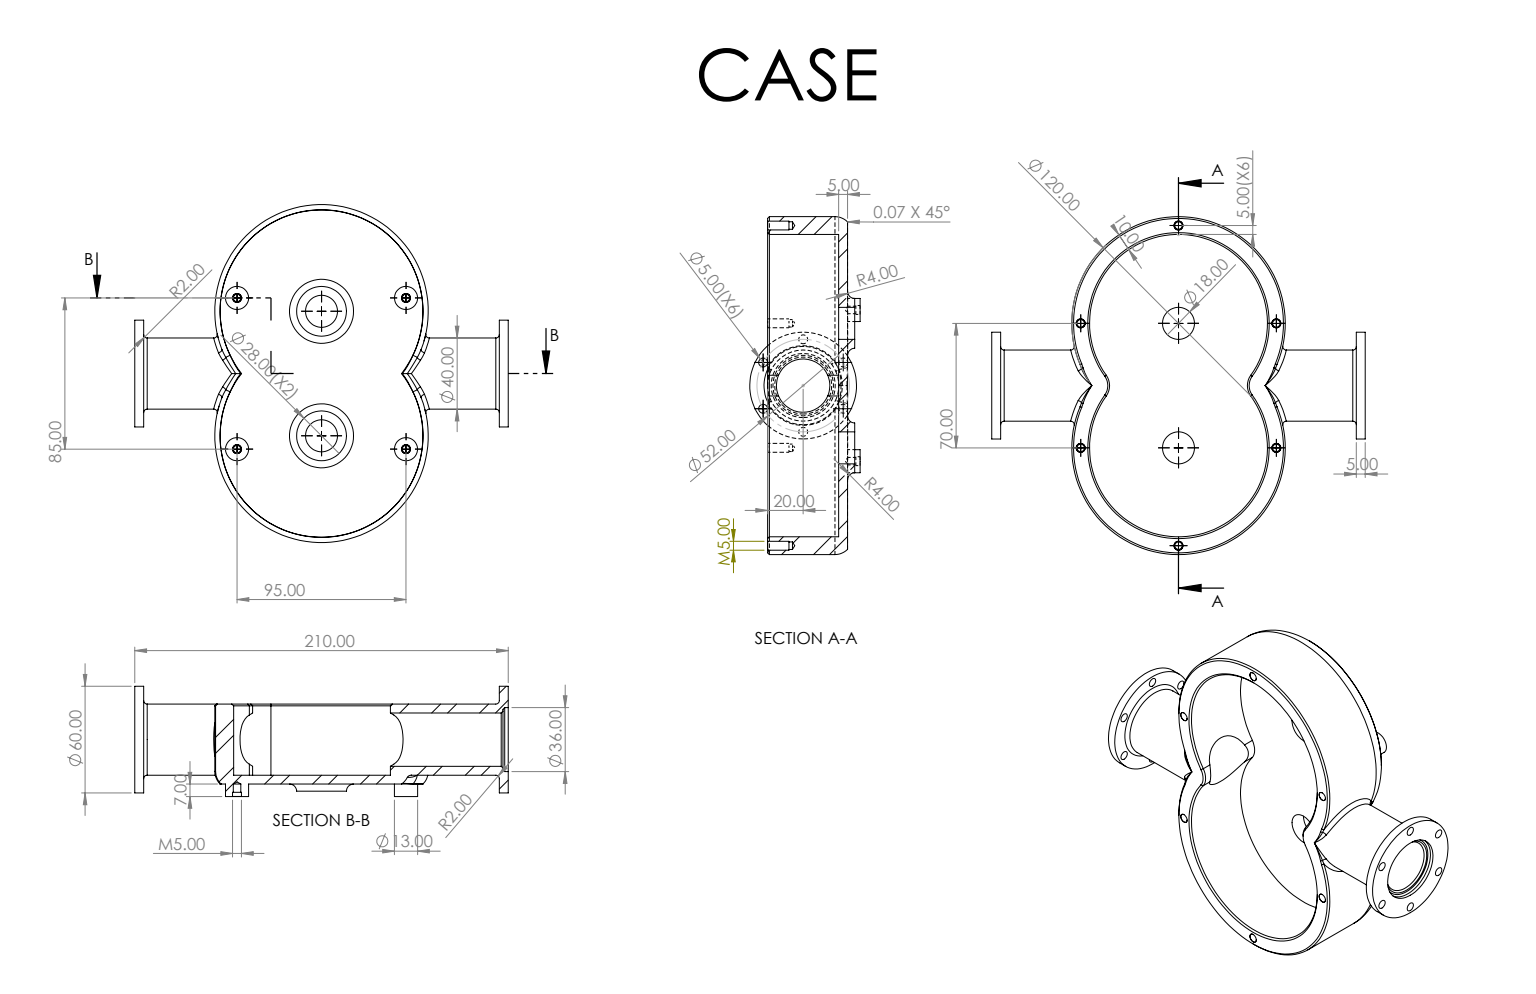
ISO-10303-21;
HEADER;
FILE_DESCRIPTION (('STEP AP214'),
    '1' );
FILE_NAME ('CASE.step',
    '2026-10-24T00:51:42',
    ( '' ),
    ( '' ),
    'SwSTEP 2.0',
    'SolidWorks 2025',
    '' );
FILE_SCHEMA (( 'AUTOMOTIVE_DESIGN' ));
ENDSEC;

DATA;
#6=VECTOR ( 'NONE', #825, 1000.000000000000000 ) ;
#8=LINE ( 'NONE', #12148, #20561 ) ;
#9=CARTESIAN_POINT ( 'NONE',  ( 7.505578006075174891, 1.461761173328240959, -55.63523492904085543 ) ) ;
#15=CARTESIAN_POINT ( 'NONE',  ( -11.08851315719095609, 40.00000000000000000, -54.00022650832062254 ) ) ;
#16=VERTEX_POINT ( 'NONE', #2397 ) ;
#17=DIRECTION ( 'NONE',  ( 0.000000000000000000, -1.000000000000000000, 0.000000000000000000 ) ) ;
#18=CARTESIAN_POINT ( 'NONE',  ( 17.25453130113929134, 34.47978402352274685, -57.33123263757907750 ) ) ;
#21=CARTESIAN_POINT ( 'NONE',  ( 7.552830766296163567, 40.00000000000000000, 52.78252194617787296 ) ) ;
#22=CARTESIAN_POINT ( 'NONE',  ( 14.52224280010135615, 23.83254695043585869, -45.61498238574513664 ) ) ;
#25=CARTESIAN_POINT ( 'NONE',  ( -14.27302218980893578, 2.669631712211265828, 56.31136122552221934 ) ) ;
#26=ADVANCED_FACE ( 'NONE', ( #12912 ), #4119, .F. ) ;
#30=DIRECTION ( 'NONE',  ( -0.000000000000000000, -1.000000000000000000, -0.000000000000000000 ) ) ;
#32=AXIS2_PLACEMENT_3D ( 'NONE', #9463, #19547, #3850 ) ;
#33=ORIENTED_EDGE ( 'NONE', *, *, #2893, .T. ) ;
#37=CARTESIAN_POINT ( 'NONE',  ( 17.68664055422810932, 6.162676607241195370, 57.44855069909474565 ) ) ;
#38=CARTESIAN_POINT ( 'NONE',  ( 9.260192184203184240, 40.00000000000000000, 53.42688922108487759 ) ) ;
#39=EDGE_CURVE ( 'NONE', #4801, #16804, #900, .T. ) ;
#42=CARTESIAN_POINT ( 'NONE',  ( -0.5350771668691333138, 5.000000000000000888, 38.73397172404479960 ) ) ;
#44=CARTESIAN_POINT ( 'NONE',  ( 4.012214033923966740E-15, -1.570715777137759117, 48.07784006879590066 ) ) ;
#46=CARTESIAN_POINT ( 'NONE',  ( -20.00000000000001421, 20.00000000000000000, -60.62177826491068799 ) ) ;
#47=EDGE_LOOP ( 'NONE', ( #21691, #2135, #22378, #2493 ) ) ;
#50=CARTESIAN_POINT ( 'NONE',  ( 35.00000000000000000, -5.000000000000000888, -18.00000000000000000 ) ) ;
#52=CARTESIAN_POINT ( 'NONE',  ( 19.96400288702118431, 18.50890182901837022, 60.61328093326561373 ) ) ;
#54=CARTESIAN_POINT ( 'NONE',  ( -5.833333333333327708, 6.180730040185831164, 40.61164310337068173 ) ) ;
#56=AXIS2_PLACEMENT_3D ( 'NONE', #2091, #11020, #12611 ) ;
#58=ORIENTED_EDGE ( 'NONE', *, *, #10603, .F. ) ;
#59=ORIENTED_EDGE ( 'NONE', *, *, #871, .T. ) ;
#60=DIRECTION ( 'NONE',  ( -0.000000000000000000, -0.000000000000000000, 1.000000000000000000 ) ) ;
#62=ADVANCED_FACE ( 'NONE', ( #18545 ), #20663, .F. ) ;
#63=DIRECTION ( 'NONE',  ( -0.000000000000000000, -1.000000000000000000, -0.000000000000000000 ) ) ;
#65=CARTESIAN_POINT ( 'NONE',  ( 2.244030701350347989, 39.96966515414118959, 50.39883264010746444 ) ) ;
#67=DIRECTION ( 'NONE',  ( -0.000000000000000000, 1.000000000000000000, -0.000000000000000000 ) ) ;
#70=CARTESIAN_POINT ( 'NONE',  ( -34.99999999999999289, 40.00000000000000000, 60.00000000000001421 ) ) ;
#71=ADVANCED_FACE ( 'NONE', ( #20271 ), #22509, .T. ) ;
#76=CARTESIAN_POINT ( 'NONE',  ( -8.123117863918686510, 39.63127865102772063, 53.85467328977310331 ) ) ;
#77=DIRECTION ( 'NONE',  ( 0.000000000000000000, 0.000000000000000000, -1.000000000000000000 ) ) ;
#82=ORIENTED_EDGE ( 'NONE', *, *, #17683, .T. ) ;
#88=DIRECTION ( 'NONE',  ( 0.000000000000000000, 0.000000000000000000, -1.000000000000000000 ) ) ;
#89=DIRECTION ( 'NONE',  ( -0.000000000000000000, 1.000000000000000000, -0.000000000000000000 ) ) ;
#90=CARTESIAN_POINT ( 'NONE',  ( -11.54473802384001324, 36.35512261685148871, -55.24115706042312013 ) ) ;
#91=CARTESIAN_POINT ( 'NONE',  ( -14.50678847729824383, 23.83439465050324912, -45.60743157421818950 ) ) ;
#95=DIRECTION ( 'NONE',  ( 0.7071067811865561215, 8.659560562355038861E-17, -0.7071067811865390240 ) ) ;
#105=VERTEX_POINT ( 'NONE', #9938 ) ;
#108=CYLINDRICAL_SURFACE ( 'NONE', #5479, 2.500000000000002220 ) ;
#110=CARTESIAN_POINT ( 'NONE',  ( 90.00000000000000000, 40.00000000000000000, -2.099999999999991651 ) ) ;
#112=ORIENTED_EDGE ( 'NONE', *, *, #18556, .F. ) ;
#114=CARTESIAN_POINT ( 'NONE',  ( -11.49398617737440986, 39.99999999999999289, 54.13866599136459001 ) ) ;
#117=CIRCLE ( 'NONE', #11814, 20.00000000000000000 ) ;
#118=CARTESIAN_POINT ( 'NONE',  ( 14.34650594848453942, 37.25275621493270961, -56.33443587181653811 ) ) ;
#120=CARTESIAN_POINT ( 'NONE',  ( 14.04383866228953259, 25.28361825225917769, -45.39674436955350245 ) ) ;
#121=VERTEX_POINT ( 'NONE', #15312 ) ;
#123=CARTESIAN_POINT ( 'NONE',  ( -1.321840103127373878, 39.98984252836526565, -49.73540240164955151 ) ) ;
#124=ORIENTED_EDGE ( 'NONE', *, *, #15859, .T. ) ;
#125=DIRECTION ( 'NONE',  ( -0.000000000000000000, -0.000000000000000000, 1.000000000000000000 ) ) ;
#126=VECTOR ( 'NONE', #7524, 1000.000000000000000 ) ;
#130=AXIS2_PLACEMENT_3D ( 'NONE', #19374, #14408, #3677 ) ;
#133=ORIENTED_EDGE ( 'NONE', *, *, #15085, .T. ) ;
#134=ADVANCED_FACE ( 'NONE', ( #4576 ), #8565, .F. ) ;
#136=DIRECTION ( 'NONE',  ( 0.000000000000000000, 0.000000000000000000, -1.000000000000000000 ) ) ;
#139=CARTESIAN_POINT ( 'NONE',  ( 2.175117723777981293, 39.99999999999999289, 50.07592572012215015 ) ) ;
#140=ORIENTED_EDGE ( 'NONE', *, *, #13576, .T. ) ;
#141=FACE_BOUND ( 'NONE', #13024, .T. ) ;
#142=DIRECTION ( 'NONE',  ( 0.000000000000000000, -0.000000000000000000, -1.000000000000000000 ) ) ;
#145=EDGE_CURVE ( 'NONE', #18194, #11720, #10158, .T. ) ;
#149=CARTESIAN_POINT ( 'NONE',  ( -3.591923118226331086E-15, -4.883049072964007919, -45.13706194851761921 ) ) ;
#150=ORIENTED_EDGE ( 'NONE', *, *, #14053, .T. ) ;
#151=CARTESIAN_POINT ( 'NONE',  ( 8.331955809010642255, 38.18181818181816567, 56.36098470834075158 ) ) ;
#152=DIRECTION ( 'NONE',  ( 1.000000000000000000, 0.000000000000000000, 0.000000000000000000 ) ) ;
#153=CARTESIAN_POINT ( 'NONE',  ( -4.436826463219276206, 39.87775421764654027, 51.86208637039475633 ) ) ;
#154=VECTOR ( 'NONE', #7572, 1000.000000000000114 ) ;
#155=CARTESIAN_POINT ( 'NONE',  ( 16.16619463698827630, 31.79081685853978101, 57.00191113791574082 ) ) ;
#158=CONICAL_SURFACE ( 'NONE', #22127, 2.524999999999999467, 0.7853981633973095011 ) ;
#160=AXIS2_PLACEMENT_3D ( 'NONE', #15195, #16931, #6621 ) ;
#164=VERTEX_POINT ( 'NONE', #8227 ) ;
#168=CARTESIAN_POINT ( 'NONE',  ( 0.9607529184257457278, 39.99453553102809877, 49.46704527242837912 ) ) ;
#170=B_SPLINE_CURVE_WITH_KNOTS ( 'NONE', 3,
 ( #22387, #25, #8397, #19283, #7015, #1634, #10434, #3588, #15593, #13972, #6677, #20996, #3128, #5083, #5301, #10546, #17549, #22616, #11941, #17094, #20771, #22497, #10215, #13635, #20652, #12275, #4959, #1859, #17430, #22274, #15253, #20548, #10099, #6572, #8504, #13532, #4852, #11822, #6912, #12059 ),
 .UNSPECIFIED., .F., .F.,
 ( 4, 2, 2, 2, 2, 2, 2, 2, 2, 2, 2, 2, 2, 2, 2, 2, 2, 2, 2, 4 ),
 ( 0.000000000000000000, 0.002766773850155583667, 0.004150160775233378320, 0.005533547700311173406, 0.008300321550466751436, 0.009683708475544540450, 0.01106709540062232947, 0.01660064310093350981, 0.01798403002601129883, 0.01936741695108909131, 0.02213419080124466934, 0.02490096465140025084, 0.02766773850155583581, 0.03043451235171141731, 0.03181789927678920632, 0.03320128620186699187, 0.03873483390217814792, 0.04011822082725592653, 0.04150160775233370514, 0.04426838160248924847 ),
 .UNSPECIFIED. ) ;
#171=EDGE_CURVE ( 'NONE', #14638, #20199, #4931, .T. ) ;
#172=ORIENTED_EDGE ( 'NONE', *, *, #12979, .T. ) ;
#174=CARTESIAN_POINT ( 'NONE',  ( 13.56354382738798847, 2.142135623730931471, -56.03997097393683191 ) ) ;
#176=DIRECTION ( 'NONE',  ( -0.5840452403773153112, 0.8117211080122311850, 0.000000000000000000 ) ) ;
#178=CARTESIAN_POINT ( 'NONE',  ( 11.86180952233169705, 39.00000000000000000, 55.35904751184887118 ) ) ;
#186=EDGE_LOOP ( 'NONE', ( #20186, #1645, #6973, #5901 ) ) ;
#187=AXIS2_PLACEMENT_3D ( 'NONE', #2297, #17991, #16268 ) ;
#191=B_SPLINE_CURVE_WITH_KNOTS ( 'NONE', 3,
 ( #12236, #6868, #6982, #6529, #11779, #5041, #16942, #13938, #20733, #8239, #18781, #17166, #17055, #13836, #5157, #1362 ),
 .UNSPECIFIED., .F., .F.,
 ( 4, 2, 2, 2, 2, 2, 2, 4 ),
 ( 8.673617379884035472E-19, 0.003169695113379691204, 0.006339390226759381540, 0.007924237783449226274, 0.008716661561794153412, 0.009509085340139077080, 0.01109393289682892789, 0.01267878045351877869 ),
 .UNSPECIFIED. ) ;
#193=CARTESIAN_POINT ( 'NONE',  ( 9.367793990832831597, -4.928932186891253231, -51.00106331756588673 ) ) ;
#194=CARTESIAN_POINT ( 'NONE',  ( 11.45074849662552197, 39.99999999999999289, -54.12667998692793958 ) ) ;
#199=VECTOR ( 'NONE', #3023, 1000.000000000000000 ) ;
#200=CARTESIAN_POINT ( 'NONE',  ( -15.91103418227302058, 35.86133518681679533, -56.88632568426858427 ) ) ;
#201=AXIS2_PLACEMENT_3D ( 'NONE', #4772, #15280, #6939 ) ;
#208=ADVANCED_FACE ( 'NONE', ( #17833 ), #17377, .F. ) ;
#213=EDGE_CURVE ( 'NONE', #13383, #4605, #12223, .T. ) ;
#216=VECTOR ( 'NONE', #1494, 1000.000000000000114 ) ;
#219=ORIENTED_EDGE ( 'NONE', *, *, #7330, .T. ) ;
#221=AXIS2_PLACEMENT_3D ( 'NONE', #15560, #3559, #10737 ) ;
#223=ADVANCED_FACE ( 'NONE', ( #21279 ), #5571, .F. ) ;
#226=CARTESIAN_POINT ( 'NONE',  ( -1.387778780781445676E-14, 20.00000000000000000, -105.0020000000000095 ) ) ;
#231=CARTESIAN_POINT ( 'NONE',  ( -9.062586715439731933, 2.130694986425758941, -54.31128890270724696 ) ) ;
#232=ORIENTED_EDGE ( 'NONE', *, *, #1295, .T. ) ;
#234=CARTESIAN_POINT ( 'NONE',  ( 17.14099744770036082, 5.493236686326223861, -57.28126710884282602 ) ) ;
#239=FACE_OUTER_BOUND ( 'NONE', #8251, .T. ) ;
#240=CARTESIAN_POINT ( 'NONE',  ( -7.031141255823502689, 39.67715640622406426, -53.36152254753006474 ) ) ;
#241=AXIS2_PLACEMENT_3D ( 'NONE', #20174, #2191, #19945 ) ;
#244=CARTESIAN_POINT ( 'NONE',  ( -2.496587642955530040, 0.1153990516131219446, 52.32802461649446002 ) ) ;
#245=VECTOR ( 'NONE', #16073, 1000.000000000000000 ) ;
#249=VERTEX_POINT ( 'NONE', #19225 ) ;
#253=LINE ( 'NONE', #3817, #4827 ) ;
#254=DIRECTION ( 'NONE',  ( -0.000000000000000000, -0.000000000000000000, -1.000000000000000000 ) ) ;
#256=CARTESIAN_POINT ( 'NONE',  ( 7.563456360162507330, 39.99999999999999289, 52.78701495172266078 ) ) ;
#259=FACE_BOUND ( 'NONE', #21033, .T. ) ;
#262=CARTESIAN_POINT ( 'NONE',  ( 7.325260514639500961E-15, -4.648749848371387827, 45.43309249825157536 ) ) ;
#264=EDGE_LOOP ( 'NONE', ( #1620, #15292, #18249, #3062 ) ) ;
#268=CARTESIAN_POINT ( 'NONE',  ( -34.99999999999980815, 40.00000000000000711, 52.47499999999922693 ) ) ;
#269=CARTESIAN_POINT ( 'NONE',  ( -0.3104238174410937634, 39.99820335227858692, 49.10409449009599570 ) ) ;
#270=CARTESIAN_POINT ( 'NONE',  ( -35.00000000000000000, 40.00000000000000000, 1.387778780781445676E-14 ) ) ;
#274=CARTESIAN_POINT ( 'NONE',  ( 21.98712579307491666, 15.48449832074051358, 58.57208548029188222 ) ) ;
#276=AXIS2_PLACEMENT_3D ( 'NONE', #12018, #17271, #16939 ) ;
#282=AXIS2_PLACEMENT_3D ( 'NONE', #21094, #12372, #5501 ) ;
#283=ORIENTED_EDGE ( 'NONE', *, *, #5855, .F. ) ;
#284=EDGE_LOOP ( 'NONE', ( #20837, #17843 ) ) ;
#285=CARTESIAN_POINT ( 'NONE',  ( -9.689843208404443686, 39.33333333333332860, 54.54983754392751649 ) ) ;
#289=VECTOR ( 'NONE', #14140, 1000.000000000000000 ) ;
#291=B_SPLINE_CURVE_WITH_KNOTS ( 'NONE', 3,
 ( #8113, #6044, #21633, #5929, #14842, #9709 ),
 .UNSPECIFIED., .F., .F.,
 ( 4, 2, 4 ),
 ( 1.788112030672749005E-18, 0.002694896630591163932, 0.005389793261182326128 ),
 .UNSPECIFIED. ) ;
#293=CARTESIAN_POINT ( 'NONE',  ( 3.944370656192286440, 39.90454853199823759, 51.54919367184183443 ) ) ;
#296=DIRECTION ( 'NONE',  ( 0.000000000000000000, 0.000000000000000000, -1.000000000000000000 ) ) ;
#297=CARTESIAN_POINT ( 'NONE',  ( -42.50000000000000711, -12.00000000000000000, -47.50000000000000000 ) ) ;
#307=DIRECTION ( 'NONE',  ( 1.000000000000000000, 0.000000000000000000, 0.000000000000000000 ) ) ;
#310=ORIENTED_EDGE ( 'NONE', *, *, #5485, .T. ) ;
#311=ADVANCED_FACE ( 'NONE', ( #9013 ), #19696, .F. ) ;
#313=ORIENTED_EDGE ( 'NONE', *, *, #10353, .F. ) ;
#317=FACE_OUTER_BOUND ( 'NONE', #17252, .T. ) ;
#319=DIRECTION ( 'NONE',  ( -0.000000000000000000, 1.000000000000000000, -0.000000000000000000 ) ) ;
#322=CARTESIAN_POINT ( 'NONE',  ( -20.00000000000001421, 19.20373330966867798, 60.62177826491072352 ) ) ;
#325=CARTESIAN_POINT ( 'NONE',  ( -15.00000000000001421, 20.00000000000000000, -45.82575694955838230 ) ) ;
#329=CARTESIAN_POINT ( 'NONE',  ( -1.387778780781445676E-14, 20.00000000000000000, 98.00000000000000000 ) ) ;
#330=DIRECTION ( 'NONE',  ( 0.000000000000000000, 0.000000000000000000, -1.000000000000000000 ) ) ;
#334=FACE_OUTER_BOUND ( 'NONE', #3737, .T. ) ;
#337=DIRECTION ( 'NONE',  ( 0.000000000000000000, -1.000000000000000000, 0.000000000000000000 ) ) ;
#339=( BOUNDED_SURFACE ( )  B_SPLINE_SURFACE ( 3, 2, ( 
 ( #20618, #22011, #20293 ),
 ( #20513, #13386, #1148 ),
 ( #11788, #8141, #20176 ),
 ( #4597, #4928, #11578 ),
 ( #1371, #10065, #17063 ),
 ( #3217, #18567, #8367 ) ),
 .UNSPECIFIED., .F., .F., .F. ) 
 B_SPLINE_SURFACE_WITH_KNOTS ( ( 4, 2, 4 ),
 ( 3, 3 ),
 ( 0.000000000000000000, 0.002858401832365834675, 0.005716803664731669350 ),
 ( 0.000000000000000000, 1.000000000000000000 ),
 .UNSPECIFIED. ) 
 GEOMETRIC_REPRESENTATION_ITEM ( )  RATIONAL_B_SPLINE_SURFACE ( (
 ( 1.000000000000000000, 0.7200096751079140267, 1.000000000000000000),
 ( 1.000000000000000000, 0.7065285139735018038, 1.000000000000000000),
 ( 1.000000000000000000, 0.6920701671002518207, 1.000000000000000000),
 ( 1.000000000000000000, 0.6615687397045608709, 1.000000000000000000),
 ( 1.000000000000000000, 0.6455195629511447653, 1.000000000000000000),
 ( 1.000000000000000000, 0.6290213284793418902, 1.000000000000000000) ) ) 
 REPRESENTATION_ITEM ( '' )  SURFACE ( )  );
#340=ORIENTED_EDGE ( 'NONE', *, *, #16660, .T. ) ;
#341=CARTESIAN_POINT ( 'NONE',  ( 0.2660997432313502165, 39.99958209296121225, -48.93999222993210196 ) ) ;
#343=CARTESIAN_POINT ( 'NONE',  ( -11.68090480754633553, 3.765577839755389622, 57.90797000640144176 ) ) ;
#348=CARTESIAN_POINT ( 'NONE',  ( -6.444993702122386203, 40.00000000000000711, 52.30045897829974422 ) ) ;
#350=DIRECTION ( 'NONE',  ( 0.000000000000000000, 0.000000000000000000, -1.000000000000000000 ) ) ;
#351=CARTESIAN_POINT ( 'NONE',  ( 18.51338123223699483, 7.266791589766445014, -57.69263490290608587 ) ) ;
#355=DIRECTION ( 'NONE',  ( -0.000000000000000000, 1.000000000000000000, -0.000000000000000000 ) ) ;
#356=EDGE_CURVE ( 'NONE', #18097, #20626, #19791, .T. ) ;
#357=EDGE_CURVE ( 'NONE', #922, #13123, #3450, .T. ) ;
#358=CARTESIAN_POINT ( 'NONE',  ( -0.4769535673226554806, 39.99865963977220673, -49.10163031951724122 ) ) ;
#364=EDGE_CURVE ( 'NONE', #16, #13103, #12663, .T. ) ;
#367=EDGE_LOOP ( 'NONE', ( #19878, #14451, #14553, #14113 ) ) ;
#369=B_SPLINE_CURVE_WITH_KNOTS ( 'NONE', 3,
 ( #18817, #9981, #13409, #16973, #17087, #15470 ),
 .UNSPECIFIED., .F., .F.,
 ( 4, 2, 4 ),
 ( 1.978164943978792966E-18, 0.005389490931282729137, 0.01077898186256545654 ),
 .UNSPECIFIED. ) ;
#370=ORIENTED_EDGE ( 'NONE', *, *, #8346, .T. ) ;
#371=CARTESIAN_POINT ( 'NONE',  ( -34.99999999999980815, 39.97500000000000142, 52.49999999999922551 ) ) ;
#373=DIRECTION ( 'NONE',  ( -0.000000000000000000, 1.000000000000000000, -0.000000000000000000 ) ) ;
#374=CARTESIAN_POINT ( 'NONE',  ( 0.3946982817249323205, 39.99999999999999289, 48.99018268902280226 ) ) ;
#380=CARTESIAN_POINT ( 'NONE',  ( -21.21578383525638145, 27.34973130705545685, -58.39578210113618439 ) ) ;
#383=CARTESIAN_POINT ( 'NONE',  ( 0.3709469612214016387, -0.009390992346610399152, 50.78654667931946420 ) ) ;
#385=CARTESIAN_POINT ( 'NONE',  ( 3.981168190751217750, 39.90684668434315086, -51.58237481356633225 ) ) ;
#386=CARTESIAN_POINT ( 'NONE',  ( -3.210361346424068341, 39.75306810546534564, 52.30715206667691319 ) ) ;
#387=CARTESIAN_POINT ( 'NONE',  ( 5.007713804312083461, 0.5950132857128228592, 54.03314628406707243 ) ) ;
#388=ORIENTED_EDGE ( 'NONE', *, *, #9153, .F. ) ;
#389=CARTESIAN_POINT ( 'NONE',  ( 21.77460018174823020, 14.53841458819210786, 58.52494103856225394 ) ) ;
#390=DIRECTION ( 'NONE',  ( -0.000000000000000000, 1.000000000000000000, -0.000000000000000000 ) ) ;
#391=ADVANCED_FACE ( 'NONE', ( #12888 ), #6369, .F. ) ;
#392=AXIS2_PLACEMENT_3D ( 'NONE', #21456, #373, #16290 ) ;
#393=ADVANCED_FACE ( 'NONE', ( #19897 ), #22473, .F. ) ;
#394=FACE_BOUND ( 'NONE', #4049, .T. ) ;
#400=DIRECTION ( 'NONE',  ( 0.000000000000000000, 0.000000000000000000, -1.000000000000000000 ) ) ;
#403=ORIENTED_EDGE ( 'NONE', *, *, #16215, .T. ) ;
#404=CARTESIAN_POINT ( 'NONE',  ( 8.215393105052410050, 1.749144060401382594, 56.08634520685871649 ) ) ;
#408=CARTESIAN_POINT ( 'NONE',  ( 90.00000000000000000, 40.00000000000000000, -9.108981535246192915E-16 ) ) ;
#409=PRODUCT_DEFINITION_CONTEXT ( 'detailed design', #19716, 'design' ) ;
#412=LINE ( 'NONE', #12881, #16434 ) ;
#413=DIRECTION ( 'NONE',  ( -0.000000000000000000, 1.000000000000000000, -0.000000000000000000 ) ) ;
#418=ORIENTED_EDGE ( 'NONE', *, *, #9253, .T. ) ;
#420=ORIENTED_EDGE ( 'NONE', *, *, #17534, .T. ) ;
#423=EDGE_CURVE ( 'NONE', #6835, #14085, #18431, .T. ) ;
#425=CARTESIAN_POINT ( 'NONE',  ( -15.99999999999994493, 20.00000000000000355, 102.0000000000000142 ) ) ;
#431=EDGE_CURVE ( 'NONE', #18746, #22096, #8909, .T. ) ;
#433=CARTESIAN_POINT ( 'NONE',  ( -1.387778780781445518E-14, 20.00000000000000355, 105.0000000000000142 ) ) ;
#434=CARTESIAN_POINT ( 'NONE',  ( -4.240553750831113966, 39.54840718952534218, -53.29860200223215827 ) ) ;
#436=CARTESIAN_POINT ( 'NONE',  ( 42.50000000000000711, -12.00000000000012434, 47.50000000000000711 ) ) ;
#437=EDGE_LOOP ( 'NONE', ( #19321, #11587 ) ) ;
#438=B_SPLINE_CURVE_WITH_KNOTS ( 'NONE', 3,
 ( #10429, #22613, #10094, #4956, #5079, #11935, #22, #18935, #120, #7012, #15588, #17091, #13969, #17204, #1404, #1517, #19051, #3358, #20993, #10316, #17312, #5297, #12272, #19735 ),
 .UNSPECIFIED., .F., .F.,
 ( 4, 2, 2, 2, 2, 2, 2, 2, 2, 2, 2, 4 ),
 ( 0.02614117015034099489, 0.02729036340605310237, 0.02843955666176521332, 0.03073794317318943869, 0.03188713642890154965, 0.03303632968461366060, 0.03533471619603787556, 0.03648390945174998651, 0.03763310270746209746, 0.03993148921888632630, 0.04222987573031054820, 0.04452826224173477704 ),
 .UNSPECIFIED. ) ;
#440=DIRECTION ( 'NONE',  ( 0.000000000000000000, 1.000000000000000000, 0.000000000000000000 ) ) ;
#441=DIRECTION ( 'NONE',  ( 0.000000000000000000, 0.000000000000000000, -1.000000000000000000 ) ) ;
#442=AXIS2_PLACEMENT_3D ( 'NONE', #3968, #12531, #11161 ) ;
#449=CARTESIAN_POINT ( 'NONE',  ( -42.50000000000000711, -9.600000000000001421, -47.50000000000000000 ) ) ;
#451=ORIENTED_EDGE ( 'NONE', *, *, #20783, .T. ) ;
#453=CARTESIAN_POINT ( 'NONE',  ( -9.689843208404424146, 39.33333333333333570, 54.54983754392744544 ) ) ;
#454=VERTEX_POINT ( 'NONE', #9919 ) ;
#464=CARTESIAN_POINT ( 'NONE',  ( -0.8008185833748354687, 39.99628548823710616, -49.34729503705691656 ) ) ;
#465=EDGE_LOOP ( 'NONE', ( #20901, #7728 ) ) ;
#466=FACE_OUTER_BOUND ( 'NONE', #16645, .T. ) ;
#469=EDGE_CURVE ( 'NONE', #19954, #548, #5572, .T. ) ;
#471=VECTOR ( 'NONE', #14248, 1000.000000000000000 ) ;
#477=CIRCLE ( 'NONE', #13626, 2.099999999999997868 ) ;
#478=VERTEX_POINT ( 'NONE', #4882 ) ;
#479=CYLINDRICAL_SURFACE ( 'NONE', #15776, 2.099999999999997868 ) ;
#485=ORIENTED_EDGE ( 'NONE', *, *, #11304, .F. ) ;
#486=CARTESIAN_POINT ( 'NONE',  ( -3.709350152758254637, -1.139907008998718663, 50.71254743501651063 ) ) ;
#487=DIRECTION ( 'NONE',  ( 0.000000000000000000, 1.000000000000000000, 0.000000000000000000 ) ) ;
#488=LINE ( 'NONE', #7485, #991 ) ;
#490=CARTESIAN_POINT ( 'NONE',  ( 2.951378045146772156, -1.204966337759544759, 50.23352299313199154 ) ) ;
#495=ORIENTED_EDGE ( 'NONE', *, *, #11690, .T. ) ;
#496=CARTESIAN_POINT ( 'NONE',  ( 9.433064893952842311, 39.99999999999999289, -53.48670810797406006 ) ) ;
#497=AXIS2_PLACEMENT_3D ( 'NONE', #8009, #16823, #14964 ) ;
#498=CARTESIAN_POINT ( 'NONE',  ( 20.00279574339558053, 20.27588806490328466, 58.14815718762942254 ) ) ;
#499=CARTESIAN_POINT ( 'NONE',  ( -15.49999999999980282, -2.516660498395516310, -105.0000000000000142 ) ) ;
#500=CIRCLE ( 'NONE', #12915, 49.99999999999998579 ) ;
#503=DIRECTION ( 'NONE',  ( 0.000000000000000000, 0.000000000000000000, -1.000000000000000000 ) ) ;
#504=EDGE_CURVE ( 'NONE', #4461, #15820, #3176, .T. ) ;
#506=CIRCLE ( 'NONE', #7080, 2.500000000000002220 ) ;
#507=VERTEX_POINT ( 'NONE', #8099 ) ;
#511=DIRECTION ( 'NONE',  ( 0.000000000000000000, 0.000000000000000000, 1.000000000000000000 ) ) ;
#513=DIRECTION ( 'NONE',  ( 0.000000000000000000, 0.000000000000000000, -1.000000000000000000 ) ) ;
#515=ORIENTED_EDGE ( 'NONE', *, *, #6519, .F. ) ;
#521=EDGE_LOOP ( 'NONE', ( #7198, #21229, #17440, #9818 ) ) ;
#523=CARTESIAN_POINT ( 'NONE',  ( -42.50000000000000711, -5.000000000000000000, -45.40000000000000568 ) ) ;
#524=FACE_OUTER_BOUND ( 'NONE', #18019, .T. ) ;
#529=CARTESIAN_POINT ( 'NONE',  ( 42.50000000000000711, -12.00000000000000000, 47.50000000000000711 ) ) ;
#530=DIRECTION ( 'NONE',  ( 0.000000000000000000, -0.000000000000000000, -1.000000000000000000 ) ) ;
#532=CYLINDRICAL_SURFACE ( 'NONE', #9399, 30.00000000000000000 ) ;
#535=EDGE_LOOP ( 'NONE', ( #8078, #13018, #9083, #19228 ) ) ;
#536=ORIENTED_EDGE ( 'NONE', *, *, #10840, .T. ) ;
#539=CARTESIAN_POINT ( 'NONE',  ( -1.247165098465854882, 0.02902681952929966891, -51.42818515578048277 ) ) ;
#540=EDGE_CURVE ( 'NONE', #20205, #18632, #21256, .T. ) ;
#543=DIRECTION ( 'NONE',  ( 0.000000000000000000, 0.000000000000000000, 1.000000000000000000 ) ) ;
#545=CARTESIAN_POINT ( 'NONE',  ( -10.79594548525845354, 39.62239930148190581, -54.90840750699925366 ) ) ;
#546=FACE_OUTER_BOUND ( 'NONE', #6799, .T. ) ;
#547=DIRECTION ( 'NONE',  ( -0.000000000000000000, 1.000000000000000000, -0.000000000000000000 ) ) ;
#548=VERTEX_POINT ( 'NONE', #54 ) ;
#550=FACE_OUTER_BOUND ( 'NONE', #1337, .T. ) ;
#551=CARTESIAN_POINT ( 'NONE',  ( -1.387778780781445676E-14, 40.00000000000000000, -48.73397172404481381 ) ) ;
#554=CARTESIAN_POINT ( 'NONE',  ( 7.033428926742989695, 6.687309450572964664, -41.47353357286041842 ) ) ;
#555=ORIENTED_EDGE ( 'NONE', *, *, #20018, .F. ) ;
#558=ORIENTED_EDGE ( 'NONE', *, *, #1941, .T. ) ;
#560=CARTESIAN_POINT ( 'NONE',  ( -1.387778780781445676E-14, 20.00000000000000000, -100.0000000000000000 ) ) ;
#563=ORIENTED_EDGE ( 'NONE', *, *, #5695, .F. ) ;
#564=CARTESIAN_POINT ( 'NONE',  ( 14.99999999999998579, 20.00000000000000355, 60.00200000000000244 ) ) ;
#566=DIRECTION ( 'NONE',  ( 0.000000000000000000, 0.000000000000000000, -1.000000000000000000 ) ) ;
#572=DIRECTION ( 'NONE',  ( 0.000000000000000000, 0.000000000000000000, -1.000000000000000000 ) ) ;
#575=VERTEX_POINT ( 'NONE', #17585 ) ;
#576=DIRECTION ( 'NONE',  ( -0.000000000000000000, 1.000000000000000000, -0.000000000000000000 ) ) ;
#578=DIRECTION ( 'NONE',  ( 0.000000000000000000, 0.000000000000000000, 1.000000000000000000 ) ) ;
#579=CARTESIAN_POINT ( 'NONE',  ( -9.064496942927510403, 40.00000000000000711, 53.36141823319849919 ) ) ;
#582=EDGE_LOOP ( 'NONE', ( #20787, #19014, #14328, #6935, #11159 ) ) ;
#585=CARTESIAN_POINT ( 'NONE',  ( -0.6551157041172263051, 39.99751803486232404, -49.23722055247538520 ) ) ;
#588=CARTESIAN_POINT ( 'NONE',  ( -6.261274683082161729, 0.9579800028911584775, 54.84444022978226485 ) ) ;
#590=EDGE_CURVE ( 'NONE', #6177, #19116, #506, .T. ) ;
#592=AXIS2_PLACEMENT_3D ( 'NONE', #3774, #3673, #10624 ) ;
#593=ORIENTED_EDGE ( 'NONE', *, *, #20919, .F. ) ;
#596=EDGE_LOOP ( 'NONE', ( #6630, #2604, #22575, #5586 ) ) ;
#597=ORIENTED_EDGE ( 'NONE', *, *, #20910, .T. ) ;
#599=VERTEX_POINT ( 'NONE', #15846 ) ;
#604=CARTESIAN_POINT ( 'NONE',  ( -26.00000000000001421, 19.99999999999982947, 105.0000000000000142 ) ) ;
#605=CARTESIAN_POINT ( 'NONE',  ( -26.00000000000001421, 19.99999999999982947, -105.0000000000000142 ) ) ;
#606=ORIENTED_EDGE ( 'NONE', *, *, #5866, .F. ) ;
#607=DIRECTION ( 'NONE',  ( 0.000000000000000000, 0.000000000000000000, 1.000000000000000000 ) ) ;
#609=CARTESIAN_POINT ( 'NONE',  ( -42.50000000000000711, -12.00000000000000000, 45.40000000000001279 ) ) ;
#613=CARTESIAN_POINT ( 'NONE',  ( 5.511499161255899004, 0.6970817516857953366, 52.42185088604356480 ) ) ;
#615=CARTESIAN_POINT ( 'NONE',  ( 6.450208405384564081, 39.75599223657528825, 53.02618523645297444 ) ) ;
#617=AXIS2_PLACEMENT_3D ( 'NONE', #4326, #16459, #11301 ) ;
#619=CARTESIAN_POINT ( 'NONE',  ( -1.387778780781445676E-14, 20.00000000000000000, 100.0000000000000000 ) ) ;
#620=CARTESIAN_POINT ( 'NONE',  ( -23.50000000000001066, 19.99999999999982947, 100.0000000000000000 ) ) ;
#623=DIRECTION ( 'NONE',  ( 0.000000000000000000, 0.000000000000000000, -1.000000000000000000 ) ) ;
#629=CARTESIAN_POINT ( 'NONE',  ( -90.00000000000000000, 40.00000000000000000, 2.500000000000001332 ) ) ;
#634=CARTESIAN_POINT ( 'NONE',  ( 90.00000000000000000, 26.00000000000000355, 2.099999999999989875 ) ) ;
#636=B_SPLINE_CURVE_WITH_KNOTS ( 'NONE', 3,
 ( #6378, #17250, #4785, #15175, #18648, #11867, #2952, #18868, #17137, #1455, #1560, #9926, #1216, #22200, #6493, #19858 ),
 .UNSPECIFIED., .F., .F.,
 ( 4, 2, 2, 2, 2, 2, 2, 4 ),
 ( 0.000000000000000000, 0.004782611835060888474, 0.005978264793826106906, 0.007173917752591319266, 0.009565223670121737048, 0.01195652958765215483, 0.01434783550518257435, 0.01913044734024341512 ),
 .UNSPECIFIED. ) ;
#637=EDGE_CURVE ( 'NONE', #15664, #18218, #10005, .T. ) ;
#640=CIRCLE ( 'NONE', #11227, 2.499999999999995115 ) ;
#641=CARTESIAN_POINT ( 'NONE',  ( -42.50000000000000711, -5.000000000000000000, 41.00000000000000711 ) ) ;
#642=CARTESIAN_POINT ( 'NONE',  ( 90.00000000000000000, 26.00000000000000355, -2.099999999999991651 ) ) ;
#646=EDGE_CURVE ( 'NONE', #11081, #11262, #14027, .T. ) ;
#647=DIRECTION ( 'NONE',  ( 0.000000000000000000, 0.000000000000000000, -1.000000000000000000 ) ) ;
#652=AXIS2_PLACEMENT_3D ( 'NONE', #13595, #1481, #11895 ) ;
#653=EDGE_LOOP ( 'NONE', ( #11685, #3181, #17197, #9101 ) ) ;
#654=VECTOR ( 'NONE', #4707, 1000.000000000000000 ) ;
#658=DIRECTION ( 'NONE',  ( 0.000000000000000000, 0.000000000000000000, 1.000000000000000000 ) ) ;
#663=CARTESIAN_POINT ( 'NONE',  ( 6.699391982047661287, -4.821764332415560794, 49.69317737456783846 ) ) ;
#670=DIRECTION ( 'NONE',  ( -1.000000000000000000, 0.000000000000000000, 0.000000000000000000 ) ) ;
#671=DIRECTION ( 'NONE',  ( -0.000000000000000000, -0.000000000000000000, 1.000000000000000000 ) ) ;
#675=VERTEX_POINT ( 'NONE', #8986 ) ;
#677=DIRECTION ( 'NONE',  ( -0.000000000000000000, -0.000000000000000000, -1.000000000000000000 ) ) ;
#678=CARTESIAN_POINT ( 'NONE',  ( -35.00000000000000000, -9.000000000000001776, -17.99999999999998934 ) ) ;
#679=ADVANCED_FACE ( 'NONE', ( #11272 ), #21599, .F. ) ;
#680=EDGE_CURVE ( 'NONE', #9888, #4267, #16975, .T. ) ;
#681=B_SPLINE_CURVE_WITH_KNOTS ( 'NONE', 1,
 ( #16046, #17548 ),
 .UNSPECIFIED., .F., .F.,
 ( 2, 2 ),
 ( 0.000000000000000000, 1.000000000000000000 ),
 .UNSPECIFIED. ) ;
#685=CONICAL_SURFACE ( 'NONE', #20455, 2.099999999999997868, 1.029744258676653867 ) ;
#690=VECTOR ( 'NONE', #4946, 1000.000000000000000 ) ;
#692=CARTESIAN_POINT ( 'NONE',  ( 1.105958719418588032, 39.99272030489618857, -49.57516106150625035 ) ) ;
#695=EDGE_LOOP ( 'NONE', ( #15730, #4327, #172, #15716, #13591, #19027, #8915 ) ) ;
#696=CARTESIAN_POINT ( 'NONE',  ( 42.50000000000000711, -11.97499999999999964, 50.00000000000000711 ) ) ;
#697=CARTESIAN_POINT ( 'NONE',  ( -9.867969867547959240, 0.2954100743916240890, -54.30456930252523051 ) ) ;
#698=EDGE_LOOP ( 'NONE', ( #8656, #15794, #19959, #10887 ) ) ;
#701=CYLINDRICAL_SURFACE ( 'NONE', #14041, 2.500000000000002220 ) ;
#703=ORIENTED_EDGE ( 'NONE', *, *, #22176, .T. ) ;
#707=CARTESIAN_POINT ( 'NONE',  ( -0.09263077948485531898, 39.99995274011368451, -48.80595708259651389 ) ) ;
#709=DIRECTION ( 'NONE',  ( 0.000000000000000000, -0.5150380749100547106, -0.8571673007021120005 ) ) ;
#711=CARTESIAN_POINT ( 'NONE',  ( -13.07600923154787864, 27.35939529837144590, 44.93756990742566870 ) ) ;
#712=DIRECTION ( 'NONE',  ( 0.000000000000000000, 0.000000000000000000, 1.000000000000000000 ) ) ;
#714=ORIENTED_EDGE ( 'NONE', *, *, #18426, .F. ) ;
#715=ORIENTED_EDGE ( 'NONE', *, *, #1941, .F. ) ;
#720=CARTESIAN_POINT ( 'NONE',  ( 19.01465036493455685, 26.21927150370769510, 60.37937655616645571 ) ) ;
#724=CARTESIAN_POINT ( 'NONE',  ( 35.00000000000000000, 0.000000000000000000, -49.99999999999997868 ) ) ;
#725=ORIENTED_EDGE ( 'NONE', *, *, #5057, .T. ) ;
#729=CARTESIAN_POINT ( 'NONE',  ( 34.99999999999980815, 26.00000000000000355, 57.09999999999921982 ) ) ;
#731=CARTESIAN_POINT ( 'NONE',  ( -20.67483659015370989, 11.23071942442636661, -58.26617649125748954 ) ) ;
#733=DIRECTION ( 'NONE',  ( 0.000000000000000000, 0.000000000000000000, -1.000000000000000000 ) ) ;
#736=CARTESIAN_POINT ( 'NONE',  ( 35.00000000000058265, 40.00000000000000000, -57.50000000000076028 ) ) ;
#737=ORIENTED_EDGE ( 'NONE', *, *, #18385, .T. ) ;
#738=CARTESIAN_POINT ( 'NONE',  ( 0.7832247060116511728, 40.00000000000097344, 49.34584201034998330 ) ) ;
#742=CIRCLE ( 'NONE', #8713, 2.499999999999995115 ) ;
#745=ORIENTED_EDGE ( 'NONE', *, *, #22049, .T. ) ;
#747=ORIENTED_EDGE ( 'NONE', *, *, #16037, .F. ) ;
#753=DIRECTION ( 'NONE',  ( 0.000000000000000000, -0.000000000000000000, -1.000000000000000000 ) ) ;
#757=ADVANCED_FACE ( 'NONE', ( #19874, #4184, #394, #12758, #16084, #21830, #9335 ), #6125, .T. ) ;
#759=DIRECTION ( 'NONE',  ( 0.000000000000000000, 1.000000000000000000, 0.000000000000000000 ) ) ;
#761=CYLINDRICAL_SURFACE ( 'NONE', #958, 2.500000000000002220 ) ;
#765=CARTESIAN_POINT ( 'NONE',  ( -1.387778780781445518E-14, 20.00000000000000355, -102.0000000000000142 ) ) ;
#769=ADVANCED_FACE ( 'NONE', ( #14353 ), #18824, .F. ) ;
#770=VECTOR ( 'NONE', #3039, 1000.000000000000114 ) ;
#771=EDGE_LOOP ( 'NONE', ( #13106, #15939, #8345, #9673 ) ) ;
#772=DIRECTION ( 'NONE',  ( -0.000000000000000000, -1.000000000000000000, -0.000000000000000000 ) ) ;
#773=CARTESIAN_POINT ( 'NONE',  ( -18.00000000000001421, 20.00000000000000355, -102.9999999999999716 ) ) ;
#774=CARTESIAN_POINT ( 'NONE',  ( 3.315551171827967991, 0.2472631163744288263, -51.08212483308732743 ) ) ;
#775=EDGE_CURVE ( 'NONE', #15249, #1751, #7841, .T. ) ;
#776=ADVANCED_FACE ( 'NONE', ( #12637 ), #12640, .F. ) ;
#777=EDGE_CURVE ( 'NONE', #10435, #18495, #16621, .T. ) ;
#778=DIRECTION ( 'NONE',  ( 0.000000000000000000, 0.000000000000000000, 1.000000000000000000 ) ) ;
#785=EDGE_CURVE ( 'NONE', #21816, #1314, #14411, .T. ) ;
#786=CARTESIAN_POINT ( 'NONE',  ( -6.401904815323844922, 38.95163572918602313, -55.13655742298576001 ) ) ;
#787=CARTESIAN_POINT ( 'NONE',  ( 28.49999999999998224, 19.99999999999999645, 100.0000000000000000 ) ) ;
#789=EDGE_CURVE ( 'NONE', #1700, #2703, #7118, .T. ) ;
#790=VERTEX_POINT ( 'NONE', #3368 ) ;
#791=ORIENTED_EDGE ( 'NONE', *, *, #16352, .T. ) ;
#792=CARTESIAN_POINT ( 'NONE',  ( 35.00000000000000000, 38.99999999999999289, -59.99999999999999289 ) ) ;
#796=CYLINDRICAL_SURFACE ( 'NONE', #18437, 2.099999999999997868 ) ;
#797=AXIS2_PLACEMENT_3D ( 'NONE', #6808, #136, #18008 ) ;
#798=CARTESIAN_POINT ( 'NONE',  ( 4.846088107612517959, 40.00000000000000000, -51.53252798484124497 ) ) ;
#799=ORIENTED_EDGE ( 'NONE', *, *, #20849, .F. ) ;
#800=CARTESIAN_POINT ( 'NONE',  ( 7.213743607555469950, 39.66007621396295946, -53.46062051868064202 ) ) ;
#806=CARTESIAN_POINT ( 'NONE',  ( -6.910507445196895304, 40.00000000000002132, 52.51112221451682416 ) ) ;
#810=DIRECTION ( 'NONE',  ( 0.000000000000000000, 1.000000000000000000, 0.000000000000000000 ) ) ;
#812=CARTESIAN_POINT ( 'NONE',  ( -0.02199734621860905542, 39.99999719748067406, -48.75108928016371124 ) ) ;
#818=ORIENTED_EDGE ( 'NONE', *, *, #18319, .T. ) ;
#819=ORIENTED_EDGE ( 'NONE', *, *, #12527, .T. ) ;
#821=CARTESIAN_POINT ( 'NONE',  ( 5.748506628226523141, -0.6819283742239256041, 52.01451867725413081 ) ) ;
#823=CIRCLE ( 'NONE', #18392, 22.00000000000000000 ) ;
#825=DIRECTION ( 'NONE',  ( 1.049727191138617217E-16, 0.5150380749100562650, -0.8571673007021111124 ) ) ;
#826=CARTESIAN_POINT ( 'NONE',  ( -34.99999999999980815, 40.00000000000000711, 54.99999999999922551 ) ) ;
#828=CARTESIAN_POINT ( 'NONE',  ( 9.952189117650823036, 40.00000000000000000, 53.64426396172073197 ) ) ;
#831=CARTESIAN_POINT ( 'NONE',  ( -11.13407802442742245, 9.941921282207680122, -43.93745127716449872 ) ) ;
#832=VECTOR ( 'NONE', #9450, 1000.000000000000000 ) ;
#834=CARTESIAN_POINT ( 'NONE',  ( 19.04641992693177244, 13.69305383064222603, -60.38882653684736823 ) ) ;
#839=CARTESIAN_POINT ( 'NONE',  ( 3.630513325115385381, 39.68566305962351493, 51.94955563033850865 ) ) ;
#841=CARTESIAN_POINT ( 'NONE',  ( -6.001999869223751283, -0.8367338791974072709, -52.11627801855959063 ) ) ;
#843=CARTESIAN_POINT ( 'NONE',  ( 11.54473802383823511, 36.35512261685320823, 55.24115706042309881 ) ) ;
#844=DIRECTION ( 'NONE',  ( 0.000000000000000000, 0.000000000000000000, 1.000000000000000000 ) ) ;
#846=DIRECTION ( 'NONE',  ( 0.000000000000000000, -0.000000000000000000, -1.000000000000000000 ) ) ;
#847=AXIS2_PLACEMENT_3D ( 'NONE', #14671, #11121, #712 ) ;
#848=EDGE_CURVE ( 'NONE', #18961, #6724, #20651, .T. ) ;
#850=ORIENTED_EDGE ( 'NONE', *, *, #1184, .T. ) ;
#851=ORIENTED_EDGE ( 'NONE', *, *, #6390, .T. ) ;
#853=CARTESIAN_POINT ( 'NONE',  ( 11.12045539253394821, 39.12082365973188303, 55.06303111140292827 ) ) ;
#856=CARTESIAN_POINT ( 'NONE',  ( -17.00000000000002842, 20.00000000000000355, -102.0000000000000142 ) ) ;
#857=ORIENTED_EDGE ( 'NONE', *, *, #19356, .F. ) ;
#860=ORIENTED_EDGE ( 'NONE', *, *, #4382, .T. ) ;
#861=CIRCLE ( 'NONE', #8544, 2.499999999999995115 ) ;
#862=VERTEX_POINT ( 'NONE', #13878 ) ;
#866=CARTESIAN_POINT ( 'NONE',  ( -0.2719375495013811039, 39.99956352816811034, 48.94448636964621357 ) ) ;
#867=TOROIDAL_SURFACE ( 'NONE', #1956, 50.00000000000000000, 10.00000000000000000 ) ;
#868=VECTOR ( 'NONE', #22657, 1000.000000000000000 ) ;
#869=CARTESIAN_POINT ( 'NONE',  ( -0.7060564148929356909, 40.00000000000297007, 49.41654780795607849 ) ) ;
#871=EDGE_CURVE ( 'NONE', #15231, #21079, #14775, .T. ) ;
#874=ORIENTED_EDGE ( 'NONE', *, *, #14173, .F. ) ;
#876=VECTOR ( 'NONE', #4480, 1000.000000000000000 ) ;
#878=CARTESIAN_POINT ( 'NONE',  ( -19.80158170751280977, 22.94611027470400089, 60.57464962002575959 ) ) ;
#879=ADVANCED_FACE ( 'NONE', ( #8621, #20896 ), #5197, .F. ) ;
#882=CARTESIAN_POINT ( 'NONE',  ( -0.3446551741029754701, -0.009348518860373671718, -50.24945914274646697 ) ) ;
#884=AXIS2_PLACEMENT_3D ( 'NONE', #22625, #19477, #2053 ) ;
#887=CARTESIAN_POINT ( 'NONE',  ( -4.628075497661881421, 39.46063506869896997, -53.65703709786517805 ) ) ;
#889=CARTESIAN_POINT ( 'NONE',  ( 35.00000000000058265, 40.00000000000000000, -52.90000000000076597 ) ) ;
#891=PRODUCT ( 'CASE', 'CASE', '', ( #13512 ) ) ;
#894=EDGE_LOOP ( 'NONE', ( #6024, #21589, #6688, #10460 ) ) ;
#895=DIRECTION ( 'NONE',  ( 0.000000000000000000, 0.000000000000000000, -1.000000000000000000 ) ) ;
#897=DIRECTION ( 'NONE',  ( 0.000000000000000000, 0.7071067811866457165, 0.7071067811864494290 ) ) ;
#900=LINE ( 'NONE', #4353, #17009 ) ;
#903=EDGE_CURVE ( 'NONE', #13935, #5360, #8572, .T. ) ;
#906=ORIENTED_EDGE ( 'NONE', *, *, #22508, .T. ) ;
#911=CARTESIAN_POINT ( 'NONE',  ( 0.5525046371098545350, 39.99819307499277699, -49.15917675262092246 ) ) ;
#914=ADVANCED_FACE ( 'NONE', ( #16533 ), #19558, .F. ) ;
#915=DIRECTION ( 'NONE',  ( -0.000000000000000000, 1.000000000000000000, -0.000000000000000000 ) ) ;
#917=CARTESIAN_POINT ( 'NONE',  ( -15.97698236194133159, 7.938033795522204450, -59.50430813415450615 ) ) ;
#922=VERTEX_POINT ( 'NONE', #11605 ) ;
#923=CARTESIAN_POINT ( 'NONE',  ( 35.00000000000058265, 26.00000000000000355, -55.00000000000076028 ) ) ;
#926=DIRECTION ( 'NONE',  ( -0.000000000000000000, -1.000000000000000000, -0.000000000000000000 ) ) ;
#927=CIRCLE ( 'NONE', #18856, 2.099999999999997868 ) ;
#929=CARTESIAN_POINT ( 'NONE',  ( -14.76055860720890500, 22.69766935715934153, 45.72055682016589628 ) ) ;
#932=ORIENTED_EDGE ( 'NONE', *, *, #1320, .T. ) ;
#933=EDGE_CURVE ( 'NONE', #11968, #13427, #9674, .T. ) ;
#935=B_SPLINE_CURVE_WITH_KNOTS ( 'NONE', 3,
 ( #21269, #3747, #5561, #17826, #19447, #174 ),
 .UNSPECIFIED., .F., .F.,
 ( 4, 2, 4 ),
 ( 1.991993874847888106E-18, 0.002694896630591175207, 0.005389793261182347812 ),
 .UNSPECIFIED. ) ;
#938=VERTEX_POINT ( 'NONE', #20206 ) ;
#939=CARTESIAN_POINT ( 'NONE',  ( 16.16780438139466014, 31.78273399965604540, 59.56292242448185448 ) ) ;
#947=CARTESIAN_POINT ( 'NONE',  ( -14.17374118098246605, 15.07546459525165261, -45.45638825402599537 ) ) ;
#949=CARTESIAN_POINT ( 'NONE',  ( 16.97539716422056699, 9.395639044392945394, -59.81372721910505419 ) ) ;
#951=CARTESIAN_POINT ( 'NONE',  ( -3.179547497537916545, 39.99999999999999289, -50.65098726527259743 ) ) ;
#952=CARTESIAN_POINT ( 'NONE',  ( 0.3104238174410367535, 39.99820335227857271, -49.10409449009593175 ) ) ;
#954=CARTESIAN_POINT ( 'NONE',  ( -18.00000000000001421, 20.00000000000000711, 103.0000000000000284 ) ) ;
#957=AXIS2_PLACEMENT_3D ( 'NONE', #1200, #4989, #11969 ) ;
#958=AXIS2_PLACEMENT_3D ( 'NONE', #6027, #9689, #16676 ) ;
#964=CARTESIAN_POINT ( 'NONE',  ( 19.96647043697146984, 18.54527240924682729, -60.61386395554088580 ) ) ;
#966=ADVANCED_FACE ( 'NONE', ( #6228 ), #11858, .F. ) ;
#967=EDGE_LOOP ( 'NONE', ( #20857, #1137, #9405, #12556 ) ) ;
#971=CIRCLE ( 'NONE', #22574, 2.499999999999996891 ) ;
#973=CARTESIAN_POINT ( 'NONE',  ( 10.81645871535806336, 39.16817317914274810, 54.94897387137724110 ) ) ;
#976=ORIENTED_EDGE ( 'NONE', *, *, #16314, .T. ) ;
#979=ORIENTED_EDGE ( 'NONE', *, *, #10273, .F. ) ;
#981=AXIS2_PLACEMENT_3D ( 'NONE', #21390, #5359, #15768 ) ;
#983=CARTESIAN_POINT ( 'NONE',  ( -1.485717122675833668, -1.299971956346735791, -49.29290837556842320 ) ) ;
#987=ADVANCED_FACE ( 'NONE', ( #11375 ), #158, .F. ) ;
#990=EDGE_LOOP ( 'NONE', ( #5095, #11437, #19565, #9961 ) ) ;
#991=VECTOR ( 'NONE', #14455, 1000.000000000000000 ) ;
#992=ORIENTED_EDGE ( 'NONE', *, *, #14848, .T. ) ;
#994=CARTESIAN_POINT ( 'NONE',  ( -20.65262896361484835, 28.82759387226903769, 58.26038807538093778 ) ) ;
#996=AXIS2_PLACEMENT_3D ( 'NONE', #6782, #6667, #13523 ) ;
#998=CARTESIAN_POINT ( 'NONE',  ( -11.45074849662542782, 39.99999999999999289, 54.12667998692793958 ) ) ;
#999=DIRECTION ( 'NONE',  ( 0.000000000000000000, 0.000000000000000000, 1.000000000000000000 ) ) ;
#1000=CARTESIAN_POINT ( 'NONE',  ( -90.00000000000000000, 40.00000000000000711, -2.525000000000000355 ) ) ;
#1001=CARTESIAN_POINT ( 'NONE',  ( 3.210598435713497345, 39.75302854575188150, 52.30739040051271616 ) ) ;
#1003=CARTESIAN_POINT ( 'NONE',  ( -2.568452277497750937E-14, 40.00000000000000000, -48.73397172404482092 ) ) ;
#1004=ADVANCED_FACE ( 'NONE', ( #2680 ), #15298, .T. ) ;
#1005=EDGE_LOOP ( 'NONE', ( #5740, #22368, #2661, #14334 ) ) ;
#1007=AXIS2_PLACEMENT_3D ( 'NONE', #13919, #17486, #21158 ) ;
#1014=AXIS2_PLACEMENT_3D ( 'NONE', #14105, #8524, #15499 ) ;
#1016=CARTESIAN_POINT ( 'NONE',  ( -42.50000000000000711, -11.97499999999999964, -45.00000000000000000 ) ) ;
#1018=AXIS2_PLACEMENT_3D ( 'NONE', #22227, #12123, #15545 ) ;
#1021=AXIS2_PLACEMENT_3D ( 'NONE', #20944, #11063, #530 ) ;
#1023=ORIENTED_EDGE ( 'NONE', *, *, #11379, .T. ) ;
#1024=CARTESIAN_POINT ( 'NONE',  ( 3.072145818613496449, 39.94358020626381744, -50.97359800879427638 ) ) ;
#1026=CIRCLE ( 'NONE', #652, 2.500000000000002220 ) ;
#1030=CARTESIAN_POINT ( 'NONE',  ( -5.004759427256008308, 40.00000000000000000, 51.61237555825404399 ) ) ;
#1031=ADVANCED_FACE ( 'NONE', ( #10212 ), #3584, .T. ) ;
#1033=AXIS2_PLACEMENT_3D ( 'NONE', #8268, #15697, #15237 ) ;
#1036=EDGE_LOOP ( 'NONE', ( #13313, #7843, #1348, #16196 ) ) ;
#1037=CARTESIAN_POINT ( 'NONE',  ( 14.04383866228953792, 25.28361825225916704, 45.39674436955350956 ) ) ;
#1040=CARTESIAN_POINT ( 'NONE',  ( 12.99999999999993960, 42.51666049839543149, 60.00099999999999767 ) ) ;
#1042=DIRECTION ( 'NONE',  ( -0.000000000000000000, -0.000000000000000000, -1.000000000000000000 ) ) ;
#1045=CARTESIAN_POINT ( 'NONE',  ( -14.05436202270911217, 25.29714423467776996, 45.40204559108968141 ) ) ;
#1049=CIRCLE ( 'NONE', #8360, 2.499999999999998668 ) ;
#1055=CARTESIAN_POINT ( 'NONE',  ( 14.31751149541521784, 33.97259629115305302, -58.93694582298954998 ) ) ;
#1058=CARTESIAN_POINT ( 'NONE',  ( -34.99999999999999289, 0.000000000000000000, 50.00000000000000000 ) ) ;
#1059=VECTOR ( 'NONE', #10373, 1000.000000000000000 ) ;
#1067=EDGE_CURVE ( 'NONE', #17407, #7645, #438, .T. ) ;
#1070=LINE ( 'NONE', #609, #17776 ) ;
#1074=CARTESIAN_POINT ( 'NONE',  ( -5.234365469061698306, 40.00000000000000711, -51.72901482534432205 ) ) ;
#1075=CARTESIAN_POINT ( 'NONE',  ( 8.331955809010596070, 38.18181818181818699, -56.36098470834070895 ) ) ;
#1077=CARTESIAN_POINT ( 'NONE',  ( 9.375581681113587251, 39.53990230686088836, 54.37755644423855017 ) ) ;
#1078=FACE_OUTER_BOUND ( 'NONE', #20598, .T. ) ;
#1079=CARTESIAN_POINT ( 'NONE',  ( -2.951413581184478829, -1.204958657596112870, -50.23354289400218420 ) ) ;
#1083=CARTESIAN_POINT ( 'NONE',  ( -15.00000000000001421, 20.00000000000000000, -101.0000000000000284 ) ) ;
#1084=CARTESIAN_POINT ( 'NONE',  ( 19.64963058618602787, 23.83053889023033634, -60.53829769526750937 ) ) ;
#1085=AXIS2_PLACEMENT_3D ( 'NONE', #4347, #671, #12905 ) ;
#1090=CARTESIAN_POINT ( 'NONE',  ( 11.25639079644659724, 39.09917355294047780, 55.11545576760340026 ) ) ;
#1092=ORIENTED_EDGE ( 'NONE', *, *, #11379, .F. ) ;
#1097=CARTESIAN_POINT ( 'NONE',  ( 12.09218358684717920, 1.291952833853752924, 55.42846997241154838 ) ) ;
#1098=AXIS2_PLACEMENT_3D ( 'NONE', #16217, #413, #16338 ) ;
#1100=DIRECTION ( 'NONE',  ( 0.000000000000000000, 0.000000000000000000, 1.000000000000000000 ) ) ;
#1101=DIRECTION ( 'NONE',  ( -0.000000000000000000, -1.000000000000000000, -0.000000000000000000 ) ) ;
#1102=CARTESIAN_POINT ( 'NONE',  ( -18.50805780747144880, 27.59542556733953944, -60.24679276096814817 ) ) ;
#1104=EDGE_CURVE ( 'NONE', #14723, #11771, #19837, .T. ) ;
#1106=CARTESIAN_POINT ( 'NONE',  ( 10.30713387248687773, 2.842164160680653584, -57.27491564205610786 ) ) ;
#1107=ADVANCED_FACE ( 'NONE', ( #21321 ), #701, .F. ) ;
#1111=ORIENTED_EDGE ( 'NONE', *, *, #17841, .F. ) ;
#1112=CARTESIAN_POINT ( 'NONE',  ( -19.96647043697144852, 18.54527240924516818, 60.61386395554428219 ) ) ;
#1113=DIRECTION ( 'NONE',  ( -1.000000000000000000, 0.000000000000000000, 0.000000000000000000 ) ) ;
#1115=CARTESIAN_POINT ( 'NONE',  ( -11.28246622563948520, 40.00000000000000711, 54.06713842414183802 ) ) ;
#1117=ORIENTED_EDGE ( 'NONE', *, *, #4115, .T. ) ;
#1119=CARTESIAN_POINT ( 'NONE',  ( -34.99999999999980815, 40.00000000000000000, 54.99999999999922551 ) ) ;
#1121=CARTESIAN_POINT ( 'NONE',  ( -5.133444049470117676, 39.34078687931064167, -53.02546735988109816 ) ) ;
#1122=DIRECTION ( 'NONE',  ( 0.000000000000000000, 0.000000000000000000, 1.000000000000000000 ) ) ;
#1123=ORIENTED_EDGE ( 'NONE', *, *, #11097, .F. ) ;
#1126=DIRECTION ( 'NONE',  ( 0.000000000000000000, -0.000000000000000000, -1.000000000000000000 ) ) ;
#1132=AXIS2_PLACEMENT_3D ( 'NONE', #8155, #6437, #14895 ) ;
#1135=CARTESIAN_POINT ( 'NONE',  ( -4.044995508448087307, -4.680814751541408469, 48.25214090642531772 ) ) ;
#1136=DIRECTION ( 'NONE',  ( -0.000000000000000000, -1.000000000000000000, -0.000000000000000000 ) ) ;
#1137=ORIENTED_EDGE ( 'NONE', *, *, #19566, .F. ) ;
#1142=CARTESIAN_POINT ( 'NONE',  ( 10.77132920883424205, 39.17511451497404806, -54.93228420922696387 ) ) ;
#1143=FACE_OUTER_BOUND ( 'NONE', #9305, .T. ) ;
#1147=CARTESIAN_POINT ( 'NONE',  ( 6.041077103367500811, -0.8288449397161629095, 52.13906252460464685 ) ) ;
#1148=CARTESIAN_POINT ( 'NONE',  ( 8.219889501001356180, 1.750964516533152437, -56.08920281153656617 ) ) ;
#1149=CARTESIAN_POINT ( 'NONE',  ( -1.387778780781445676E-14, 40.00000000000000000, -48.73397172404481381 ) ) ;
#1150=VERTEX_POINT ( 'NONE', #19494 ) ;
#1151=EDGE_CURVE ( 'NONE', #1471, #10193, #15429, .T. ) ;
#1155=EDGE_CURVE ( 'NONE', #18643, #19011, #9589, .T. ) ;
#1159=CARTESIAN_POINT ( 'NONE',  ( 19.41351212956690730, 24.83257706694782030, -60.47995209899215041 ) ) ;
#1161=CARTESIAN_POINT ( 'NONE',  ( 5.833333333333336590, 39.00000000000000711, 40.61164310337068173 ) ) ;
#1162=DIRECTION ( 'NONE',  ( 1.000000000000000000, 0.000000000000000000, 0.000000000000000000 ) ) ;
#1163=DIRECTION ( 'NONE',  ( 0.000000000000000000, 0.000000000000000000, 1.000000000000000000 ) ) ;
#1164=CARTESIAN_POINT ( 'NONE',  ( 0.5279010140432808251, 4.999719073153301885, -38.73355033370100386 ) ) ;
#1166=DIRECTION ( 'NONE',  ( -1.000000000000000000, 0.000000000000000000, 0.000000000000000000 ) ) ;
#1168=ORIENTED_EDGE ( 'NONE', *, *, #20660, .T. ) ;
#1171=LINE ( 'NONE', #6331, #5023 ) ;
#1174=CARTESIAN_POINT ( 'NONE',  ( -1.387778780781445676E-14, 40.00000000000000000, -48.73397172404481381 ) ) ;
#1175=ORIENTED_EDGE ( 'NONE', *, *, #2779, .F. ) ;
#1176=LINE ( 'NONE', #13633, #12302 ) ;
#1177=EDGE_LOOP ( 'NONE', ( #4533, #4568 ) ) ;
#1181=DIRECTION ( 'NONE',  ( -0.000000000000000000, -0.000000000000000000, 1.000000000000000000 ) ) ;
#1182=CARTESIAN_POINT ( 'NONE',  ( 17.96966555604127791, 28.82469637350566671, -60.10139901455266198 ) ) ;
#1184=EDGE_CURVE ( 'NONE', #18333, #16148, #3013, .T. ) ;
#1185=ORIENTED_EDGE ( 'NONE', *, *, #5813, .F. ) ;
#1186=AXIS2_PLACEMENT_3D ( 'NONE', #12099, #19093, #17360 ) ;
#1187=VERTEX_POINT ( 'NONE', #10645 ) ;
#1188=EDGE_LOOP ( 'NONE', ( #4686, #20113, #19205, #17754, #20799, #14313 ) ) ;
#1190=CARTESIAN_POINT ( 'NONE',  ( 10.87562399044275274, 39.15903841214502279, 54.97094722865957550 ) ) ;
#1193=ORIENTED_EDGE ( 'NONE', *, *, #10418, .F. ) ;
#1195=CARTESIAN_POINT ( 'NONE',  ( -4.842578813368415780, -0.8535550256952800785, -51.47191290771856131 ) ) ;
#1197=DIRECTION ( 'NONE',  ( 0.000000000000000000, 0.000000000000000000, 1.000000000000000000 ) ) ;
#1198=CARTESIAN_POINT ( 'NONE',  ( 9.857944917837743404, 0.2919354798308393395, 54.29891737064654222 ) ) ;
#1200=CARTESIAN_POINT ( 'NONE',  ( 35.00000000000058265, 40.00000000000000000, -55.00000000000076028 ) ) ;
#1202=DIRECTION ( 'NONE',  ( 0.000000000000000000, 0.000000000000000000, -1.000000000000000000 ) ) ;
#1203=DIRECTION ( 'NONE',  ( -0.000000000000000000, -0.000000000000000000, -1.000000000000000000 ) ) ;
#1204=CARTESIAN_POINT ( 'NONE',  ( -12.24033418603700873, 35.84417766536505923, -58.14550894043696161 ) ) ;
#1205=AXIS2_PLACEMENT_3D ( 'NONE', #2980, #20505, #19016 ) ;
#1207=CARTESIAN_POINT ( 'NONE',  ( -14.92530643917655375, 18.45549920837825653, 45.79309713780078539 ) ) ;
#1209=ORIENTED_EDGE ( 'NONE', *, *, #1765, .F. ) ;
#1210=ADVANCED_FACE ( 'NONE', ( #5858 ), #7792, .F. ) ;
#1212=CARTESIAN_POINT ( 'NONE',  ( -18.15458487487865114, 6.756534690977250790, 57.58998093367232940 ) ) ;
#1216=CARTESIAN_POINT ( 'NONE',  ( -19.23800698326016700, 14.47374112874266316, -60.43633296823762890 ) ) ;
#1217=CARTESIAN_POINT ( 'NONE',  ( 9.075375594263590528, 39.43595020987488198, 54.33405310157220924 ) ) ;
#1218=AXIS2_PLACEMENT_3D ( 'NONE', #16052, #4046, #11014 ) ;
#1222=CARTESIAN_POINT ( 'NONE',  ( -13.00000000000011546, 42.51666049839536043, 105.0000000000000142 ) ) ;
#1225=ORIENTED_EDGE ( 'NONE', *, *, #15054, .T. ) ;
#1226=AXIS2_PLACEMENT_3D ( 'NONE', #17024, #22324, #13460 ) ;
#1227=CARTESIAN_POINT ( 'NONE',  ( -10.07716038413160220, 39.27871711242732289, 54.68297691402418792 ) ) ;
#1228=FACE_OUTER_BOUND ( 'NONE', #10168, .T. ) ;
#1232=CARTESIAN_POINT ( 'NONE',  ( -34.99999999999980815, 40.00000000000000000, 54.99999999999922551 ) ) ;
#1233=FACE_BOUND ( 'NONE', #5891, .T. ) ;
#1234=AXIS2_PLACEMENT_3D ( 'NONE', #18228, #14666, #5966 ) ;
#1239=CARTESIAN_POINT ( 'NONE',  ( -34.99999999999980815, 40.00000000000000711, 54.99999999999922551 ) ) ;
#1240=AXIS2_PLACEMENT_3D ( 'NONE', #16313, #6008, #623 ) ;
#1245=EDGE_CURVE ( 'NONE', #4801, #14603, #15791, .T. ) ;
#1246=FACE_OUTER_BOUND ( 'NONE', #2056, .T. ) ;
#1248=CARTESIAN_POINT ( 'NONE',  ( -19.67353980729183860, 23.69994786803828646, -58.06093965453396066 ) ) ;
#1249=AXIS2_PLACEMENT_3D ( 'NONE', #16047, #355, #4140 ) ;
#1250=CARTESIAN_POINT ( 'NONE',  ( -8.115799706357579524, 39.55796121550449129, 53.89994064586117872 ) ) ;
#1253=CARTESIAN_POINT ( 'NONE',  ( 11.13407802442741357, 30.05807871779230922, 43.93745127716450583 ) ) ;
#1257=DIRECTION ( 'NONE',  ( 0.000000000000000000, 0.000000000000000000, -1.000000000000000000 ) ) ;
#1258=EDGE_CURVE ( 'NONE', #19899, #11765, #2874, .T. ) ;
#1268=SHAPE_DEFINITION_REPRESENTATION ( #11514, #21292 ) ;
#1269=B_SPLINE_CURVE_WITH_KNOTS ( 'NONE', 3,
 ( #20292, #4596, #1147, #15100, #20405, #4714 ),
 .UNSPECIFIED., .F., .F.,
 ( 4, 2, 4 ),
 ( 1.116583492552567205E-17, 0.005389490931280165216, 0.01077898186256031829 ),
 .UNSPECIFIED. ) ;
#1270=EDGE_LOOP ( 'NONE', ( #4084, #14632, #16343, #5836 ) ) ;
#1274=CARTESIAN_POINT ( 'NONE',  ( 34.99999999999980815, 40.00000000000000711, 54.99999999999922551 ) ) ;
#1279=LINE ( 'NONE', #2904, #17100 ) ;
#1282=FACE_BOUND ( 'NONE', #19366, .T. ) ;
#1285=CARTESIAN_POINT ( 'NONE',  ( 8.847970474273168406, 40.00000000000000711, 53.28481329029794011 ) ) ;
#1286=VERTEX_POINT ( 'NONE', #20172 ) ;
#1287=CARTESIAN_POINT ( 'NONE',  ( -8.197131438766653844, 40.00000000000000711, -53.04141935927233931 ) ) ;
#1289=DIRECTION ( 'NONE',  ( -0.000000000000000000, -0.000000000000000000, 1.000000000000000000 ) ) ;
#1290=CARTESIAN_POINT ( 'NONE',  ( -6.626710883749606351E-15, -0.4099546584827634121, -48.99240008041271466 ) ) ;
#1294=DIRECTION ( 'NONE',  ( -1.000000000000000000, 0.000000000000000000, 0.000000000000000000 ) ) ;
#1295=EDGE_CURVE ( 'NONE', #11321, #18787, #22415, .T. ) ;
#1296=CARTESIAN_POINT ( 'NONE',  ( 21.83670385715308271, 14.52494903933254911, -58.53909266577284143 ) ) ;
#1298=CIRCLE ( 'NONE', #18126, 2.099999999999997868 ) ;
#1299=ORIENTED_EDGE ( 'NONE', *, *, #14707, .F. ) ;
#1300=ORIENTED_EDGE ( 'NONE', *, *, #1610, .F. ) ;
#1301=PLANE ( 'NONE',  #6546 ) ;
#1305=EDGE_CURVE ( 'NONE', #5648, #21174, #12867, .T. ) ;
#1308=CARTESIAN_POINT ( 'NONE',  ( -6.661198439252719261, -4.819795714544886422, -49.67388352366067750 ) ) ;
#1312=CIRCLE ( 'NONE', #2406, 2.500000000000002220 ) ;
#1314=VERTEX_POINT ( 'NONE', #11574 ) ;
#1315=CARTESIAN_POINT ( 'NONE',  ( 5.204790488456048969, 39.83796511861606859, -52.32473449166996460 ) ) ;
#1316=AXIS2_PLACEMENT_3D ( 'NONE', #12247, #4233, #13025 ) ;
#1320=EDGE_CURVE ( 'NONE', #19781, #3437, #5567, .T. ) ;
#1323=CARTESIAN_POINT ( 'NONE',  ( -9.855264211176372413, 8.670295722316108566, 43.22210574525161064 ) ) ;
#1327=ORIENTED_EDGE ( 'NONE', *, *, #3809, .T. ) ;
#1329=ORIENTED_EDGE ( 'NONE', *, *, #637, .T. ) ;
#1330=CARTESIAN_POINT ( 'NONE',  ( -22.43750227530606978, 20.33721733311116253, 58.67013217117688839 ) ) ;
#1335=CARTESIAN_POINT ( 'NONE',  ( -11.16030968682941804, 40.00000000000000000, 54.02479386262969996 ) ) ;
#1337=EDGE_LOOP ( 'NONE', ( #4788, #4078 ) ) ;
#1339=CARTESIAN_POINT ( 'NONE',  ( -6.019227127673981492, 39.99999999999999289, -52.10376796897383400 ) ) ;
#1340=EDGE_CURVE ( 'NONE', #7376, #22334, #6534, .T. ) ;
#1346=DIRECTION ( 'NONE',  ( -0.000000000000000000, -1.000000000000000000, -0.000000000000000000 ) ) ;
#1348=ORIENTED_EDGE ( 'NONE', *, *, #7352, .T. ) ;
#1350=DIRECTION ( 'NONE',  ( 0.000000000000000000, 0.000000000000000000, -1.000000000000000000 ) ) ;
#1352=DIRECTION ( 'NONE',  ( 0.000000000000000000, 0.000000000000000000, -1.000000000000000000 ) ) ;
#1358=DIRECTION ( 'NONE',  ( -0.000000000000000000, 1.000000000000000000, -0.000000000000000000 ) ) ;
#1362=CARTESIAN_POINT ( 'NONE',  ( -5.833333333333341919, 33.81926995981417150, -40.61164310337066041 ) ) ;
#1364=CARTESIAN_POINT ( 'NONE',  ( -20.31722544680652476, 29.72987180553229791, -58.17992760854140499 ) ) ;
#1367=CARTESIAN_POINT ( 'NONE',  ( -16.64903669413044085, 31.11586081922098757, 59.71532480898648743 ) ) ;
#1371=CARTESIAN_POINT ( 'NONE',  ( 12.84005703541281207, 1.693876179768766699, -55.76322220626109072 ) ) ;
#1372=CARTESIAN_POINT ( 'NONE',  ( 6.696867368503558448E-15, 40.00000000000000000, 39.73397172404484223 ) ) ;
#1376=DIRECTION ( 'NONE',  ( 0.4124789556921644729, -0.7071067811865296981, -0.5743353646704393300 ) ) ;
#1383=VERTEX_POINT ( 'NONE', #18561 ) ;
#1389=CARTESIAN_POINT ( 'NONE',  ( 3.174475770757817727, -4.645331003331005348, 47.72510079651066661 ) ) ;
#1390=CARTESIAN_POINT ( 'NONE',  ( -34.99999999999980815, 39.97500000000000142, 54.99999999999922551 ) ) ;
#1392=CARTESIAN_POINT ( 'NONE',  ( -26.00000000000001421, 19.99999999999982947, -105.0010000000000048 ) ) ;
#1395=CARTESIAN_POINT ( 'NONE',  ( -11.51194040402259233, 39.05862814753313472, 55.21283662269736681 ) ) ;
#1396=ORIENTED_EDGE ( 'NONE', *, *, #848, .F. ) ;
#1397=FACE_OUTER_BOUND ( 'NONE', #4955, .T. ) ;
#1403=EDGE_LOOP ( 'NONE', ( #1123, #13567, #12653, #15852 ) ) ;
#1404=CARTESIAN_POINT ( 'NONE',  ( 11.84374239103369142, 29.21200678190360378, -44.31542800769554447 ) ) ;
#1409=AXIS2_PLACEMENT_3D ( 'NONE', #1876, #7030, #17340 ) ;
#1416=CIRCLE ( 'NONE', #9481, 30.00000000000000000 ) ;
#1417=CARTESIAN_POINT ( 'NONE',  ( 18.43720426448665961, 27.80056269872056163, -57.71457384194849993 ) ) ;
#1423=ORIENTED_EDGE ( 'NONE', *, *, #18959, .T. ) ;
#1425=DIRECTION ( 'NONE',  ( -0.000000000000000000, -1.000000000000000000, -0.000000000000000000 ) ) ;
#1428=CARTESIAN_POINT ( 'NONE',  ( 42.50000000000000711, -12.00000000000000000, 49.60000000000000853 ) ) ;
#1433=ADVANCED_FACE ( 'NONE', ( #20613 ), #4310, .F. ) ;
#1438=CARTESIAN_POINT ( 'NONE',  ( -1.044209099552145581, 39.99351895515111011, 49.52925835065091320 ) ) ;
#1443=ADVANCED_FACE ( 'NONE', ( #5341 ), #12144, .F. ) ;
#1445=ORIENTED_EDGE ( 'NONE', *, *, #22074, .T. ) ;
#1449=ORIENTED_EDGE ( 'NONE', *, *, #14657, .F. ) ;
#1450=CARTESIAN_POINT ( 'NONE',  ( -16.35275686153619645, 4.590993025983391540, 57.03319805596881054 ) ) ;
#1454=CARTESIAN_POINT ( 'NONE',  ( 1.080492130498492465, 39.99305441129651228, -49.55624281123191821 ) ) ;
#1455=CARTESIAN_POINT ( 'NONE',  ( -18.11182660255255428, 11.48022137427004097, -60.14030069439205306 ) ) ;
#1456=DIRECTION ( 'NONE',  ( -1.000000000000000000, 0.000000000000000000, 0.000000000000000000 ) ) ;
#1458=CARTESIAN_POINT ( 'NONE',  ( -35.00000000000058265, 40.00000000000000711, -55.00000000000076028 ) ) ;
#1459=CARTESIAN_POINT ( 'NONE',  ( -2.321955456489504854, 40.00000000000000000, -50.16149369290168636 ) ) ;
#1468=AXIS2_PLACEMENT_3D ( 'NONE', #529, #7523, #7638 ) ;
#1471=VERTEX_POINT ( 'NONE', #15518 ) ;
#1473=ORIENTED_EDGE ( 'NONE', *, *, #8027, .T. ) ;
#1474=CARTESIAN_POINT ( 'NONE',  ( -8.309432361859336424, 0.006312382049299974755, 53.49092837495744845 ) ) ;
#1478=CARTESIAN_POINT ( 'NONE',  ( 14.40375226887234206, 15.79546342576956164, 45.56106839101555295 ) ) ;
#1479=ADVANCED_FACE ( 'NONE', ( #4888 ), #22667, .F. ) ;
#1480=DIRECTION ( 'NONE',  ( -0.000000000000000000, -0.000000000000000000, -1.000000000000000000 ) ) ;
#1481=DIRECTION ( 'NONE',  ( -0.000000000000000000, 1.000000000000000000, -0.000000000000000000 ) ) ;
#1482=CARTESIAN_POINT ( 'NONE',  ( -22.42250004520216677, 20.31170080112651277, -58.66691407552180237 ) ) ;
#1484=EDGE_CURVE ( 'NONE', #1150, #5679, #16906, .T. ) ;
#1485=CARTESIAN_POINT ( 'NONE',  ( -8.331955809010626268, 38.18181818181818699, 56.36098470834075158 ) ) ;
#1494=DIRECTION ( 'NONE',  ( 0.000000000000000000, -0.7071067811865302533, -0.7071067811865647812 ) ) ;
#1497=ORIENTED_EDGE ( 'NONE', *, *, #12359, .T. ) ;
#1501=CARTESIAN_POINT ( 'NONE',  ( -40.40000000000001279, -9.600000000000001421, -47.50000000000000000 ) ) ;
#1502=CARTESIAN_POINT ( 'NONE',  ( -1.564319729173390128, -1.162775034690427534, 47.08282483555631615 ) ) ;
#1509=DIRECTION ( 'NONE',  ( 0.000000000000000000, 0.000000000000000000, -1.000000000000000000 ) ) ;
#1511=ORIENTED_EDGE ( 'NONE', *, *, #14720, .F. ) ;
#1514=DIRECTION ( 'NONE',  ( -0.000000000000000000, -1.000000000000000000, -0.000000000000000000 ) ) ;
#1515=CARTESIAN_POINT ( 'NONE',  ( 4.996179657326272228, 39.84467275760181337, 52.21079474515372709 ) ) ;
#1517=CARTESIAN_POINT ( 'NONE',  ( 11.37797799463863591, 29.78145794493465459, -44.06891764425670033 ) ) ;
#1520=CARTESIAN_POINT ( 'NONE',  ( -7.882609639814679786E-15, -9.552912840896525389E-26, -50.50395615645409464 ) ) ;
#1524=AXIS2_PLACEMENT_3D ( 'NONE', #5066, #8595, #12043 ) ;
#1525=AXIS2_PLACEMENT_3D ( 'NONE', #8048, #13175, #16519 ) ;
#1527=DIRECTION ( 'NONE',  ( 1.049727191138618326E-16, -0.5150380749100547106, 0.8571673007021120005 ) ) ;
#1532=ADVANCED_FACE ( 'NONE', ( #10360 ), #2668, .F. ) ;
#1535=CARTESIAN_POINT ( 'NONE',  ( 19.75454541434352862, 30.69619330606318997, 58.03277863335249975 ) ) ;
#1537=CARTESIAN_POINT ( 'NONE',  ( 7.763914066288519322, 40.00000000000000711, -52.86923209262808854 ) ) ;
#1538=VERTEX_POINT ( 'NONE', #18865 ) ;
#1539=CARTESIAN_POINT ( 'NONE',  ( -90.00000000000000000, 40.00000000000000000, -2.099999999999991651 ) ) ;
#1542=CARTESIAN_POINT ( 'NONE',  ( -6.976160265002656402, 1.175630724176373931, 53.22984522349711511 ) ) ;
#1544=ORIENTED_EDGE ( 'NONE', *, *, #3658, .T. ) ;
#1545=CARTESIAN_POINT ( 'NONE',  ( 8.620000862318205392, 38.06588505537628464, -54.65497975194055869 ) ) ;
#1548=CARTESIAN_POINT ( 'NONE',  ( -7.213741798857487453, 39.66007640230202469, 53.46061959581572154 ) ) ;
#1550=EDGE_CURVE ( 'NONE', #10325, #15602, #6308, .T. ) ;
#1560=CARTESIAN_POINT ( 'NONE',  ( -18.43548664438527851, 12.20444905678966308, -60.22785496272550176 ) ) ;
#1561=CARTESIAN_POINT ( 'NONE',  ( 0.5103185168914748937, 39.99845979616902270, 49.12706063236587539 ) ) ;
#1564=ORIENTED_EDGE ( 'NONE', *, *, #14623, .T. ) ;
#1568=CARTESIAN_POINT ( 'NONE',  ( 12.24744603030438839, 40.00000000000000000, -54.43639671998947449 ) ) ;
#1571=CARTESIAN_POINT ( 'NONE',  ( -18.52604901273059212, 27.59774142807035346, 60.25307787776294077 ) ) ;
#1572=ADVANCED_FACE ( 'NONE', ( #20929 ), #20220, .F. ) ;
#1576=CARTESIAN_POINT ( 'NONE',  ( -42.50000000000000711, -11.97499999999999964, 47.50000000000000711 ) ) ;
#1583=DIRECTION ( 'NONE',  ( -1.000000000000000000, 0.000000000000000000, 0.000000000000000000 ) ) ;
#1585=ORIENTED_EDGE ( 'NONE', *, *, #10418, .T. ) ;
#1586=CARTESIAN_POINT ( 'NONE',  ( 5.833333333333339255, 6.180730040185842711, 40.61164310337068173 ) ) ;
#1587=ADVANCED_FACE ( 'NONE', ( #15973 ), #12644, .T. ) ;
#1590=CARTESIAN_POINT ( 'NONE',  ( -22.42386962120398408, 19.82082524447363525, -58.66720683610021325 ) ) ;
#1592=B_SPLINE_SURFACE_WITH_KNOTS ( 'NONE', 1, 3, ( 
 ( #13655, #4977, #1873, #10231, #15611, #12077, #6928, #1537, #15496, #5206, #22516, #7027, #19628, #5423, #9192, #12841, #12735, #10784, #12401, #3936 ),
 ( #8855, #19412, #2209, #14218, #21233, #5525, #11130, #19751, #14332, #1980, #18128, #16167, #3713, #10663, #21340, #8963, #12500, #4055, #15943, #21578 ) ),
 .UNSPECIFIED., .F., .F., .F.,
 ( 2, 2 ),
 ( 4, 2, 2, 2, 2, 2, 2, 2, 2, 4 ),
 ( 0.000000000000000000, 1.000000000000000000 ),
 ( -4.253008135335690669E-05, 0.0006545663507244089139, 0.001351662782802174646, 0.002048759214879940487, 0.002745855646957706328, 0.004140048511113238010, 0.005534241375268769692, 0.006928434239424301373, 0.008322627103579833055, 0.01111101283189089642 ),
 .UNSPECIFIED. ) ;
#1596=AXIS2_PLACEMENT_3D ( 'NONE', #16018, #10738, #7429 ) ;
#1597=FACE_BOUND ( 'NONE', #3600, .T. ) ;
#1599=ADVANCED_FACE ( 'NONE', ( #16200 ), #5577, .F. ) ;
#1600=CARTESIAN_POINT ( 'NONE',  ( 42.50000000000000711, -9.600000000000001421, -50.00000000000000000 ) ) ;
#1601=AXIS2_PLACEMENT_3D ( 'NONE', #4261, #18232, #2545 ) ;
#1606=AXIS2_PLACEMENT_3D ( 'NONE', #13672, #20241, #16907 ) ;
#1608=VERTEX_POINT ( 'NONE', #17818 ) ;
#1609=VECTOR ( 'NONE', #8019, 1000.000000000000000 ) ;
#1610=EDGE_CURVE ( 'NONE', #18860, #9318, #823, .T. ) ;
#1620=ORIENTED_EDGE ( 'NONE', *, *, #6633, .F. ) ;
#1622=CARTESIAN_POINT ( 'NONE',  ( -10.43027093729826227, 39.22757009021512431, 54.80615623442511009 ) ) ;
#1623=ORIENTED_EDGE ( 'NONE', *, *, #10554, .F. ) ;
#1627=CARTESIAN_POINT ( 'NONE',  ( 35.00000000000000000, 25.00000000000000000, -9.000000000000000000 ) ) ;
#1628=CARTESIAN_POINT ( 'NONE',  ( -9.689843208404349539, 39.33333333333335702, -54.54983754392760886 ) ) ;
#1629=ORIENTED_EDGE ( 'NONE', *, *, #17873, .F. ) ;
#1630=LINE ( 'NONE', #18937, #3903 ) ;
#1633=EDGE_CURVE ( 'NONE', #1608, #11692, #15808, .T. ) ;
#1634=CARTESIAN_POINT ( 'NONE',  ( -16.84758200736127165, 5.154512310753007753, 57.18908790048120494 ) ) ;
#1635=ORIENTED_EDGE ( 'NONE', *, *, #21786, .T. ) ;
#1636=DIRECTION ( 'NONE',  ( -0.000000000000000000, -0.000000000000000000, 1.000000000000000000 ) ) ;
#1639=CIRCLE ( 'NONE', #14415, 8.999999999999966249 ) ;
#1640=ADVANCED_FACE ( 'NONE', ( #9117 ), #4496, .F. ) ;
#1645=ORIENTED_EDGE ( 'NONE', *, *, #22450, .F. ) ;
#1647=ORIENTED_EDGE ( 'NONE', *, *, #15067, .T. ) ;
#1648=CARTESIAN_POINT ( 'NONE',  ( 0.000000000000000000, 0.000000000000000000, 0.000000000000000000 ) ) ;
#1651=AXIS2_PLACEMENT_3D ( 'NONE', #3074, #22337, #8228 ) ;
#1654=CARTESIAN_POINT ( 'NONE',  ( 5.967611645685026112, 40.00000000000000000, 52.07955725514904088 ) ) ;
#1655=ORIENTED_EDGE ( 'NONE', *, *, #6446, .F. ) ;
#1662=PLANE ( 'NONE',  #19986 ) ;
#1665=CARTESIAN_POINT ( 'NONE',  ( -0.9019241164162912217, 39.99518131173311986, 49.42300732039321076 ) ) ;
#1666=DIRECTION ( 'NONE',  ( 0.000000000000000000, 0.000000000000000000, -1.000000000000000000 ) ) ;
#1667=CARTESIAN_POINT ( 'NONE',  ( -13.00000000000011546, 42.51666049839536043, -105.0010000000000048 ) ) ;
#1668=EDGE_CURVE ( 'NONE', #19116, #11797, #16440, .T. ) ;
#1669=CIRCLE ( 'NONE', #3863, 60.00000000000000000 ) ;
#1677=CARTESIAN_POINT ( 'NONE',  ( -35.00000000000058265, 26.00000000000000355, -55.00000000000076028 ) ) ;
#1680=DIRECTION ( 'NONE',  ( -0.000000000000000000, -1.000000000000000000, -0.000000000000000000 ) ) ;
#1683=CARTESIAN_POINT ( 'NONE',  ( 0.5415566900166211006, 39.99826507346841709, 49.15084922740629736 ) ) ;
#1687=CARTESIAN_POINT ( 'NONE',  ( -6.975411493712906363, 39.99999999999999289, -52.53649954156576740 ) ) ;
#1690=ADVANCED_FACE ( 'NONE', ( #7733 ), #5670, .T. ) ;
#1694=ORIENTED_EDGE ( 'NONE', *, *, #22279, .T. ) ;
#1695=FACE_BOUND ( 'NONE', #20390, .T. ) ;
#1699=CARTESIAN_POINT ( 'NONE',  ( 42.50000000000000711, -12.00000000000000000, -47.50000000000000000 ) ) ;
#1700=VERTEX_POINT ( 'NONE', #2008 ) ;
#1701=AXIS2_PLACEMENT_3D ( 'NONE', #19714, #14292, #10986 ) ;
#1702=VERTEX_POINT ( 'NONE', #285 ) ;
#1705=CARTESIAN_POINT ( 'NONE',  ( 1.522021317812884300, -4.618502324868824616, -46.61386490714788522 ) ) ;
#1706=CARTESIAN_POINT ( 'NONE',  ( 11.77933723464115445, 40.00000000000000000, -54.24924979334851116 ) ) ;
#1712=CARTESIAN_POINT ( 'NONE',  ( -17.18568680885986666, 30.37812028685642218, -59.88587632368449221 ) ) ;
#1718=DIRECTION ( 'NONE',  ( -0.000000000000000000, 1.000000000000000000, -0.000000000000000000 ) ) ;
#1719=LINE ( 'NONE', #21188, #13756 ) ;
#1722=CARTESIAN_POINT ( 'NONE',  ( 35.00000000000000000, 2.142135623730931471, 4.258610482196280173E-15 ) ) ;
#1723=CARTESIAN_POINT ( 'NONE',  ( -42.50000000000000711, -12.00000000000012434, -44.97499999999988773 ) ) ;
#1726=ORIENTED_EDGE ( 'NONE', *, *, #10016, .F. ) ;
#1730=DIRECTION ( 'NONE',  ( 0.000000000000000000, 1.000000000000000000, 0.000000000000000000 ) ) ;
#1731=CARTESIAN_POINT ( 'NONE',  ( 8.349099696861289388, 1.803277857259551364, -53.93591755799868537 ) ) ;
#1732=AXIS2_PLACEMENT_3D ( 'NONE', #22641, #3717, #20676 ) ;
#1736=VECTOR ( 'NONE', #9880, 1000.000000000000000 ) ;
#1739=CARTESIAN_POINT ( 'NONE',  ( -11.03199507241031618, 40.00000000000000000, -53.98106524768372338 ) ) ;
#1740=ORIENTED_EDGE ( 'NONE', *, *, #9652, .F. ) ;
#1743=CARTESIAN_POINT ( 'NONE',  ( 20.15166188517204304, 29.89072699358925433, -58.13409936646343823 ) ) ;
#1746=CARTESIAN_POINT ( 'NONE',  ( -6.631891324090021023, 39.71688158846335881, -53.15285336691422202 ) ) ;
#1750=DIRECTION ( 'NONE',  ( 1.049727191138618326E-16, -0.5150380749100547106, 0.8571673007021120005 ) ) ;
#1751=VERTEX_POINT ( 'NONE', #11392 ) ;
#1752=CARTESIAN_POINT ( 'NONE',  ( 11.68987541775893391, 3.735186999536483921, 55.40064774187846552 ) ) ;
#1753=VECTOR ( 'NONE', #17415, 1000.000000000000000 ) ;
#1758=ADVANCED_FACE ( 'NONE', ( #2585 ), #3762, .F. ) ;
#1765=EDGE_CURVE ( 'NONE', #17743, #6038, #8882, .T. ) ;
#1770=CARTESIAN_POINT ( 'NONE',  ( 2.274190170887435691, 40.00000000000000000, 50.13372671147816106 ) ) ;
#1771=AXIS2_PLACEMENT_3D ( 'NONE', #8287, #15255, #22277 ) ;
#1772=ORIENTED_EDGE ( 'NONE', *, *, #12359, .F. ) ;
#1774=CARTESIAN_POINT ( 'NONE',  ( -1.522021317825201336, -4.618502324872293840, -46.61386490715217690 ) ) ;
#1777=CIRCLE ( 'NONE', #12365, 2.099999999999997868 ) ;
#1782=AXIS2_PLACEMENT_3D ( 'NONE', #12775, #6026, #14609 ) ;
#1785=AXIS2_PLACEMENT_3D ( 'NONE', #18466, #4737, #18248 ) ;
#1786=CARTESIAN_POINT ( 'NONE',  ( -4.586067100669611207, 39.86904425122069995, 51.95541839444461374 ) ) ;
#1787=CARTESIAN_POINT ( 'NONE',  ( 22.29034605647553136, 17.39518641927312714, 58.63862881473038158 ) ) ;
#1792=ORIENTED_EDGE ( 'NONE', *, *, #7408, .T. ) ;
#1794=VERTEX_POINT ( 'NONE', #6132 ) ;
#1796=ORIENTED_EDGE ( 'NONE', *, *, #2744, .F. ) ;
#1801=CARTESIAN_POINT ( 'NONE',  ( 0.05198799887590952601, 39.99998426521146655, 48.77440217005271705 ) ) ;
#1802=EDGE_CURVE ( 'NONE', #7505, #5679, #9677, .T. ) ;
#1804=CIRCLE ( 'NONE', #9122, 2.499999999999998668 ) ;
#1806=DIRECTION ( 'NONE',  ( -0.000000000000000000, 1.000000000000000000, -0.000000000000000000 ) ) ;
#1807=DIRECTION ( 'NONE',  ( 0.000000000000000000, 0.000000000000000000, -1.000000000000000000 ) ) ;
#1815=CARTESIAN_POINT ( 'NONE',  ( -1.387778780781445518E-14, 20.00000000000000355, -105.0000000000000142 ) ) ;
#1816=B_SPLINE_CURVE_WITH_KNOTS ( 'NONE', 3,
 ( #7333, #10873, #9054, #14418, #7217, #2178 ),
 .UNSPECIFIED., .F., .F.,
 ( 4, 2, 4 ),
 ( 1.845645724737087379E-18, 0.002694896630591183447, 0.005389793261182365160 ),
 .UNSPECIFIED. ) ;
#1818=EDGE_LOOP ( 'NONE', ( #1300, #6762, #10355, #11585 ) ) ;
#1825=( BOUNDED_SURFACE ( )  B_SPLINE_SURFACE ( 3, 2, ( 
 ( #151, #4068, #9325 ),
 ( #14693, #8066, #1077 ),
 ( #21937, #19869, #4291 ),
 ( #2457, #16302, #4404 ),
 ( #11263, #9551, #21701 ),
 ( #6231, #13191, #4172 ),
 ( #19762, #9443, #615 ),
 ( #21470, #12751, #7719 ),
 ( #11148, #16536, #14802 ),
 ( #11035, #839, #19982 ),
 ( #7950, #18142, #5889 ),
 ( #12857, #7829, #20098 ),
 ( #16423, #21817, #738 ),
 ( #5998, #6116, #13079 ) ),
 .UNSPECIFIED., .F., .F., .F. ) 
 B_SPLINE_SURFACE_WITH_KNOTS ( ( 4, 2, 2, 2, 2, 2, 4 ),
 ( 3, 3 ),
 ( 0.004259382447192771454, 0.005809352080732710713, 0.007359321714272649105, 0.008909291347812587497, 0.01045926098135252676, 0.01355920024843240354, 0.01665913951551228206 ),
 ( 0.000000000000000000, 0.8363185636274830248 ),
 .UNSPECIFIED. ) 
 GEOMETRIC_REPRESENTATION_ITEM ( )  RATIONAL_B_SPLINE_SURFACE ( (
 ( 1.000000000000000000, 0.7012747261256253584, 0.9022084361829376675),
 ( 1.000000000000000000, 0.7322972190981885676, 0.9123640486021487028),
 ( 1.000000000000000000, 0.7591999772719525419, 0.9211710128026768807),
 ( 1.000000000000000000, 0.8072870422117247591, 0.9369129325232377070),
 ( 1.000000000000000000, 0.8284615345039458845, 0.9438446751489368847),
 ( 1.000000000000000000, 0.8663823161282082630, 0.9562585311581923708),
 ( 1.000000000000000000, 0.8831521068476495540, 0.9617483380234417290),
 ( 1.000000000000000000, 0.9127686518824577044, 0.9714436952868192865),
 ( 1.000000000000000000, 0.9255811113611541741, 0.9756380188286946087),
 ( 1.000000000000000000, 0.9589863376200309375, 0.9865736496614985196),
 ( 1.000000000000000000, 0.9746016745770703649, 0.9916855312266366074),
 ( 1.000000000000000000, 0.9951270285874161958, 0.9984047700795721791),
 ( 1.000000000000000000, 0.9999818007053916658, 0.9999940422266351270),
 ( 1.000000000000000000, 1.000000000000000000, 1.000000000000000000) ) ) 
 REPRESENTATION_ITEM ( '' )  SURFACE ( )  );
#1828=CARTESIAN_POINT ( 'NONE',  ( -10.55176496409658604, 37.02956028564889124, -54.80914071361400630 ) ) ;
#1831=ORIENTED_EDGE ( 'NONE', *, *, #22079, .F. ) ;
#1834=FACE_OUTER_BOUND ( 'NONE', #6477, .T. ) ;
#1836=ORIENTED_EDGE ( 'NONE', *, *, #8521, .F. ) ;
#1838=CARTESIAN_POINT ( 'NONE',  ( -35.00000000000000000, -9.000000000000001776, 14.00000000000001421 ) ) ;
#1840=EDGE_LOOP ( 'NONE', ( #9020, #7436, #19859 ) ) ;
#1845=FACE_OUTER_BOUND ( 'NONE', #19525, .T. ) ;
#1847=CARTESIAN_POINT ( 'NONE',  ( 25.99999999999998579, 19.99999999999999645, 105.0000000000000142 ) ) ;
#1848=ORIENTED_EDGE ( 'NONE', *, *, #7591, .T. ) ;
#1850=CARTESIAN_POINT ( 'NONE',  ( 42.50000000000000711, -9.600000000000001421, -49.60000000000000142 ) ) ;
#1851=ORIENTED_EDGE ( 'NONE', *, *, #3289, .F. ) ;
#1855=AXIS2_PLACEMENT_3D ( 'NONE', #2978, #3205, #13487 ) ;
#1856=CARTESIAN_POINT ( 'NONE',  ( -4.996179737156035472, 39.84467275235065387, -52.21079479358778741 ) ) ;
#1859=CARTESIAN_POINT ( 'NONE',  ( -20.34735785252017237, 29.47800210776924601, 58.18363580933387880 ) ) ;
#1860=CARTESIAN_POINT ( 'NONE',  ( 11.00126833624750766, 3.276569432396202242, 57.62199738689401585 ) ) ;
#1862=CARTESIAN_POINT ( 'NONE',  ( -34.99999999999980815, 40.00000000000000000, 54.99999999999922551 ) ) ;
#1864=AXIS2_PLACEMENT_3D ( 'NONE', #7257, #15830, #142 ) ;
#1868=ORIENTED_EDGE ( 'NONE', *, *, #15920, .F. ) ;
#1870=ORIENTED_EDGE ( 'NONE', *, *, #10684, .F. ) ;
#1872=CARTESIAN_POINT ( 'NONE',  ( 18.49252681899428197, 7.260825773989753706, 57.68517796515787666 ) ) ;
#1873=CARTESIAN_POINT ( 'NONE',  ( 9.505538832396775106, 39.99999999999999289, -53.50900172497617291 ) ) ;
#1874=CARTESIAN_POINT ( 'NONE',  ( 7.313763269676020862, 40.00000000000000711, 52.68151666842681635 ) ) ;
#1876=CARTESIAN_POINT ( 'NONE',  ( -35.00000000000000000, 39.00000000000000711, 1.387778780781445676E-14 ) ) ;
#1877=CARTESIAN_POINT ( 'NONE',  ( -0.7217013448959017641, -4.626342591392887726, -46.01887142923196450 ) ) ;
#1879=CYLINDRICAL_SURFACE ( 'NONE', #4631, 2.099999999999997868 ) ;
#1881=DIRECTION ( 'NONE',  ( -0.000000000000000000, -1.000000000000000000, -0.000000000000000000 ) ) ;
#1884=CARTESIAN_POINT ( 'NONE',  ( -90.00000000000000000, 28.00000000000000000, -2.500000000000003109 ) ) ;
#1887=DIRECTION ( 'NONE',  ( -0.000000000000000000, -1.000000000000000000, -0.000000000000000000 ) ) ;
#1888=CARTESIAN_POINT ( 'NONE',  ( -3.946564738182986698, 39.90443716068799063, 51.55060801955053762 ) ) ;
#1889=CARTESIAN_POINT ( 'NONE',  ( 19.42347305479415454, 31.41593231561366650, 57.95407386126545646 ) ) ;
#1890=CARTESIAN_POINT ( 'NONE',  ( 42.50000000000000711, -12.00000000000012434, -44.97499999999988773 ) ) ;
#1893=DIRECTION ( 'NONE',  ( 0.000000000000000000, 0.000000000000000000, 1.000000000000000000 ) ) ;
#1894=VERTEX_POINT ( 'NONE', #10114 ) ;
#1896=ORIENTED_EDGE ( 'NONE', *, *, #13510, .T. ) ;
#1897=EDGE_CURVE ( 'NONE', #16909, #2243, #3406, .T. ) ;
#1903=DIRECTION ( 'NONE',  ( 8.659560562354932858E-17, 0.7071067811865474617, -0.7071067811865474617 ) ) ;
#1904=CARTESIAN_POINT ( 'NONE',  ( 6.264962364260838967, 39.74816733111172340, 52.94809029108233744 ) ) ;
#1906=EDGE_LOOP ( 'NONE', ( #11289, #11944, #13198, #17080 ) ) ;
#1910=DIRECTION ( 'NONE',  ( 0.000000000000000000, 1.000000000000000000, 0.000000000000000000 ) ) ;
#1913=CARTESIAN_POINT ( 'NONE',  ( -42.50000000000000711, -12.00000000000000000, 45.00000000000000711 ) ) ;
#1920=ORIENTED_EDGE ( 'NONE', *, *, #1155, .F. ) ;
#1922=CARTESIAN_POINT ( 'NONE',  ( 7.682546357471700560, -2.941798577943465443, -52.37062424970318375 ) ) ;
#1924=CARTESIAN_POINT ( 'NONE',  ( 12.01755860117725661, 39.99999999999998579, -54.34185968360765173 ) ) ;
#1925=AXIS2_PLACEMENT_3D ( 'NONE', #4573, #11549, #2853 ) ;
#1927=CARTESIAN_POINT ( 'NONE',  ( 35.00000000000000000, -9.000000000000001776, 9.000000000000007105 ) ) ;
#1928=CARTESIAN_POINT ( 'NONE',  ( -19.04641992693179020, 13.69305383064222781, 60.38882653684734692 ) ) ;
#1933=FACE_OUTER_BOUND ( 'NONE', #18238, .T. ) ;
#1939=CARTESIAN_POINT ( 'NONE',  ( -34.99999999999980815, 39.97500000000000142, 57.49999999999921840 ) ) ;
#1940=AXIS2_PLACEMENT_3D ( 'NONE', #21222, #19502, #19846 ) ;
#1941=EDGE_CURVE ( 'NONE', #16162, #12420, #4452, .T. ) ;
#1943=ADVANCED_FACE ( 'NONE', ( #2316 ), #479, .F. ) ;
#1948=CARTESIAN_POINT ( 'NONE',  ( -8.215393105055655454, 1.749144060402859857, 56.08634520686069180 ) ) ;
#1950=ORIENTED_EDGE ( 'NONE', *, *, #10208, .F. ) ;
#1953=CARTESIAN_POINT ( 'NONE',  ( -7.349635197212319504, 40.00000000000000000, 52.69668167434164729 ) ) ;
#1954=EDGE_LOOP ( 'NONE', ( #15619, #232 ) ) ;
#1955=FACE_OUTER_BOUND ( 'NONE', #1270, .T. ) ;
#1956=AXIS2_PLACEMENT_3D ( 'NONE', #9749, #21909, #4488 ) ;
#1961=ORIENTED_EDGE ( 'NONE', *, *, #21275, .T. ) ;
#1962=DIRECTION ( 'NONE',  ( 0.000000000000000000, 0.000000000000000000, 1.000000000000000000 ) ) ;
#1963=CARTESIAN_POINT ( 'NONE',  ( -12.27586057105632378, 4.193657236093761398, 55.54740530681011990 ) ) ;
#1964=CARTESIAN_POINT ( 'NONE',  ( -8.230913598554863597, 39.55470085923248291, -53.98103024247675563 ) ) ;
#1965=ORIENTED_EDGE ( 'NONE', *, *, #9711, .F. ) ;
#1966=ADVANCED_FACE ( 'NONE', ( #10780 ), #2206, .F. ) ;
#1969=FACE_OUTER_BOUND ( 'NONE', #15934, .T. ) ;
#1973=ORIENTED_EDGE ( 'NONE', *, *, #11285, .F. ) ;
#1975=ORIENTED_EDGE ( 'NONE', *, *, #2118, .T. ) ;
#1977=EDGE_LOOP ( 'NONE', ( #11008, #9081 ) ) ;
#1980=CARTESIAN_POINT ( 'NONE',  ( 6.629170412548176294, 39.71713055914890589, -53.15137697417961959 ) ) ;
#1981=CARTESIAN_POINT ( 'NONE',  ( 5.030996208853185436, 39.99999999999998579, 51.62610378409378598 ) ) ;
#1982=EDGE_LOOP ( 'NONE', ( #8822, #16245, #2807, #12860 ) ) ;
#1984=CARTESIAN_POINT ( 'NONE',  ( 0.1963897509099326311, -3.154216256267534213, -47.17168727993868060 ) ) ;
#1988=CARTESIAN_POINT ( 'NONE',  ( -4.295527433237782828E-15, -1.236374842841486021, 48.24164917503448180 ) ) ;
#1990=CARTESIAN_POINT ( 'NONE',  ( 15.49999999999993783, 42.51666049839543149, -105.0010000000000048 ) ) ;
#1992=CARTESIAN_POINT ( 'NONE',  ( 6.696867368502865039E-15, 35.00000000000000000, 38.73397172404480671 ) ) ;
#1995=CARTESIAN_POINT ( 'NONE',  ( -4.240361389880785481, 39.54844917561619866, 53.29842195655543691 ) ) ;
#1996=DIRECTION ( 'NONE',  ( -0.000000000000000000, -0.000000000000000000, -1.000000000000000000 ) ) ;
#1998=CARTESIAN_POINT ( 'NONE',  ( 35.00000000000000000, -5.000000000000000000, 4.258610482196280173E-15 ) ) ;
#2000=CARTESIAN_POINT ( 'NONE',  ( 15.06716847275090387, 33.15945890355548897, 59.19951139074275659 ) ) ;
#2004=VERTEX_POINT ( 'NONE', #12399 ) ;
#2008=CARTESIAN_POINT ( 'NONE',  ( -16.00000000000000000, 20.00000000000000000, -102.0000000000000142 ) ) ;
#2010=CARTESIAN_POINT ( 'NONE',  ( 35.00000000000000000, 39.00000000000000711, 49.99999999999999289 ) ) ;
#2011=CARTESIAN_POINT ( 'NONE',  ( 34.99999999999980815, 40.00000000000000000, 52.89999999999922409 ) ) ;
#2012=CARTESIAN_POINT ( 'NONE',  ( 0.03962180513328213832, 39.99999108785333135, 48.76479353913838821 ) ) ;
#2018=CARTESIAN_POINT ( 'NONE',  ( -9.519381208426278107, 40.00000000000000711, -53.51361895679583114 ) ) ;
#2020=DIRECTION ( 'NONE',  ( -0.000000000000000000, -0.000000000000000000, 1.000000000000000000 ) ) ;
#2025=EDGE_LOOP ( 'NONE', ( #5795, #20438, #16358, #11845 ) ) ;
#2026=CONICAL_SURFACE ( 'NONE', #12259, 2.099999999999997868, 1.029744258676653867 ) ;
#2029=VECTOR ( 'NONE', #19162, 1000.000000000000000 ) ;
#2035=EDGE_CURVE ( 'NONE', #15147, #2703, #10661, .T. ) ;
#2037=DIRECTION ( 'NONE',  ( 0.000000000000000000, 0.000000000000000000, 1.000000000000000000 ) ) ;
#2040=CIRCLE ( 'NONE', #11912, 49.99999999999998579 ) ;
#2041=CARTESIAN_POINT ( 'NONE',  ( -9.870870746768591886, 37.43479630316498685, -54.49920060631094998 ) ) ;
#2045=CARTESIAN_POINT ( 'NONE',  ( -35.00000000000000000, 40.00000000000000000, 1.387778780781445676E-14 ) ) ;
#2047=EDGE_CURVE ( 'NONE', #10753, #19175, #253, .T. ) ;
#2048=DIRECTION ( 'NONE',  ( -0.000000000000000000, 1.000000000000000000, -0.000000000000000000 ) ) ;
#2049=DIRECTION ( 'NONE',  ( 0.000000000000000000, 0.000000000000000000, -1.000000000000000000 ) ) ;
#2050=AXIS2_PLACEMENT_3D ( 'NONE', #678, #5942, #19926 ) ;
#2053=DIRECTION ( 'NONE',  ( 0.000000000000000000, 0.000000000000000000, -1.000000000000000000 ) ) ;
#2056=EDGE_LOOP ( 'NONE', ( #9955, #14243, #15268, #21628 ) ) ;
#2057=VECTOR ( 'NONE', #18363, 1000.000000000000000 ) ;
#2058=AXIS2_PLACEMENT_3D ( 'NONE', #10921, #17579, #5539 ) ;
#2067=CARTESIAN_POINT ( 'NONE',  ( -6.816848327306503030, 40.00000000000000000, 52.46798795272709981 ) ) ;
#2071=DIRECTION ( 'NONE',  ( 0.000000000000000000, 0.000000000000000000, 1.000000000000000000 ) ) ;
#2072=EDGE_CURVE ( 'NONE', #22642, #15602, #17239, .T. ) ;
#2077=CARTESIAN_POINT ( 'NONE',  ( -2.229105529478774717, 39.97007248092597820, -50.38830888536040931 ) ) ;
#2084=AXIS2_PLACEMENT_3D ( 'NONE', #14630, #21635, #4220 ) ;
#2091=CARTESIAN_POINT ( 'NONE',  ( 13.00000000000024336, -2.516660498395250745, -105.0010000000000048 ) ) ;
#2097=FACE_OUTER_BOUND ( 'NONE', #3973, .T. ) ;
#2098=ORIENTED_EDGE ( 'NONE', *, *, #15554, .T. ) ;
#2103=FACE_OUTER_BOUND ( 'NONE', #18603, .T. ) ;
#2107=DIRECTION ( 'NONE',  ( 0.000000000000000000, 0.000000000000000000, -1.000000000000000000 ) ) ;
#2112=CIRCLE ( 'NONE', #14887, 10.00000000000000178 ) ;
#2114=CARTESIAN_POINT ( 'NONE',  ( 19.23106185100178323, 25.51013774189591388, 60.43438466297350686 ) ) ;
#2115=CARTESIAN_POINT ( 'NONE',  ( -35.00000000000058265, 39.97500000000000142, -57.50000000000076028 ) ) ;
#2116=AXIS2_PLACEMENT_3D ( 'NONE', #4212, #18990, #17023 ) ;
#2117=CARTESIAN_POINT ( 'NONE',  ( 10.58465497538991507, 37.06540556996028357, -54.84139108225040360 ) ) ;
#2118=EDGE_CURVE ( 'NONE', #11218, #2374, #12851, .T. ) ;
#2120=VERTEX_POINT ( 'NONE', #371 ) ;
#2121=VECTOR ( 'NONE', #1376, 1000.000000000000114 ) ;
#2122=EDGE_LOOP ( 'NONE', ( #20601, #21676 ) ) ;
#2125=EDGE_CURVE ( 'NONE', #14214, #22156, #21717, .T. ) ;
#2126=CIRCLE ( 'NONE', #14914, 2.500000000000002220 ) ;
#2128=EDGE_CURVE ( 'NONE', #3791, #5986, #11323, .T. ) ;
#2129=AXIS2_PLACEMENT_3D ( 'NONE', #20168, #18557, #11570 ) ;
#2131=AXIS2_PLACEMENT_3D ( 'NONE', #10243, #4658, #1100 ) ;
#2134=VECTOR ( 'NONE', #21153, 1000.000000000000000 ) ;
#2135=ORIENTED_EDGE ( 'NONE', *, *, #17290, .T. ) ;
#2144=VECTOR ( 'NONE', #11426, 1000.000000000000000 ) ;
#2147=FACE_OUTER_BOUND ( 'NONE', #10095, .T. ) ;
#2148=EDGE_CURVE ( 'NONE', #3138, #18756, #4223, .T. ) ;
#2149=VECTOR ( 'NONE', #10534, 1000.000000000000000 ) ;
#2150=ORIENTED_EDGE ( 'NONE', *, *, #12686, .F. ) ;
#2152=ORIENTED_EDGE ( 'NONE', *, *, #13561, .T. ) ;
#2153=ADVANCED_FACE ( 'NONE', ( #9642, #16632 ), #22255, .F. ) ;
#2159=DIRECTION ( 'NONE',  ( -0.000000000000000000, -1.000000000000000000, -0.000000000000000000 ) ) ;
#2161=CARTESIAN_POINT ( 'NONE',  ( -15.89815672374914080, 32.14246426897781816, -59.47617874060593124 ) ) ;
#2165=LINE ( 'NONE', #17398, #16809 ) ;
#2167=CARTESIAN_POINT ( 'NONE',  ( 10.63866000424712688, 9.419394561690120682, -43.66469350997162024 ) ) ;
#2172=ADVANCED_FACE ( 'NONE', ( #9969 ), #17298, .T. ) ;
#2178=CARTESIAN_POINT ( 'NONE',  ( -13.56354382738803466, 2.142135623730931471, 56.03997097393687454 ) ) ;
#2179=B_SPLINE_CURVE_WITH_KNOTS ( 'NONE', 3,
 ( #22425, #11757, #13685, #3297, #8215, #20700, #6607, #13571, #998, #1115, #11537, #1335, #11868, #18526, #11991, #20253, #18991 ),
 .UNSPECIFIED., .F., .F.,
 ( 4, 1, 1, 2, 2, 1, 1, 1, 2, 2, 4 ),
 ( 0.000000000000000000, 0.1250000000000117129, 0.1875000000000175693, 0.2187500000000204836, 0.2500000000000234257, 0.3750000000000403566, 0.4375000000000473510, 0.4687500000000494049, 0.4843750000000508482, 0.5000000000000522915, 1.000000000000000000 ),
 .UNSPECIFIED. ) ;
#2180=DIRECTION ( 'NONE',  ( -0.000000000000000000, -0.000000000000000000, 1.000000000000000000 ) ) ;
#2183=CARTESIAN_POINT ( 'NONE',  ( -5.553309044144580042, 39.99999999999999289, 51.88330199943927568 ) ) ;
#2184=ORIENTED_EDGE ( 'NONE', *, *, #15752, .F. ) ;
#2186=DIRECTION ( 'NONE',  ( 0.000000000000000000, -1.000000000000000000, 0.000000000000000000 ) ) ;
#2191=DIRECTION ( 'NONE',  ( -0.000000000000000000, -0.000000000000000000, 1.000000000000000000 ) ) ;
#2193=CARTESIAN_POINT ( 'NONE',  ( -6.692425220448997791, 39.70962082156066231, -53.18141015372126645 ) ) ;
#2195=CONICAL_SURFACE ( 'NONE', #21971, 15.00000000000000000, 0.7853981633974552734 ) ;
#2196=DIRECTION ( 'NONE',  ( -0.000000000000000000, 1.000000000000000000, -0.000000000000000000 ) ) ;
#2197=CARTESIAN_POINT ( 'NONE',  ( 35.00000000000058265, 26.00000000000000355, -52.90000000000076597 ) ) ;
#2201=EDGE_CURVE ( 'NONE', #11720, #12153, #8, .T. ) ;
#2203=ORIENTED_EDGE ( 'NONE', *, *, #13624, .F. ) ;
#2206=CYLINDRICAL_SURFACE ( 'NONE', #56, 2.499999999999998668 ) ;
#2209=CARTESIAN_POINT ( 'NONE',  ( 9.225361348764007374, 39.40776743449596609, -54.37884520109041375 ) ) ;
#2211=EDGE_CURVE ( 'NONE', #9264, #10753, #8115, .T. ) ;
#2212=EDGE_LOOP ( 'NONE', ( #18111, #16152 ) ) ;
#2216=CARTESIAN_POINT ( 'NONE',  ( 35.00000000000058265, 40.00000000000000711, -55.00000000000076028 ) ) ;
#2217=CARTESIAN_POINT ( 'NONE',  ( -11.86180952233172725, 39.00000000000000000, -55.35904751184885697 ) ) ;
#2218=DIRECTION ( 'NONE',  ( -0.000000000000000000, -1.000000000000000000, -0.000000000000000000 ) ) ;
#2219=ORIENTED_EDGE ( 'NONE', *, *, #19831, .T. ) ;
#2220=DIRECTION ( 'NONE',  ( -0.000000000000000000, 1.000000000000000000, -0.000000000000000000 ) ) ;
#2223=CARTESIAN_POINT ( 'NONE',  ( 6.696867368502865039E-15, 35.00000000000000000, 38.73397172404480671 ) ) ;
#2224=CARTESIAN_POINT ( 'NONE',  ( -42.50000000000000711, -11.97499999999999964, 50.00000000000000711 ) ) ;
#2225=EDGE_LOOP ( 'NONE', ( #19995, #18967 ) ) ;
#2227=CARTESIAN_POINT ( 'NONE',  ( 20.31722544680816256, 29.72987180553230502, 58.17992760854182421 ) ) ;
#2230=CARTESIAN_POINT ( 'NONE',  ( -35.00000000000000000, 39.00000000000000711, 1.387778780781445676E-14 ) ) ;
#2231=ORIENTED_EDGE ( 'NONE', *, *, #5568, .F. ) ;
#2232=EDGE_CURVE ( 'NONE', #19255, #15800, #10651, .T. ) ;
#2233=ORIENTED_EDGE ( 'NONE', *, *, #17462, .T. ) ;
#2235=ORIENTED_EDGE ( 'NONE', *, *, #4469, .F. ) ;
#2238=LINE ( 'NONE', #2010, #14014 ) ;
#2243=VERTEX_POINT ( 'NONE', #19038 ) ;
#2249=EDGE_CURVE ( 'NONE', #21816, #7482, #4094, .T. ) ;
#2251=ADVANCED_FACE ( 'NONE', ( #20753 ), #9578, .F. ) ;
#2255=CARTESIAN_POINT ( 'NONE',  ( 35.00000000000000000, -9.000000000000001776, 18.00000000000000711 ) ) ;
#2258=ORIENTED_EDGE ( 'NONE', *, *, #2366, .F. ) ;
#2260=CARTESIAN_POINT ( 'NONE',  ( -6.262904276180248253, 0.9586397763588609955, -54.84547588849994781 ) ) ;
#2262=VECTOR ( 'NONE', #14767, 1000.000000000000000 ) ;
#2265=CARTESIAN_POINT ( 'NONE',  ( -19.80871821058217108, 17.21148610482000763, 60.57629886234796857 ) ) ;
#2267=CARTESIAN_POINT ( 'NONE',  ( -12.26943921815750116, 35.80002840870906766, -58.15275698935778337 ) ) ;
#2269=ORIENTED_EDGE ( 'NONE', *, *, #22339, .F. ) ;
#2274=FACE_OUTER_BOUND ( 'NONE', #4306, .T. ) ;
#2281=AXIS2_PLACEMENT_3D ( 'NONE', #20000, #13098, #16664 ) ;
#2284=ADVANCED_FACE ( 'NONE', ( #18920 ), #10196, .F. ) ;
#2287=FACE_OUTER_BOUND ( 'NONE', #20245, .T. ) ;
#2290=CARTESIAN_POINT ( 'NONE',  ( -12.84899528830096926, 2.142135623730930583, 57.90797000640143466 ) ) ;
#2295=DIRECTION ( 'NONE',  ( 1.000000000000000000, 0.000000000000000000, 0.000000000000000000 ) ) ;
#2297=CARTESIAN_POINT ( 'NONE',  ( 25.99999999999998579, 19.99999999999999645, -100.0000000000000000 ) ) ;
#2299=ORIENTED_EDGE ( 'NONE', *, *, #11532, .F. ) ;
#2301=CARTESIAN_POINT ( 'NONE',  ( -13.56354382738793696, 2.142135623730796468, 56.03997097393716587 ) ) ;
#2302=CARTESIAN_POINT ( 'NONE',  ( -3.069014598162472129, 39.94370170965071765, -50.97148269059585601 ) ) ;
#2305=CARTESIAN_POINT ( 'NONE',  ( 10.62139969368200454, 0.6004703193300734432, 54.70636795414621645 ) ) ;
#2313=CIRCLE ( 'NONE', #15101, 18.00000000000000000 ) ;
#2316=FACE_OUTER_BOUND ( 'NONE', #2660, .T. ) ;
#2319=LINE ( 'NONE', #4389, #6 ) ;
#2324=EDGE_CURVE ( 'NONE', #17065, #6302, #3364, .T. ) ;
#2325=ADVANCED_FACE ( 'NONE', ( #17981 ), #7102, .F. ) ;
#2336=CARTESIAN_POINT ( 'NONE',  ( 3.126261098509322434, 0.2355326842376759267, 52.75562998449589003 ) ) ;
#2338=DIRECTION ( 'NONE',  ( -0.000000000000000000, 1.000000000000000000, -0.000000000000000000 ) ) ;
#2340=CARTESIAN_POINT ( 'NONE',  ( 12.50843255120944875, 35.62740313860285113, 55.64392373821144133 ) ) ;
#2346=EDGE_LOOP ( 'NONE', ( #12465, #20087, #1961, #7729 ) ) ;
#2347=AXIS2_PLACEMENT_3D ( 'NONE', #7152, #8652, #21143 ) ;
#2348=ORIENTED_EDGE ( 'NONE', *, *, #5691, .F. ) ;
#2353=CIRCLE ( 'NONE', #5280, 2.500000000000002220 ) ;
#2355=ORIENTED_EDGE ( 'NONE', *, *, #4969, .F. ) ;
#2361=CARTESIAN_POINT ( 'NONE',  ( -42.50000000000000711, -12.00000000000012434, -44.97499999999988773 ) ) ;
#2363=DIRECTION ( 'NONE',  ( 0.000000000000000000, 0.000000000000000000, -1.000000000000000000 ) ) ;
#2364=CARTESIAN_POINT ( 'NONE',  ( -11.68090480754633731, 3.765577839755393619, -57.90797000640141334 ) ) ;
#2366=EDGE_CURVE ( 'NONE', #19351, #478, #11387, .T. ) ;
#2368=DIRECTION ( 'NONE',  ( 0.000000000000000000, 0.000000000000000000, 1.000000000000000000 ) ) ;
#2372=CARTESIAN_POINT ( 'NONE',  ( 21.99999999999998579, 20.00000000000000000, 100.0000000000000000 ) ) ;
#2374=VERTEX_POINT ( 'NONE', #16605 ) ;
#2375=VERTEX_POINT ( 'NONE', #8023 ) ;
#2379=VECTOR ( 'NONE', #15019, 1000.000000000000114 ) ;
#2381=CARTESIAN_POINT ( 'NONE',  ( 90.00000000000000000, 28.00000000000000000, 2.099999999999989875 ) ) ;
#2382=LINE ( 'NONE', #13688, #15205 ) ;
#2383=CARTESIAN_POINT ( 'NONE',  ( -1.387778780781445518E-14, 20.00000000000000355, 105.0000000000000142 ) ) ;
#2384=CARTESIAN_POINT ( 'NONE',  ( -1.427806064787912943, 39.96253293977173371, -50.08434658998346123 ) ) ;
#2385=DIRECTION ( 'NONE',  ( 0.000000000000000000, 1.000000000000000000, 0.000000000000000000 ) ) ;
#2390=CARTESIAN_POINT ( 'NONE',  ( 42.50000000000000711, -12.00000000000000000, 54.00000000000000711 ) ) ;
#2391=DIRECTION ( 'NONE',  ( 0.000000000000000000, 0.000000000000000000, 1.000000000000000000 ) ) ;
#2397=CARTESIAN_POINT ( 'NONE',  ( 17.99999999999998579, 20.00000000000000711, -102.9999999999999716 ) ) ;
#2398=DIRECTION ( 'NONE',  ( -0.000000000000000000, -1.000000000000000000, -0.000000000000000000 ) ) ;
#2399=DIRECTION ( 'NONE',  ( -1.000000000000000000, 0.000000000000000000, 0.000000000000000000 ) ) ;
#2400=VECTOR ( 'NONE', #18818, 1000.000000000000000 ) ;
#2403=DIRECTION ( 'NONE',  ( 0.000000000000000000, 0.5150380749100562650, 0.8571673007021111124 ) ) ;
#2405=CARTESIAN_POINT ( 'NONE',  ( 3.092931222847586259, 39.99999999999999289, -50.60141000603072570 ) ) ;
#2406=AXIS2_PLACEMENT_3D ( 'NONE', #14824, #16334, #9687 ) ;
#2408=CARTESIAN_POINT ( 'NONE',  ( 0.3010984638803619884, 39.99946791130895463, -48.96692764038679258 ) ) ;
#2409=AXIS2_PLACEMENT_3D ( 'NONE', #5465, #12657, #10951 ) ;
#2410=CARTESIAN_POINT ( 'NONE',  ( 11.87329829275380533, 39.99999999999997868, 54.28004929202755591 ) ) ;
#2411=DIRECTION ( 'NONE',  ( 0.000000000000000000, 1.000000000000000000, 0.000000000000000000 ) ) ;
#2412=ORIENTED_EDGE ( 'NONE', *, *, #13612, .F. ) ;
#2413=CARTESIAN_POINT ( 'NONE',  ( -90.00000000000000000, 40.00000000000000711, 2.524999999999998579 ) ) ;
#2414=CARTESIAN_POINT ( 'NONE',  ( -11.05758567242951607, 3.294696707132223512, -55.18338768060504407 ) ) ;
#2418=CARTESIAN_POINT ( 'NONE',  ( -5.649790292151565474, 40.00000000000000711, 51.93142534747384786 ) ) ;
#2422=FACE_OUTER_BOUND ( 'NONE', #8100, .T. ) ;
#2423=DIRECTION ( 'NONE',  ( -0.000000000000000000, 1.000000000000000000, -0.000000000000000000 ) ) ;
#2425=ORIENTED_EDGE ( 'NONE', *, *, #13673, .F. ) ;
#2426=DIRECTION ( 'NONE',  ( 0.000000000000000000, 0.000000000000000000, 1.000000000000000000 ) ) ;
#2428=CARTESIAN_POINT ( 'NONE',  ( -10.38193264731104648, 30.83255023748043655, 43.52061562521062399 ) ) ;
#2439=ORIENTED_EDGE ( 'NONE', *, *, #14768, .T. ) ;
#2444=CARTESIAN_POINT ( 'NONE',  ( 34.99999999999980815, 28.00000000000000000, 57.49999999999921840 ) ) ;
#2445=CARTESIAN_POINT ( 'NONE',  ( 42.50000000000000711, -12.00000000000012434, 50.02500000000011937 ) ) ;
#2455=LINE ( 'NONE', #736, #7262 ) ;
#2456=ORIENTED_EDGE ( 'NONE', *, *, #21678, .T. ) ;
#2457=CARTESIAN_POINT ( 'NONE',  ( 6.803227178529145824, 38.81166136533732214, 55.43135129401766648 ) ) ;
#2461=ADVANCED_FACE ( 'NONE', ( #22423 ), #685, .F. ) ;
#2462=DIRECTION ( 'NONE',  ( 0.000000000000000000, -0.000000000000000000, 1.000000000000000000 ) ) ;
#2465=AXIS2_PLACEMENT_3D ( 'NONE', #17422, #17, #20762 ) ;
#2466=EDGE_CURVE ( 'NONE', #13970, #20079, #12744, .T. ) ;
#2469=EDGE_LOOP ( 'NONE', ( #13082, #11885 ) ) ;
#2477=VERTEX_POINT ( 'NONE', #10698 ) ;
#2478=DIRECTION ( 'NONE',  ( 0.000000000000000000, 0.000000000000000000, -1.000000000000000000 ) ) ;
#2479=CIRCLE ( 'NONE', #11987, 2.500000000000002220 ) ;
#2480=VERTEX_POINT ( 'NONE', #13683 ) ;
#2481=FACE_OUTER_BOUND ( 'NONE', #14323, .T. ) ;
#2483=CARTESIAN_POINT ( 'NONE',  ( -9.689843208404459673, 39.33333333333334991, -54.54983754392748807 ) ) ;
#2486=CARTESIAN_POINT ( 'NONE',  ( 35.00000000000000000, 25.00000000000000000, 4.258610482196280173E-15 ) ) ;
#2487=DIRECTION ( 'NONE',  ( 0.000000000000000000, 0.5150380749100562650, 0.8571673007021111124 ) ) ;
#2488=DIRECTION ( 'NONE',  ( 9.523972024970703335E-16, 0.000000000000000000, 1.000000000000000000 ) ) ;
#2490=DIRECTION ( 'NONE',  ( -0.4332438415859253822, 0.000000000000000000, 0.9012767464701779696 ) ) ;
#2491=EDGE_LOOP ( 'NONE', ( #16736, #17445, #19403, #21173 ) ) ;
#2493=ORIENTED_EDGE ( 'NONE', *, *, #14262, .T. ) ;
#2495=ADVANCED_FACE ( 'NONE', ( #8663 ), #11827, .T. ) ;
#2496=ORIENTED_EDGE ( 'NONE', *, *, #213, .F. ) ;
#2502=DIRECTION ( 'NONE',  ( 0.000000000000000000, 1.000000000000000000, 0.000000000000000000 ) ) ;
#2504=CARTESIAN_POINT ( 'NONE',  ( 0.7809641287214827976, -4.625293788890135538, 46.06432795380052170 ) ) ;
#2505=CARTESIAN_POINT ( 'NONE',  ( -35.00000000000058265, 40.00000000000000000, -55.00000000000076028 ) ) ;
#2508=VECTOR ( 'NONE', #13892, 1000.000000000000000 ) ;
#2512=CARTESIAN_POINT ( 'NONE',  ( 25.99999999999998579, 19.99999999999999645, -105.0000000000000142 ) ) ;
#2516=CONICAL_SURFACE ( 'NONE', #1785, 2.099999999999997868, 1.029744258676652091 ) ;
#2524=CARTESIAN_POINT ( 'NONE',  ( -42.50000000000000711, -5.000000000000000000, -47.50000000000000000 ) ) ;
#2525=CARTESIAN_POINT ( 'NONE',  ( 7.130216064151039923, 40.00000000000000000, -52.60396709977539587 ) ) ;
#2527=ORIENTED_EDGE ( 'NONE', *, *, #17266, .T. ) ;
#2528=CARTESIAN_POINT ( 'NONE',  ( 3.658198312395513518, 39.91812900842233347, -51.36232427839211567 ) ) ;
#2532=DIRECTION ( 'NONE',  ( -0.000000000000000000, 1.000000000000000000, -0.000000000000000000 ) ) ;
#2533=LINE ( 'NONE', #15094, #14889 ) ;
#2539=DIRECTION ( 'NONE',  ( -0.000000000000000000, -0.000000000000000000, 1.000000000000000000 ) ) ;
#2541=CARTESIAN_POINT ( 'NONE',  ( -1.387778780781445518E-14, 20.00000000000000355, 102.0000000000000142 ) ) ;
#2544=CARTESIAN_POINT ( 'NONE',  ( 8.349099696857495090, 1.803277857257809424, 53.93591755799672427 ) ) ;
#2545=DIRECTION ( 'NONE',  ( -1.000000000000000000, 0.000000000000000000, 0.000000000000000000 ) ) ;
#2550=ORIENTED_EDGE ( 'NONE', *, *, #1258, .T. ) ;
#2552=ORIENTED_EDGE ( 'NONE', *, *, #10261, .T. ) ;
#2556=CARTESIAN_POINT ( 'NONE',  ( 7.480086125706187694, -0.2526605362868768467, 53.02285530597295349 ) ) ;
#2561=DIRECTION ( 'NONE',  ( -0.000000000000000000, -1.000000000000000000, -0.000000000000000000 ) ) ;
#2562=CARTESIAN_POINT ( 'NONE',  ( 6.696867368503558448E-15, 40.00000000000000000, 48.73397172404481381 ) ) ;
#2565=FACE_OUTER_BOUND ( 'NONE', #16556, .T. ) ;
#2566=CARTESIAN_POINT ( 'NONE',  ( 14.04165170564756870, 5.752764646445603702, -58.83649392397241229 ) ) ;
#2567=EDGE_LOOP ( 'NONE', ( #11959, #4394, #19309, #6880 ) ) ;
#2572=DIRECTION ( 'NONE',  ( 0.000000000000000000, 0.000000000000000000, -1.000000000000000000 ) ) ;
#2573=CARTESIAN_POINT ( 'NONE',  ( -8.349099696861340902, 1.803277857259562911, -53.93591755799872800 ) ) ;
#2577=LINE ( 'NONE', #12863, #832 ) ;
#2578=CARTESIAN_POINT ( 'NONE',  ( 11.59291124596733091, 39.24500985575833312, -55.27372209264543557 ) ) ;
#2579=B_SPLINE_CURVE_WITH_KNOTS ( 'NONE', 3,
 ( #2217, #17798, #9094, #3614, #10574, #17572, #19520, #15833, #5430, #12409, #3720, #7260, #3828, #16072, #380, #7373, #5646, #12620, #19639, #3943, #16177, #20092, #11486, #12965, #18473, #19976, #6110, #9771, #731, #7712, #21931, #14577, #4507, #9320, #12850, #11256, #9653, #18254 ),
 .UNSPECIFIED., .F., .F.,
 ( 4, 2, 2, 2, 2, 2, 2, 2, 2, 2, 2, 2, 2, 2, 2, 2, 2, 2, 4 ),
 ( 0.002265996298495699668, 0.003649092030476641657, 0.005032187762457583646, 0.007798379226419466757, 0.01056457069038134813, 0.01333076215434323038, 0.01609695361830511262, 0.01886314508226699313, 0.02439552801019075068, 0.02577862374217168920, 0.02716171947415263466, 0.02992791093811452557, 0.03131100667009547450, 0.03269410240207642343, 0.03546029386603831435, 0.03822648533000020526, 0.03960958106198115419, 0.04099267679396210312, 0.04652505972188589189 ),
 .UNSPECIFIED. ) ;
#2582=VERTEX_POINT ( 'NONE', #16204 ) ;
#2585=FACE_OUTER_BOUND ( 'NONE', #17532, .T. ) ;
#2590=DIRECTION ( 'NONE',  ( 0.000000000000000000, 0.000000000000000000, -1.000000000000000000 ) ) ;
#2591=FACE_OUTER_BOUND ( 'NONE', #7850, .T. ) ;
#2594=CARTESIAN_POINT ( 'NONE',  ( -6.041077103370482426, -0.8288449397156264498, -52.13906252460640900 ) ) ;
#2597=FACE_OUTER_BOUND ( 'NONE', #9543, .T. ) ;
#2599=FACE_OUTER_BOUND ( 'NONE', #1818, .T. ) ;
#2604=ORIENTED_EDGE ( 'NONE', *, *, #20625, .T. ) ;
#2607=EDGE_CURVE ( 'NONE', #14950, #4040, #6765, .T. ) ;
#2609=CARTESIAN_POINT ( 'NONE',  ( -20.32373648405383193, 10.46972314276651872, 58.17772014969900596 ) ) ;
#2617=CARTESIAN_POINT ( 'NONE',  ( -5.833333333333325932, 39.00000000000000711, 40.61164310337068883 ) ) ;
#2618=CARTESIAN_POINT ( 'NONE',  ( -3.499474518498425473E-16, -0.4099377891817043151, 48.99242580662814106 ) ) ;
#2619=CARTESIAN_POINT ( 'NONE',  ( -34.99999999999980815, 26.00000000000000355, 52.89999999999922409 ) ) ;
#2620=CARTESIAN_POINT ( 'NONE',  ( -7.938322399558154885, 38.36220367130613340, -56.16250688146275394 ) ) ;
#2623=CARTESIAN_POINT ( 'NONE',  ( -35.00000000000058265, 40.00000000000000000, -52.90000000000076597 ) ) ;
#2624=CIRCLE ( 'NONE', #1525, 2.099999999999990763 ) ;
#2625=ORIENTED_EDGE ( 'NONE', *, *, #16777, .F. ) ;
#2626=CARTESIAN_POINT ( 'NONE',  ( -35.00000000000000000, 40.00000000000000000, 1.387778780781445676E-14 ) ) ;
#2629=DIRECTION ( 'NONE',  ( 0.000000000000000000, 0.000000000000000000, 1.000000000000000000 ) ) ;
#2633=DIRECTION ( 'NONE',  ( -1.000000000000000000, 0.000000000000000000, 0.000000000000000000 ) ) ;
#2635=DIRECTION ( 'NONE',  ( 0.000000000000000000, 0.000000000000000000, -1.000000000000000000 ) ) ;
#2636=EDGE_CURVE ( 'NONE', #575, #6067, #20441, .T. ) ;
#2638=EDGE_LOOP ( 'NONE', ( #1975, #18570 ) ) ;
#2646=CARTESIAN_POINT ( 'NONE',  ( -12.27586057105639838, 4.193657236093905283, -55.54740530680978594 ) ) ;
#2648=CARTESIAN_POINT ( 'NONE',  ( -90.00000000000000000, 40.00000000000000711, -9.108981535246192915E-16 ) ) ;
#2649=ORIENTED_EDGE ( 'NONE', *, *, #12103, .F. ) ;
#2652=FACE_OUTER_BOUND ( 'NONE', #3675, .T. ) ;
#2654=ORIENTED_EDGE ( 'NONE', *, *, #13007, .T. ) ;
#2655=CARTESIAN_POINT ( 'NONE',  ( 8.923978417719926171, 2.083761144193561066, 56.51262908347950997 ) ) ;
#2660=EDGE_LOOP ( 'NONE', ( #6265, #17790, #11522, #5448 ) ) ;
#2661=ORIENTED_EDGE ( 'NONE', *, *, #17816, .F. ) ;
#2662=B_SPLINE_CURVE_WITH_KNOTS ( 'NONE', 3,
 ( #21325, #21563, #1964, #240, #19842, #19498, #2193, #7459, #10890, #12484, #7119, #17892, #5621, #17998, #12597, #12387, #16049, #3803, #10649, #8948, #9295, #7235, #4143, #11011, #15813, #2302, #21106, #19395, #11119, #2077, #18109, #8838, #3700, #16151, #19611, #123, #14204, #10765, #21216, #14431, #17771, #14316, #464, #585, #14552, #9071, #21440, #358, #7348, #5743, #4043, #16274, #7573, #5862, #20407, #4258, #707, #11691, #15103, #16505, #14994, #11351, #21905, #4375, #6201, #13164, #20067, #812, #18336, #4482, #2881, #1149 ),
 .UNSPECIFIED., .F., .F.,
 ( 4, 2, 1, 2, 2, 1, 1, 2, 2, 2, 2, 1, 1, 1, 1, 1, 2, 2, 2, 1, 1, 1, 1, 1, 2, 2, 1, 1, 1, 1, 2, 2, 1, 1, 2, 2, 1, 2, 2, 2, 1, 1, 2, 2, 2, 2, 4 ),
 ( 0.000000000000000000, 0.2499923706055057759, 0.2812414169311941992, 0.2851475477219057586, 0.2871006131172617604, 0.2890536785126177621, 0.2968659400940392712, 0.3124904632568824558, 0.3749885559082549724, 0.4999847412109998945, 0.5019378066063551191, 0.5038908720017102327, 0.5077970027924207930, 0.5156092643738410253, 0.5312337875366800466, 0.5624828338623590884, 0.6249809265137173941, 0.7499771118164337835, 0.7519301772117895633, 0.7538832426071453430, 0.7577893733978569024, 0.7656016349792786890, 0.7812261581421213741, 0.8124752044678077434, 0.8749732971191792608, 0.8769263625145349295, 0.8788794279098904871, 0.8827855587006018245, 0.8905978202820242773, 0.9062223434448704040, 0.9374713897705615473, 0.9413775205612727737, 0.9452836513519840000, 0.9530959129334075630, 0.9687204360962549110, 0.9726265668869673586, 0.9765326976776796952, 0.9843449592591031472, 0.9921572208405267101, 0.9926454871893649612, 0.9931337535382033233, 0.9941102862358790482, 0.9960633516312306091, 0.9965516179800615326, 0.9970398843288925672, 0.9980164170265533041, 0.9999694824218750000 ),
 .UNSPECIFIED. ) ;
#2665=CARTESIAN_POINT ( 'NONE',  ( 12.24744603029285273, 40.00000000000000000, 54.43639671998466412 ) ) ;
#2667=AXIS2_PLACEMENT_3D ( 'NONE', #10055, #4811, #22578 ) ;
#2668=CONICAL_SURFACE ( 'NONE', #8144, 2.099999999999990763, 1.029744258676652091 ) ;
#2670=CARTESIAN_POINT ( 'NONE',  ( -22.00000000000001421, 20.00000000000000355, 100.0000000000000000 ) ) ;
#2672=ORIENTED_EDGE ( 'NONE', *, *, #10261, .F. ) ;
#2673=FACE_OUTER_BOUND ( 'NONE', #3912, .T. ) ;
#2674=ORIENTED_EDGE ( 'NONE', *, *, #17086, .T. ) ;
#2676=DIRECTION ( 'NONE',  ( 0.000000000000000000, 0.000000000000000000, 1.000000000000000000 ) ) ;
#2678=DIRECTION ( 'NONE',  ( 0.000000000000000000, 0.000000000000000000, 1.000000000000000000 ) ) ;
#2680=FACE_OUTER_BOUND ( 'NONE', #22269, .T. ) ;
#2681=CARTESIAN_POINT ( 'NONE',  ( 5.666031183648402525, 39.18449859167989757, -54.55698311759260122 ) ) ;
#2682=ORIENTED_EDGE ( 'NONE', *, *, #19566, .T. ) ;
#2684=CARTESIAN_POINT ( 'NONE',  ( -3.711215864303547551, -1.139709857517552605, -50.71371062340998037 ) ) ;
#2686=DIRECTION ( 'NONE',  ( 0.000000000000000000, 1.000000000000000000, 0.000000000000000000 ) ) ;
#2690=CARTESIAN_POINT ( 'NONE',  ( 20.11496009237018256, 10.03305173526324445, -58.12476682723747956 ) ) ;
#2699=( BOUNDED_SURFACE ( )  B_SPLINE_SURFACE ( 3, 2, ( 
 ( #20266, #7888, #3390 ),
 ( #4572, #14852, #15188 ),
 ( #4457, #22213, #11547 ),
 ( #9714, #21876, #20806 ),
 ( #10349, #17351, #8650 ),
 ( #15625, #13139, #20153 ),
 ( #10926, #5779, #14349 ),
 ( #10805, #3839, #9210 ),
 ( #21477, #7274, #12756 ),
 ( #15842, #19429, #389 ),
 ( #17810, #19767, #274 ),
 ( #7384, #12518, #1787 ),
 ( #52, #21360, #19315 ),
 ( #10681, #5658, #21252 ),
 ( #15740, #498, #7042 ),
 ( #8982, #14236, #15963 ),
 ( #5543, #17688, #7497 ),
 ( #3624, #21140, #4072 ),
 ( #3729, #19532, #17465 ),
 ( #16188, #8771, #12633 ),
 ( #2114, #14466, #9106 ),
 ( #10583, #14001, #16082 ),
 ( #21029, #19652, #17582 ),
 ( #3957, #17923, #2227 ),
 ( #5330, #12310, #1889 ),
 ( #8871, #155, #7149 ),
 ( #14120, #5442, #12417 ),
 ( #2000, #13304, #9556 ),
 ( #11381, #21597, #21705 ),
 ( #13193, #15029, #6004 ),
 ( #9666, #6121, #7723 ),
 ( #9331, #9781, #20328 ),
 ( #14696, #2340, #16310 ),
 ( #6237, #16773, #16541 ),
 ( #4519, #843, #7955 ),
 ( #12975, #6340, #19989 ),
 ( #7833, #11039, #16653 ),
 ( #22047, #21943, #18027 ) ),
 .UNSPECIFIED., .F., .F., .F. ) 
 B_SPLINE_SURFACE_WITH_KNOTS ( ( 4, 2, 2, 2, 2, 2, 2, 2, 2, 2, 2, 2, 2, 2, 2, 2, 2, 2, 4 ),
 ( 3, 3 ),
 ( 0.000000000000000000, 0.005809515383400559035, 0.008714273075100838553, 0.01161903076680111807, 0.01452378845850139759, 0.01742854615020167711, 0.02033330384190195489, 0.02178568268775209552, 0.02323806153360223614, 0.02614281922530251739, 0.02759519807115265455, 0.02904757691700279518, 0.03485709230040335421, 0.03630947114625349137, 0.03776184999210363546, 0.04066660768380390978, 0.04211898652965405387, 0.04357136537550419103, 0.04647612306720447228 ),
 ( 0.000000000000000000, 1.000000000000000000 ),
 .UNSPECIFIED. ) 
 GEOMETRIC_REPRESENTATION_ITEM ( )  RATIONAL_B_SPLINE_SURFACE ( (
 ( 1.000000000000000000, 0.6290213284793357840, 1.000000000000000000),
 ( 1.000000000000000000, 0.6248939334218988062, 1.000000000000000000),
 ( 1.000000000000000000, 0.6231525367052294095, 1.000000000000000000),
 ( 1.000000000000000000, 0.6225790212148355485, 1.000000000000000000),
 ( 1.000000000000000000, 0.6227321005834843826, 1.000000000000000000),
 ( 1.000000000000000000, 0.6234255931488940083, 1.000000000000000000),
 ( 1.000000000000000000, 0.6239617638513688114, 1.000000000000000000),
 ( 1.000000000000000000, 0.6251439415237010078, 1.000000000000000000),
 ( 1.000000000000000000, 0.6257917911431671865, 1.000000000000000000),
 ( 1.000000000000000000, 0.6269741839755182955, 1.000000000000000000),
 ( 1.000000000000000000, 0.6274966600224924917, 1.000000000000000000),
 ( 1.000000000000000000, 0.6282667852389482999, 1.000000000000000000),
 ( 1.000000000000000000, 0.6285148503998102543, 1.000000000000000000),
 ( 1.000000000000000000, 0.6286307432047592014, 1.000000000000000000),
 ( 1.000000000000000000, 0.6286269973787815823, 1.000000000000000000),
 ( 1.000000000000000000, 0.6285335994519584135, 1.000000000000000000),
 ( 1.000000000000000000, 0.6284444584874891992, 1.000000000000000000),
 ( 1.000000000000000000, 0.6280613430741410763, 1.000000000000000000),
 ( 1.000000000000000000, 0.6276496514169409568, 1.000000000000000000),
 ( 1.000000000000000000, 0.6268798492406927325, 1.000000000000000000),
 ( 1.000000000000000000, 0.6265983628749475232, 1.000000000000000000),
 ( 1.000000000000000000, 0.6260058463378762594, 1.000000000000000000),
 ( 1.000000000000000000, 0.6256937179550182693, 1.000000000000000000),
 ( 1.000000000000000000, 0.6241358698957584217, 1.000000000000000000),
 ( 1.000000000000000000, 0.6228888902089158019, 1.000000000000000000),
 ( 1.000000000000000000, 0.6226627606244575786, 1.000000000000000000),
 ( 1.000000000000000000, 0.6226866229701797373, 1.000000000000000000),
 ( 1.000000000000000000, 0.6229108014427007234, 1.000000000000000000),
 ( 1.000000000000000000, 0.6231102808943920213, 1.000000000000000000),
 ( 1.000000000000000000, 0.6240167787603944083, 1.000000000000000000),
 ( 1.000000000000000000, 0.6250322308941094196, 1.000000000000000000),
 ( 1.000000000000000000, 0.6273487183751635943, 1.000000000000000000),
 ( 1.000000000000000000, 0.6282530044593329643, 1.000000000000000000),
 ( 1.000000000000000000, 0.6303541273114475763, 1.000000000000000000),
 ( 1.000000000000000000, 0.6315549423244221083, 1.000000000000000000),
 ( 1.000000000000000000, 0.6356032421436564883, 1.000000000000000000),
 ( 1.000000000000000000, 0.6388921020275880602, 1.000000000000000000),
 ( 1.000000000000000000, 0.6428092274089116653, 1.000000000000000000) ) ) 
 REPRESENTATION_ITEM ( '' )  SURFACE ( )  );
#2703=VERTEX_POINT ( 'NONE', #11843 ) ;
#2709=CONICAL_SURFACE ( 'NONE', #10364, 2.099999999999997868, 1.029744258676653867 ) ;
#2711=FACE_OUTER_BOUND ( 'NONE', #8187, .T. ) ;
#2713=AXIS2_PLACEMENT_3D ( 'NONE', #11467, #8146, #6425 ) ;
#2720=EDGE_CURVE ( 'NONE', #13383, #15997, #1777, .T. ) ;
#2723=CARTESIAN_POINT ( 'NONE',  ( -16.50118549063250484, 8.665255721999203686, 59.66909312737204374 ) ) ;
#2725=CARTESIAN_POINT ( 'NONE',  ( -2.498922976470538515, 0.1467742037829277146, -52.32005940076825112 ) ) ;
#2727=AXIS2_PLACEMENT_3D ( 'NONE', #16544, #19769, #846 ) ;
#2729=CARTESIAN_POINT ( 'NONE',  ( 2.546974693918149679, 39.84782899243125343, 51.61921092574152681 ) ) ;
#2731=CARTESIAN_POINT ( 'NONE',  ( -2.576224933361803249, 39.84426458497839718, -51.65025110505525419 ) ) ;
#2732=DIRECTION ( 'NONE',  ( 2.659909329831104080E-15, 0.000000000000000000, 1.000000000000000000 ) ) ;
#2736=FACE_OUTER_BOUND ( 'NONE', #2926, .T. ) ;
#2742=CARTESIAN_POINT ( 'NONE',  ( -3.235223465815032728, -4.647308930658605952, -47.76313845446086503 ) ) ;
#2743=DIRECTION ( 'NONE',  ( -0.000000000000000000, -1.000000000000000000, -0.000000000000000000 ) ) ;
#2744=EDGE_CURVE ( 'NONE', #10749, #11797, #2126, .T. ) ;
#2748=CARTESIAN_POINT ( 'NONE',  ( -42.50000000000000711, -12.00000000000000000, -47.50000000000000000 ) ) ;
#2749=EDGE_LOOP ( 'NONE', ( #21722, #17724, #10308, #18794 ) ) ;
#2750=CARTESIAN_POINT ( 'NONE',  ( 0.4976208372498681087, 39.99853765106635706, -49.11738758647563685 ) ) ;
#2754=CARTESIAN_POINT ( 'NONE',  ( -4.925981507846746155, 40.00000000000000711, 51.57279734433891605 ) ) ;
#2757=CARTESIAN_POINT ( 'NONE',  ( -4.995686258823919701, 39.84470010994202482, 52.21048258191389380 ) ) ;
#2765=CARTESIAN_POINT ( 'NONE',  ( 13.00000000000024336, -2.516660498395250745, 60.00099999999999767 ) ) ;
#2768=CARTESIAN_POINT ( 'NONE',  ( 35.00000000000000000, -9.000000000000001776, 4.258610482196280173E-15 ) ) ;
#2770=ORIENTED_EDGE ( 'NONE', *, *, #423, .F. ) ;
#2771=CIRCLE ( 'NONE', #3518, 2.099999999999997868 ) ;
#2773=ADVANCED_FACE ( 'NONE', ( #8859, #3494, #18962, #11960, #141, #13987, #15829, #6812 ), #13777, .F. ) ;
#2774=ORIENTED_EDGE ( 'NONE', *, *, #8336, .T. ) ;
#2775=CARTESIAN_POINT ( 'NONE',  ( 17.21151300967877162, 30.19805602791846511, -59.88250013944306716 ) ) ;
#2779=EDGE_CURVE ( 'NONE', #7020, #20079, #10452, .T. ) ;
#2786=CARTESIAN_POINT ( 'NONE',  ( -12.06668108811420836, 11.08190912999967459, -44.43106897542661216 ) ) ;
#2788=CARTESIAN_POINT ( 'NONE',  ( 35.00000000000000000, 0.000000000000000000, 9.000000000000007105 ) ) ;
#2789=CARTESIAN_POINT ( 'NONE',  ( 3.995109193065607744, 40.00000000000000711, 51.09401218757847118 ) ) ;
#2794=ORIENTED_EDGE ( 'NONE', *, *, #5649, .F. ) ;
#2796=CARTESIAN_POINT ( 'NONE',  ( -6.041077103370461110, -0.8288449397156272269, 52.13906252460642321 ) ) ;
#2802=DIRECTION ( 'NONE',  ( -0.000000000000000000, 1.000000000000000000, -0.000000000000000000 ) ) ;
#2804=CARTESIAN_POINT ( 'NONE',  ( 16.86148599981780194, 30.79460519221557391, -57.23208912996602749 ) ) ;
#2805=EDGE_LOOP ( 'NONE', ( #5274, #9508, #9161, #20402 ) ) ;
#2807=ORIENTED_EDGE ( 'NONE', *, *, #1340, .T. ) ;
#2808=AXIS2_PLACEMENT_3D ( 'NONE', #17710, #17602, #22675 ) ;
#2814=CARTESIAN_POINT ( 'NONE',  ( -9.377138775076145905, -4.928932188134508507, 51.00555535510815730 ) ) ;
#2817=AXIS2_PLACEMENT_3D ( 'NONE', #21733, #2218, #12410 ) ;
#2819=EDGE_LOOP ( 'NONE', ( #9502, #16436, #14820, #21310 ) ) ;
#2822=DIRECTION ( 'NONE',  ( -0.000000000000000000, -1.000000000000000000, -0.000000000000000000 ) ) ;
#2825=EDGE_CURVE ( 'NONE', #790, #11530, #5209, .T. ) ;
#2826=CARTESIAN_POINT ( 'NONE',  ( -6.426802710256907858, 6.431242889908570071, 41.03786381671503847 ) ) ;
#2828=ADVANCED_FACE ( 'NONE', ( #14104 ), #5427, .T. ) ;
#2832=CARTESIAN_POINT ( 'NONE',  ( -16.86148599981783036, 30.79460519221558457, 57.23208912996606301 ) ) ;
#2837=CARTESIAN_POINT ( 'NONE',  ( 35.00000000000000000, 0.000000000000000000, 4.258610482196280173E-15 ) ) ;
#2842=LINE ( 'NONE', #21867, #10831 ) ;
#2844=CARTESIAN_POINT ( 'NONE',  ( -7.464612179280154969, 38.57206774498447288, -54.30634996223604105 ) ) ;
#2845=DIRECTION ( 'NONE',  ( -0.000000000000000000, 1.000000000000000000, -0.000000000000000000 ) ) ;
#2846=EDGE_LOOP ( 'NONE', ( #15417, #10007, #14803, #8317 ) ) ;
#2849=CARTESIAN_POINT ( 'NONE',  ( 42.50000000000000711, -11.97499999999999964, 47.50000000000000711 ) ) ;
#2851=CARTESIAN_POINT ( 'NONE',  ( 35.00000000000000000, 40.00000000000000000, 4.258610482196280173E-15 ) ) ;
#2853=DIRECTION ( 'NONE',  ( -1.000000000000000000, 0.000000000000000000, 0.000000000000000000 ) ) ;
#2854=ORIENTED_EDGE ( 'NONE', *, *, #2779, .T. ) ;
#2857=CARTESIAN_POINT ( 'NONE',  ( -0.7809641287214766914, -4.625293788890096458, -46.06432795380058565 ) ) ;
#2858=AXIS2_PLACEMENT_3D ( 'NONE', #7912, #21898, #7789 ) ;
#2862=CARTESIAN_POINT ( 'NONE',  ( 1.564866216807978994, -1.162741450739184890, 47.08240428779123476 ) ) ;
#2864=CARTESIAN_POINT ( 'NONE',  ( -42.50000000000000711, -11.97499999999999964, -47.50000000000000000 ) ) ;
#2870=CARTESIAN_POINT ( 'NONE',  ( -5.188160884119104033, 39.99999999999999289, 51.70385028745301526 ) ) ;
#2872=AXIS2_PLACEMENT_3D ( 'NONE', #2901, #4499, #18590 ) ;
#2873=CARTESIAN_POINT ( 'NONE',  ( -10.38193264731105003, 30.83255023748042944, -43.52061562521058136 ) ) ;
#2874=LINE ( 'NONE', #4710, #2262 ) ;
#2876=CARTESIAN_POINT ( 'NONE',  ( 14.52224280010135793, 23.83254695043585514, 45.61498238574513664 ) ) ;
#2880=EDGE_CURVE ( 'NONE', #11090, #16909, #17127, .T. ) ;
#2881=CARTESIAN_POINT ( 'NONE',  ( -0.005835298841899191902, 39.99999999999999289, -48.73851474269406481 ) ) ;
#2885=CARTESIAN_POINT ( 'NONE',  ( -1.387778780781445676E-14, 20.00000000000000000, -101.0000000000000284 ) ) ;
#2893=EDGE_CURVE ( 'NONE', #10333, #10996, #14180, .T. ) ;
#2895=CARTESIAN_POINT ( 'NONE',  ( 10.95224849132198131, 40.00000000000000000, 53.95427542910576335 ) ) ;
#2896=DIRECTION ( 'NONE',  ( -0.000000000000000000, -1.000000000000000000, -0.000000000000000000 ) ) ;
#2898=CARTESIAN_POINT ( 'NONE',  ( 18.99836266309356247, 13.69920652258249483, 60.37582729383724001 ) ) ;
#2901=CARTESIAN_POINT ( 'NONE',  ( 35.00000000000000000, 0.000000000000000000, 4.258610482196280173E-15 ) ) ;
#2902=VERTEX_POINT ( 'NONE', #7593 ) ;
#2904=CARTESIAN_POINT ( 'NONE',  ( -15.00000000000001421, 20.00000000000000000, -101.0000000000000284 ) ) ;
#2905=CONICAL_SURFACE ( 'NONE', #13466, 2.525000000000110489, 0.7853981633971014453 ) ;
#2907=CARTESIAN_POINT ( 'NONE',  ( -35.00000000000058265, 26.00000000000000355, -57.10000000000076170 ) ) ;
#2910=CARTESIAN_POINT ( 'NONE',  ( 2.774848782070428399, 40.00000000000000000, 50.42374031262293954 ) ) ;
#2911=ORIENTED_EDGE ( 'NONE', *, *, #5631, .F. ) ;
#2917=CARTESIAN_POINT ( 'NONE',  ( 2.432942025170123296E-14, -0.5379598322809753252, -48.80682109170825100 ) ) ;
#2918=ORIENTED_EDGE ( 'NONE', *, *, #20893, .T. ) ;
#2921=CARTESIAN_POINT ( 'NONE',  ( 35.00000000000058265, 40.00000000000000000, -55.00000000000076028 ) ) ;
#2922=ADVANCED_FACE ( 'NONE', ( #14449 ), #16770, .T. ) ;
#2923=CARTESIAN_POINT ( 'NONE',  ( 16.50118549063284590, 8.665255721999795213, -59.66909312737200821 ) ) ;
#2926=EDGE_LOOP ( 'NONE', ( #18294, #17238, #3471, #14348, #5498, #3287 ) ) ;
#2929=EDGE_LOOP ( 'NONE', ( #22524, #13285 ) ) ;
#2933=CARTESIAN_POINT ( 'NONE',  ( -5.770190843045729601, -4.767707482271699604, -49.21533144469186283 ) ) ;
#2934=ORIENTED_EDGE ( 'NONE', *, *, #20496, .F. ) ;
#2937=EDGE_LOOP ( 'NONE', ( #21696, #5503, #19295, #1870 ) ) ;
#2938=CARTESIAN_POINT ( 'NONE',  ( 4.628075497661257032, 39.46063506869912629, -53.65703709786517805 ) ) ;
#2939=DIRECTION ( 'NONE',  ( 0.000000000000000000, -1.000000000000000000, 0.000000000000000000 ) ) ;
#2941=CARTESIAN_POINT ( 'NONE',  ( -17.70396115872096132, 29.35428329955201576, -60.02641142872582236 ) ) ;
#2947=AXIS2_PLACEMENT_3D ( 'NONE', #10906, #18348, #7477 ) ;
#2950=CARTESIAN_POINT ( 'NONE',  ( -19.64963058618614511, 23.83053889022995619, 60.53829769526753779 ) ) ;
#2952=CARTESIAN_POINT ( 'NONE',  ( -16.30820259622267088, 8.415540886845235491, -59.60694662124532073 ) ) ;
#2953=CARTESIAN_POINT ( 'NONE',  ( 12.99999999999993960, 42.51666049839543149, -105.0000000000000142 ) ) ;
#2958=CYLINDRICAL_SURFACE ( 'NONE', #20451, 2.099999999999997868 ) ;
#2959=CARTESIAN_POINT ( 'NONE',  ( -0.9873823818543894237, 39.99999999999998579, -49.36449638065314360 ) ) ;
#2965=DIRECTION ( 'NONE',  ( -0.000000000000000000, -1.000000000000000000, -0.000000000000000000 ) ) ;
#2967=DIRECTION ( 'NONE',  ( 0.000000000000000000, 0.000000000000000000, 1.000000000000000000 ) ) ;
#2969=DIRECTION ( 'NONE',  ( 0.000000000000000000, 0.000000000000000000, 1.000000000000000000 ) ) ;
#2975=DIRECTION ( 'NONE',  ( -1.000000000000000000, 0.000000000000000000, 0.000000000000000000 ) ) ;
#2976=CYLINDRICAL_SURFACE ( 'NONE', #7979, 2.499999999999996891 ) ;
#2977=ORIENTED_EDGE ( 'NONE', *, *, #5631, .T. ) ;
#2978=CARTESIAN_POINT ( 'NONE',  ( 8.256135806678233990, -0.3920627093407412778, 55.63523492903830459 ) ) ;
#2979=AXIS2_PLACEMENT_3D ( 'NONE', #21518, #4894, #5011 ) ;
#2980=CARTESIAN_POINT ( 'NONE',  ( 42.50000000000000711, -12.00000000000000000, 47.50000000000000711 ) ) ;
#2981=CARTESIAN_POINT ( 'NONE',  ( -9.952189117650851458, 40.00000000000000000, -53.64426396172072486 ) ) ;
#2982=DIRECTION ( 'NONE',  ( -0.000000000000000000, -0.000000000000000000, 1.000000000000000000 ) ) ;
#2983=CARTESIAN_POINT ( 'NONE',  ( -14.40375226887236515, 24.20453657423045968, -45.56106839101555295 ) ) ;
#2984=EDGE_CURVE ( 'NONE', #8022, #6315, #11312, .T. ) ;
#2985=DIRECTION ( 'NONE',  ( -0.000000000000000000, 1.000000000000000000, -0.000000000000000000 ) ) ;
#2987=CARTESIAN_POINT ( 'NONE',  ( 14.87996495114178508, 21.93329436794035914, 45.77322900830825603 ) ) ;
#2989=DIRECTION ( 'NONE',  ( 0.000000000000000000, 0.000000000000000000, -1.000000000000000000 ) ) ;
#2997=ORIENTED_EDGE ( 'NONE', *, *, #19076, .T. ) ;
#2999=ADVANCED_FACE ( 'NONE', ( #21460 ), #7480, .T. ) ;
#3003=CARTESIAN_POINT ( 'NONE',  ( 10.27431133777208316, -4.928932188134517389, 51.43682631505490832 ) ) ;
#3004=CYLINDRICAL_SURFACE ( 'NONE', #16835, 9.000000000000003553 ) ;
#3006=CARTESIAN_POINT ( 'NONE',  ( -2.114046819835667446, 5.114762345337546812, -38.90380387758576575 ) ) ;
#3008=CARTESIAN_POINT ( 'NONE',  ( 35.00000000000000000, 38.99999999999999289, 4.258610482196280173E-15 ) ) ;
#3010=ORIENTED_EDGE ( 'NONE', *, *, #7740, .F. ) ;
#3013=CIRCLE ( 'NONE', #18001, 6.499999999999999112 ) ;
#3015=CARTESIAN_POINT ( 'NONE',  ( 9.952189117650764416, 40.00000000000000000, 53.64426396172094513 ) ) ;
#3017=CARTESIAN_POINT ( 'NONE',  ( -9.066530188944724955, 39.99999999999999289, -53.36211916096569752 ) ) ;
#3021=ORIENTED_EDGE ( 'NONE', *, *, #4693, .T. ) ;
#3023=DIRECTION ( 'NONE',  ( -0.000000000000000000, -1.000000000000000000, -0.000000000000000000 ) ) ;
#3025=CARTESIAN_POINT ( 'NONE',  ( 19.27753112431989635, 25.39788459340050153, -57.95296232962348171 ) ) ;
#3026=EDGE_CURVE ( 'NONE', #21259, #8676, #13482, .T. ) ;
#3028=VECTOR ( 'NONE', #1480, 1000.000000000000000 ) ;
#3031=EDGE_CURVE ( 'NONE', #19508, #17065, #3824, .T. ) ;
#3033=ORIENTED_EDGE ( 'NONE', *, *, #22659, .F. ) ;
#3034=CARTESIAN_POINT ( 'NONE',  ( 10.95789470907245189, 39.14627205505679086, 55.00167764548202598 ) ) ;
#3035=DIRECTION ( 'NONE',  ( 0.000000000000000000, 1.000000000000000000, 0.000000000000000000 ) ) ;
#3038=CARTESIAN_POINT ( 'NONE',  ( 35.00000000000000000, 40.00000000000000000, 4.258610482196280173E-15 ) ) ;
#3039=DIRECTION ( 'NONE',  ( 0.000000000000000000, -0.7071067811865302533, -0.7071067811865647812 ) ) ;
#3040=VERTEX_POINT ( 'NONE', #9090 ) ;
#3042=VERTEX_POINT ( 'NONE', #7367 ) ;
#3043=FACE_OUTER_BOUND ( 'NONE', #10903, .T. ) ;
#3047=CARTESIAN_POINT ( 'NONE',  ( -15.58352763714665556, 32.54529335663308842, -59.37339313163356991 ) ) ;
#3048=CIRCLE ( 'NONE', #21707, 1.999999999999999778 ) ;
#3049=CARTESIAN_POINT ( 'NONE',  ( -11.84374239103370563, 10.78799321809638734, 44.31542800769557289 ) ) ;
#3053=ORIENTED_EDGE ( 'NONE', *, *, #13561, .F. ) ;
#3054=CARTESIAN_POINT ( 'NONE',  ( -19.88294660283940374, 17.66261523023111124, 60.59423886784515645 ) ) ;
#3055=DIRECTION ( 'NONE',  ( -1.000000000000000000, 0.000000000000000000, 0.000000000000000000 ) ) ;
#3057=CARTESIAN_POINT ( 'NONE',  ( -42.50000000000000711, -5.000000000000000000, 47.50000000000000711 ) ) ;
#3058=AXIS2_PLACEMENT_3D ( 'NONE', #19171, #22502, #3132 ) ;
#3060=EDGE_CURVE ( 'NONE', #11765, #11771, #13127, .T. ) ;
#3062=ORIENTED_EDGE ( 'NONE', *, *, #5369, .F. ) ;
#3064=DIRECTION ( 'NONE',  ( -0.000000000000000000, 1.000000000000000000, -0.000000000000000000 ) ) ;
#3067=EDGE_LOOP ( 'NONE', ( #4156, #14561, #11052, #2355 ) ) ;
#3068=EDGE_CURVE ( 'NONE', #17245, #22326, #18702, .T. ) ;
#3074=CARTESIAN_POINT ( 'NONE',  ( 35.00000000000000000, -9.000000000000001776, 4.258610482196280173E-15 ) ) ;
#3076=AXIS2_PLACEMENT_3D ( 'NONE', #17866, #5594, #7097 ) ;
#3080=EDGE_CURVE ( 'NONE', #9683, #17743, #10559, .T. ) ;
#3081=AXIS2_PLACEMENT_3D ( 'NONE', #14799, #18600, #4627 ) ;
#3082=DIRECTION ( 'NONE',  ( -0.000000000000000000, -0.000000000000000000, 1.000000000000000000 ) ) ;
#3087=CARTESIAN_POINT ( 'NONE',  ( -9.952189117650851458, 40.00000000000000000, -53.64426396172072486 ) ) ;
#3088=CARTESIAN_POINT ( 'NONE',  ( -22.20997089757256049, 23.22761694305070534, -58.62102808997008907 ) ) ;
#3090=CARTESIAN_POINT ( 'NONE',  ( -0.7361830413879804080, 39.99998182960236193, 49.30709089395045197 ) ) ;
#3091=CARTESIAN_POINT ( 'NONE',  ( -17.76087593031472522, 33.76750075041050536, 57.47290953699844351 ) ) ;
#3093=CARTESIAN_POINT ( 'NONE',  ( 13.08927703801864872, 27.36553638769444063, 44.94509734929667388 ) ) ;
#3094=CARTESIAN_POINT ( 'NONE',  ( -35.00000000000058265, 40.00000000000000711, -55.00000000000076028 ) ) ;
#3096=DIRECTION ( 'NONE',  ( -0.000000000000000000, -0.000000000000000000, -1.000000000000000000 ) ) ;
#3104=EDGE_CURVE ( 'NONE', #2120, #12680, #21562, .T. ) ;
#3106=ORIENTED_EDGE ( 'NONE', *, *, #10249, .T. ) ;
#3109=DIRECTION ( 'NONE',  ( 0.000000000000000000, 0.000000000000000000, -1.000000000000000000 ) ) ;
#3122=CARTESIAN_POINT ( 'NONE',  ( 9.689843208404314012, 39.33333333333335702, 54.54983754392762307 ) ) ;
#3125=ADVANCED_FACE ( 'NONE', ( #2673 ), #6219, .T. ) ;
#3128=CARTESIAN_POINT ( 'NONE',  ( -20.10834676944521249, 10.02088872142242693, 58.12296025200766536 ) ) ;
#3129=ORIENTED_EDGE ( 'NONE', *, *, #12487, .T. ) ;
#3132=DIRECTION ( 'NONE',  ( 0.000000000000000000, 0.000000000000000000, -1.000000000000000000 ) ) ;
#3136=CARTESIAN_POINT ( 'NONE',  ( 20.25803107563791983, 29.70716601075176300, -58.16264420749838138 ) ) ;
#3138=VERTEX_POINT ( 'NONE', #828 ) ;
#3139=B_SPLINE_CURVE_WITH_KNOTS ( 'NONE', 3,
 ( #22338, #18886, #15538, #8567, #3316, #22219 ),
 .UNSPECIFIED., .F., .F.,
 ( 4, 2, 4 ),
 ( 1.734723475976807094E-18, 0.003173601132114239540, 0.006347202264228477345 ),
 .UNSPECIFIED. ) ;
#3140=AXIS2_PLACEMENT_3D ( 'NONE', #16818, #9493, #13351 ) ;
#3146=FACE_OUTER_BOUND ( 'NONE', #13165, .T. ) ;
#3147=DIRECTION ( 'NONE',  ( 0.000000000000000000, 0.000000000000000000, 1.000000000000000000 ) ) ;
#3149=CARTESIAN_POINT ( 'NONE',  ( -42.50000000000000711, -12.00000000000000000, -47.50000000000000000 ) ) ;
#3150=CARTESIAN_POINT ( 'NONE',  ( -2.066061548966867889, -1.174227811081267614, -49.70141618117483517 ) ) ;
#3152=CIRCLE ( 'NONE', #17050, 15.00000000000000000 ) ;
#3157=CARTESIAN_POINT ( 'NONE',  ( 8.957608338236010326, 39.56964539817487037, -54.21301299504590077 ) ) ;
#3158=LINE ( 'NONE', #10125, #6157 ) ;
#3159=CARTESIAN_POINT ( 'NONE',  ( 6.696867368504048330E-15, 5.000000000000000888, 38.73397172404480671 ) ) ;
#3160=CARTESIAN_POINT ( 'NONE',  ( -2.243248548005440046, 39.96968647079420123, 50.39828113659874731 ) ) ;
#3165=CARTESIAN_POINT ( 'NONE',  ( 8.916870955515532771, 2.080241304161451144, -56.50845996868347498 ) ) ;
#3166=CIRCLE ( 'NONE', #7924, 2.500000000000002220 ) ;
#3167=ORIENTED_EDGE ( 'NONE', *, *, #3026, .F. ) ;
#3170=EDGE_CURVE ( 'NONE', #15847, #19175, #19739, .T. ) ;
#3173=DIRECTION ( 'NONE',  ( -1.000000000000000000, 0.000000000000000000, 0.000000000000000000 ) ) ;
#3176=B_SPLINE_CURVE_WITH_KNOTS ( 'NONE', 3,
 ( #11857, #11636, #1106, #3165, #10132, #17124 ),
 .UNSPECIFIED., .F., .F.,
 ( 4, 2, 4 ),
 ( 0.000000000000000000, 0.002641318319677479071, 0.005282636639354958141 ),
 .UNSPECIFIED. ) ;
#3180=EDGE_CURVE ( 'NONE', #2243, #15662, #14792, .T. ) ;
#3181=ORIENTED_EDGE ( 'NONE', *, *, #6274, .T. ) ;
#3183=CARTESIAN_POINT ( 'NONE',  ( -7.892682273998517850, 40.00000000000000000, -52.92195235550753551 ) ) ;
#3186=AXIS2_PLACEMENT_3D ( 'NONE', #21667, #5741, #9522 ) ;
#3188=CARTESIAN_POINT ( 'NONE',  ( 42.50000000000000711, -12.00000000000012434, 44.97499999999989484 ) ) ;
#3189=VECTOR ( 'NONE', #3945, 1000.000000000000114 ) ;
#3190=ORIENTED_EDGE ( 'NONE', *, *, #1104, .T. ) ;
#3193=FACE_OUTER_BOUND ( 'NONE', #4822, .T. ) ;
#3205=DIRECTION ( 'NONE',  ( 0.8171172023792930839, 0.3308262969259979092, 0.4720947350247287067 ) ) ;
#3207=CARTESIAN_POINT ( 'NONE',  ( -28.50000000000001421, 19.99999999999982947, 60.00099999999999767 ) ) ;
#3209=CARTESIAN_POINT ( 'NONE',  ( -20.89003165053261313, 11.75591475223743210, -58.31867307082492147 ) ) ;
#3210=DIRECTION ( 'NONE',  ( 0.000000000000000000, 0.000000000000000000, 1.000000000000000000 ) ) ;
#3212=CARTESIAN_POINT ( 'NONE',  ( -14.30127497006392012, 34.01755211514664978, 56.34491176086896047 ) ) ;
#3213=EDGE_LOOP ( 'NONE', ( #17359, #9039 ) ) ;
#3214=CARTESIAN_POINT ( 'NONE',  ( 29.99999999999998579, 20.00000000000000355, -105.0000000000000142 ) ) ;
#3217=CARTESIAN_POINT ( 'NONE',  ( 13.56354382738788367, 2.142135623730777372, -56.03997097393713034 ) ) ;
#3218=CARTESIAN_POINT ( 'NONE',  ( -35.00000000000058265, 28.00000000000000000, -55.00000000000076028 ) ) ;
#3220=DIRECTION ( 'NONE',  ( 0.000000000000000000, 0.000000000000000000, 1.000000000000000000 ) ) ;
#3221=LINE ( 'NONE', #10187, #216 ) ;
#3224=EDGE_CURVE ( 'NONE', #12952, #8904, #8491, .T. ) ;
#3225=VECTOR ( 'NONE', #9664, 1000.000000000000000 ) ;
#3227=CIRCLE ( 'NONE', #16011, 10.00000000000000178 ) ;
#3230=CARTESIAN_POINT ( 'NONE',  ( 6.696867368503558448E-15, 0.000000000000000000, 48.73397172404481381 ) ) ;
#3238=EDGE_LOOP ( 'NONE', ( #4771, #12071 ) ) ;
#3239=CARTESIAN_POINT ( 'NONE',  ( -5.833333333333340143, 39.00000000000000711, -40.61164310337066041 ) ) ;
#3242=CARTESIAN_POINT ( 'NONE',  ( -42.50000000000000711, -12.00000000000000000, -47.50000000000000000 ) ) ;
#3243=CARTESIAN_POINT ( 'NONE',  ( 7.474679896992488359, 39.63145871420505273, 53.58934897198174241 ) ) ;
#3248=DIRECTION ( 'NONE',  ( -0.000000000000000000, 1.000000000000000000, -0.000000000000000000 ) ) ;
#3252=EDGE_CURVE ( 'NONE', #10996, #10333, #13849, .T. ) ;
#3253=AXIS2_PLACEMENT_3D ( 'NONE', #14800, #20096, #16180 ) ;
#3260=CIRCLE ( 'NONE', #5080, 2.099999999999990763 ) ;
#3264=ORIENTED_EDGE ( 'NONE', *, *, #2607, .T. ) ;
#3266=CARTESIAN_POINT ( 'NONE',  ( -8.331955809010628045, 38.18181818181818699, 56.36098470834075158 ) ) ;
#3267=CARTESIAN_POINT ( 'NONE',  ( -34.99999999999980815, 26.00000000000000355, 57.09999999999921982 ) ) ;
#3274=DIRECTION ( 'NONE',  ( -0.000000000000000000, -1.000000000000000000, -0.000000000000000000 ) ) ;
#3275=DIRECTION ( 'NONE',  ( 0.000000000000000000, 0.000000000000000000, 1.000000000000000000 ) ) ;
#3279=CARTESIAN_POINT ( 'NONE',  ( -42.50000000000000711, -12.00000000000012434, 47.50000000000000711 ) ) ;
#3281=CARTESIAN_POINT ( 'NONE',  ( -0.9695481421535360189, 39.99443253533478781, 49.47361716149077182 ) ) ;
#3287=ORIENTED_EDGE ( 'NONE', *, *, #3841, .F. ) ;
#3289=EDGE_CURVE ( 'NONE', #7701, #21800, #20982, .T. ) ;
#3296=CARTESIAN_POINT ( 'NONE',  ( -90.00000000000000000, 40.00000000000000711, -9.108981535246192915E-16 ) ) ;
#3297=CARTESIAN_POINT ( 'NONE',  ( -11.85142133643352480, 40.00000000000000711, 54.27688992489014908 ) ) ;
#3298=EDGE_CURVE ( 'NONE', #21800, #16, #21928, .T. ) ;
#3300=ORIENTED_EDGE ( 'NONE', *, *, #14528, .F. ) ;
#3302=CARTESIAN_POINT ( 'NONE',  ( -8.540030425000768588, 39.99999999999998579, -53.17106805020448945 ) ) ;
#3307=( BOUNDED_SURFACE ( )  B_SPLINE_SURFACE ( 3, 2, ( 
 ( #12972, #2573, #18364 ),
 ( #4632, #11610, #18605 ),
 ( #841, #18262, #16539 ),
 ( #2684, #9890, #7830 ),
 ( #1079, #7951, #8067 ),
 ( #14913, #9662, #21940 ),
 ( #20440, #18715, #16880 ),
 ( #8172, #6232, #6789 ) ),
 .UNSPECIFIED., .F., .F., .F. ) 
 B_SPLINE_SURFACE_WITH_KNOTS ( ( 4, 2, 2, 4 ),
 ( 3, 3 ),
 ( 0.000000000000000000, 0.005619275362615350038, 0.008428913043923024623, 0.01123855072523070008 ),
 ( 0.000000000000000000, 1.000000000000000000 ),
 .UNSPECIFIED. ) 
 GEOMETRIC_REPRESENTATION_ITEM ( )  RATIONAL_B_SPLINE_SURFACE ( (
 ( 1.000000000000000000, 0.7200096751079133606, 1.000000000000000000),
 ( 1.000000000000000000, 0.7496867072825520451, 1.000000000000000000),
 ( 1.000000000000000000, 0.7737790075298972559, 1.000000000000000000),
 ( 1.000000000000000000, 0.8024253043749317582, 1.000000000000000000),
 ( 1.000000000000000000, 0.8107149009171402687, 1.000000000000000000),
 ( 1.000000000000000000, 0.8248887618771173491, 1.000000000000000000),
 ( 1.000000000000000000, 0.8307759608768628956, 1.000000000000000000),
 ( 1.000000000000000000, 0.8354972831517065712, 1.000000000000000000) ) ) 
 REPRESENTATION_ITEM ( '' )  SURFACE ( )  );
#3308=ORIENTED_EDGE ( 'NONE', *, *, #357, .T. ) ;
#3309=EDGE_CURVE ( 'NONE', #22647, #15500, #14945, .T. ) ;
#3311=EDGE_LOOP ( 'NONE', ( #5449, #14473 ) ) ;
#3313=CARTESIAN_POINT ( 'NONE',  ( 42.50000000000000711, -12.00000000000000000, -47.50000000000000000 ) ) ;
#3316=CARTESIAN_POINT ( 'NONE',  ( -1.072795092646378734, 35.00000000000000000, 38.73397172404480671 ) ) ;
#3329=CARTESIAN_POINT ( 'NONE',  ( -20.00424115936587199, 19.83711385861052889, -60.62278039730740886 ) ) ;
#3330=ADVANCED_FACE ( 'NONE', ( #20876 ), #2905, .F. ) ;
#3333=CARTESIAN_POINT ( 'NONE',  ( -12.99999999999980282, -2.516660498395516310, -105.0010000000000048 ) ) ;
#3335=EDGE_CURVE ( 'NONE', #11258, #2243, #6559, .T. ) ;
#3336=FACE_BOUND ( 'NONE', #1977, .T. ) ;
#3338=ORIENTED_EDGE ( 'NONE', *, *, #9562, .T. ) ;
#3339=CIRCLE ( 'NONE', #11005, 18.00000000000000000 ) ;
#3340=LINE ( 'NONE', #18571, #11181 ) ;
#3346=CARTESIAN_POINT ( 'NONE',  ( 0.7217013449060836194, -4.626342591398014292, 46.01887142923336427 ) ) ;
#3348=CARTESIAN_POINT ( 'NONE',  ( -1.387778780781445518E-14, 20.00000000000000355, 100.0000000000000000 ) ) ;
#3351=CARTESIAN_POINT ( 'NONE',  ( -11.87329829276355042, 39.99999999999998579, 54.28004929203131468 ) ) ;
#3353=LINE ( 'NONE', #3239, #14138 ) ;
#3356=DIRECTION ( 'NONE',  ( 0.8391477167891899791, 0.3845457931435842802, 0.3846500258456529431 ) ) ;
#3357=LINE ( 'NONE', #1627, #2029 ) ;
#3358=CARTESIAN_POINT ( 'NONE',  ( 10.38220159744132509, 30.85082733156617607, -43.52345836121336475 ) ) ;
#3361=DIRECTION ( 'NONE',  ( -0.000000000000000000, -1.000000000000000000, -0.000000000000000000 ) ) ;
#3364=CIRCLE ( 'NONE', #22017, 10.00000000000000178 ) ;
#3366=DIRECTION ( 'NONE',  ( -0.000000000000000000, 1.000000000000000000, -0.000000000000000000 ) ) ;
#3368=CARTESIAN_POINT ( 'NONE',  ( -90.00000000000000000, 26.00000000000000355, -2.099999999999991651 ) ) ;
#3369=ORIENTED_EDGE ( 'NONE', *, *, #11016, .F. ) ;
#3372=DIRECTION ( 'NONE',  ( 0.000000000000000000, 0.000000000000000000, 1.000000000000000000 ) ) ;
#3375=CARTESIAN_POINT ( 'NONE',  ( 22.39119123459438043, 18.77992731964035755, 58.66020055843083014 ) ) ;
#3381=FACE_OUTER_BOUND ( 'NONE', #9789, .T. ) ;
#3384=CARTESIAN_POINT ( 'NONE',  ( 1.838758599476162825, 34.88915224291387318, 38.90097524723616829 ) ) ;
#3385=ORIENTED_EDGE ( 'NONE', *, *, #39, .F. ) ;
#3386=CARTESIAN_POINT ( 'NONE',  ( 5.905685660495028522, 39.12130596110461767, -53.51375433846526875 ) ) ;
#3387=DIRECTION ( 'NONE',  ( 0.000000000000000000, 0.000000000000000000, -1.000000000000000000 ) ) ;
#3388=CARTESIAN_POINT ( 'NONE',  ( -4.557459432784731312, 39.87073546004029367, 51.93758234736819190 ) ) ;
#3390=CARTESIAN_POINT ( 'NONE',  ( 13.56354382738799558, 2.142135623730931471, 56.03997097393685323 ) ) ;
#3392=AXIS2_PLACEMENT_3D ( 'NONE', #15750, #60, #7052 ) ;
#3395=ORIENTED_EDGE ( 'NONE', *, *, #12725, .F. ) ;
#3397=ORIENTED_EDGE ( 'NONE', *, *, #8346, .F. ) ;
#3398=VERTEX_POINT ( 'NONE', #16139 ) ;
#3399=VERTEX_POINT ( 'NONE', #11106 ) ;
#3400=CARTESIAN_POINT ( 'NONE',  ( -13.03660953228011010, 4.807999378483081898, 58.46122805341369855 ) ) ;
#3403=CARTESIAN_POINT ( 'NONE',  ( 42.50000000000000711, -9.600000000000001421, 47.50000000000000711 ) ) ;
#3404=CARTESIAN_POINT ( 'NONE',  ( -12.99999999999980282, -2.516660498395516310, -100.0000000000000000 ) ) ;
#3405=CARTESIAN_POINT ( 'NONE',  ( 1.076296735955945660, 39.99310909908677303, 49.55311975943427427 ) ) ;
#3406=CIRCLE ( 'NONE', #11030, 10.00000000000000178 ) ;
#3409=CARTESIAN_POINT ( 'NONE',  ( -5.708997464095411090, 39.99999999999998579, -51.95724526860413306 ) ) ;
#3411=CARTESIAN_POINT ( 'NONE',  ( 7.505578006071305985, 1.461761173326671104, 55.63523492903841117 ) ) ;
#3412=EDGE_CURVE ( 'NONE', #21198, #18097, #8734, .T. ) ;
#3413=VERTEX_POINT ( 'NONE', #19385 ) ;
#3414=CARTESIAN_POINT ( 'NONE',  ( 42.50000000000000711, -12.00000000000012434, -47.50000000000000000 ) ) ;
#3415=VERTEX_POINT ( 'NONE', #5850 ) ;
#3416=CARTESIAN_POINT ( 'NONE',  ( -7.555723902515834922, 38.52224445567419764, 55.93227658743229114 ) ) ;
#3418=FACE_BOUND ( 'NONE', #12714, .T. ) ;
#3423=VECTOR ( 'NONE', #10978, 1000.000000000000000 ) ;
#3425=ORIENTED_EDGE ( 'NONE', *, *, #16886, .T. ) ;
#3429=CARTESIAN_POINT ( 'NONE',  ( 13.07600923154786088, 12.64060470162857364, 44.93756990742568291 ) ) ;
#3432=CARTESIAN_POINT ( 'NONE',  ( -1.387778780781445518E-14, 20.00000000000000355, 103.0000000000000284 ) ) ;
#3433=CARTESIAN_POINT ( 'NONE',  ( -16.49514046905042264, 8.656442121909590171, -59.66722042020315087 ) ) ;
#3435=CONICAL_SURFACE ( 'NONE', #9279, 49.99999999999998579, 0.7853981633974657095 ) ;
#3437=VERTEX_POINT ( 'NONE', #2413 ) ;
#3439=FACE_BOUND ( 'NONE', #5934, .T. ) ;
#3443=DIRECTION ( 'NONE',  ( -0.000000000000000000, 1.000000000000000000, -0.000000000000000000 ) ) ;
#3450=CIRCLE ( 'NONE', #12919, 51.00000000000001421 ) ;
#3452=AXIS2_PLACEMENT_3D ( 'NONE', #9395, #4360, #4237 ) ;
#3456=ORIENTED_EDGE ( 'NONE', *, *, #10987, .T. ) ;
#3459=DIRECTION ( 'NONE',  ( 0.000000000000000000, 0.000000000000000000, -1.000000000000000000 ) ) ;
#3461=CARTESIAN_POINT ( 'NONE',  ( 12.99999999999993960, 42.51666049839543149, 100.0000000000000000 ) ) ;
#3462=ORIENTED_EDGE ( 'NONE', *, *, #12562, .T. ) ;
#3463=DIRECTION ( 'NONE',  ( -0.000000000000000000, -1.000000000000000000, -0.000000000000000000 ) ) ;
#3466=CARTESIAN_POINT ( 'NONE',  ( 3.235223465815040278, -4.647308930658603288, -47.76313845446085793 ) ) ;
#3468=CARTESIAN_POINT ( 'NONE',  ( 5.833333333333339255, 6.180730040185842711, 40.61164310337068173 ) ) ;
#3471=ORIENTED_EDGE ( 'NONE', *, *, #16678, .T. ) ;
#3473=AXIS2_PLACEMENT_3D ( 'NONE', #9453, #503, #21364 ) ;
#3474=CARTESIAN_POINT ( 'NONE',  ( -42.50000000000000711, -5.000000000000000000, 49.60000000000000853 ) ) ;
#3485=EDGE_LOOP ( 'NONE', ( #8615, #10110, #2918, #13373 ) ) ;
#3486=EDGE_LOOP ( 'NONE', ( #20263, #6307, #6714, #22054 ) ) ;
#3488=CIRCLE ( 'NONE', #20671, 57.07106781186551103 ) ;
#3489=CARTESIAN_POINT ( 'NONE',  ( 14.98269809772825489, 3.197274675470657357, 56.58282704237544891 ) ) ;
#3491=CARTESIAN_POINT ( 'NONE',  ( 8.910373529401164561, 39.99999999999999289, 53.30647735977077417 ) ) ;
#3494=FACE_BOUND ( 'NONE', #18429, .T. ) ;
#3495=CARTESIAN_POINT ( 'NONE',  ( 0.05567163769005373242, -4.650449146058893923, -45.38800358221575948 ) ) ;
#3497=CARTESIAN_POINT ( 'NONE',  ( 34.99999999999980815, 40.00000000000000711, 52.47499999999922693 ) ) ;
#3499=CARTESIAN_POINT ( 'NONE',  ( 35.00000000000058265, 26.00000000000000355, -52.90000000000076597 ) ) ;
#3501=CARTESIAN_POINT ( 'NONE',  ( 0.6290164960677582240, 40.00000000000000000, -49.48738346576788416 ) ) ;
#3504=CARTESIAN_POINT ( 'NONE',  ( -2.105491371362254949, 39.97335800984880194, 50.30091810999239499 ) ) ;
#3508=VECTOR ( 'NONE', #5185, 1000.000000000000000 ) ;
#3513=AXIS2_PLACEMENT_3D ( 'NONE', #16509, #7799, #5748 ) ;
#3515=ORIENTED_EDGE ( 'NONE', *, *, #5686, .F. ) ;
#3517=DIRECTION ( 'NONE',  ( 0.000000000000000000, -0.5150380749100547106, -0.8571673007021120005 ) ) ;
#3518=AXIS2_PLACEMENT_3D ( 'NONE', #18049, #2822, #4430 ) ;
#3520=CARTESIAN_POINT ( 'NONE',  ( 8.331955809010601399, 38.18181818181818699, 56.36098470834073026 ) ) ;
#3522=CARTESIAN_POINT ( 'NONE',  ( 1.092487586117354859, 39.99289797745701236, 49.56515079790309386 ) ) ;
#3526=CARTESIAN_POINT ( 'NONE',  ( -9.260192196558032052, 40.00000000000000000, -53.42688922523713302 ) ) ;
#3527=CARTESIAN_POINT ( 'NONE',  ( 12.84899528830092130, 2.142135623730915039, -57.90797000640139913 ) ) ;
#3532=ORIENTED_EDGE ( 'NONE', *, *, #16392, .F. ) ;
#3536=CIRCLE ( 'NONE', #6456, 2.099999999999997868 ) ;
#3539=FACE_OUTER_BOUND ( 'NONE', #11919, .T. ) ;
#3540=DIRECTION ( 'NONE',  ( 0.000000000000000000, -1.000000000000000000, 0.000000000000000000 ) ) ;
#3542=CIRCLE ( 'NONE', #1701, 2.499999999999998668 ) ;
#3544=ORIENTED_EDGE ( 'NONE', *, *, #21402, .F. ) ;
#3545=CARTESIAN_POINT ( 'NONE',  ( -0.6864184775308176389, -1.216838870806101092, -47.75834167804065800 ) ) ;
#3546=CARTESIAN_POINT ( 'NONE',  ( 11.85142133643347506, 39.99999999999999289, -54.27688992489011355 ) ) ;
#3547=AXIS2_PLACEMENT_3D ( 'NONE', #20995, #19393, #1962 ) ;
#3548=VERTEX_POINT ( 'NONE', #14420 ) ;
#3552=EDGE_CURVE ( 'NONE', #7430, #16727, #3048, .T. ) ;
#3553=CARTESIAN_POINT ( 'NONE',  ( -9.814839119317305460, 37.44644195123124319, -57.08682537453712769 ) ) ;
#3559=DIRECTION ( 'NONE',  ( 0.000000000000000000, -1.000000000000000000, 0.000000000000000000 ) ) ;
#3560=CARTESIAN_POINT ( 'NONE',  ( 34.99999999999980815, 28.00000000000000000, 52.49999999999922551 ) ) ;
#3562=ORIENTED_EDGE ( 'NONE', *, *, #11829, .F. ) ;
#3568=CARTESIAN_POINT ( 'NONE',  ( 0.2227364088704490985, -1.232651810762517064, 48.42315971483671433 ) ) ;
#3571=DIRECTION ( 'NONE',  ( -0.000000000000000000, -1.000000000000000000, -0.000000000000000000 ) ) ;
#3572=CARTESIAN_POINT ( 'NONE',  ( -15.49999999999980460, -2.516660498395515866, 100.0000000000000000 ) ) ;
#3574=ORIENTED_EDGE ( 'NONE', *, *, #14203, .F. ) ;
#3579=CYLINDRICAL_SURFACE ( 'NONE', #8684, 2.499999999999995115 ) ;
#3584=CYLINDRICAL_SURFACE ( 'NONE', #17715, 20.00000000000000000 ) ;
#3586=DIRECTION ( 'NONE',  ( -1.000000000000000000, 0.000000000000000000, 0.000000000000000000 ) ) ;
#3588=CARTESIAN_POINT ( 'NONE',  ( -17.98964431006460174, 6.536084871031949461, 57.54127157382312419 ) ) ;
#3589=EDGE_LOOP ( 'NONE', ( #3395, #17004 ) ) ;
#3590=CARTESIAN_POINT ( 'NONE',  ( 13.56354382738799735, 2.142135623730926142, 56.03997097393686033 ) ) ;
#3595=CYLINDRICAL_SURFACE ( 'NONE', #14729, 2.499999999999995115 ) ;
#3596=B_SPLINE_CURVE_WITH_KNOTS ( 'NONE', 3,
 ( #19002, #9713, #10604, #10269, #8675, #8560, #7175, #5143, #15533, #19223, #14144, #7063, #22557, #1571, #9008, #6853, #12331, #17493, #8794, #10375, #13817, #20835 ),
 .UNSPECIFIED., .F., .F.,
 ( 4, 2, 2, 2, 2, 2, 2, 2, 2, 2, 4 ),
 ( 0.000000000000000000, 0.005822207826702250309, 0.007277759783377815705, 0.008733311740053380234, 0.01164441565340452317, 0.01309996761008009464, 0.01455551956675566784, 0.01746662348010682292, 0.01892217543678240133, 0.02037772739345797973, 0.02328883130680912961 ),
 .UNSPECIFIED. ) ;
#3600=EDGE_LOOP ( 'NONE', ( #715, #15242 ) ) ;
#3601=EDGE_LOOP ( 'NONE', ( #21781, #13201, #16226, #1209 ) ) ;
#3603=ORIENTED_EDGE ( 'NONE', *, *, #2128, .F. ) ;
#3606=DIRECTION ( 'NONE',  ( -1.000000000000000000, 0.000000000000000000, 0.000000000000000000 ) ) ;
#3614=CARTESIAN_POINT ( 'NONE',  ( -13.32368996328071376, 38.03919112700260285, -55.94897837928603934 ) ) ;
#3617=CARTESIAN_POINT ( 'NONE',  ( 0.5350771668691457483, 35.00000000000000711, 38.73397172404481381 ) ) ;
#3618=ORIENTED_EDGE ( 'NONE', *, *, #2825, .T. ) ;
#3619=CARTESIAN_POINT ( 'NONE',  ( 0.7832304697071968969, 40.00000000000098055, -49.34583672932542697 ) ) ;
#3620=CARTESIAN_POINT ( 'NONE',  ( -1.387778780781445676E-14, 20.00000000000000000, 101.0000000000000568 ) ) ;
#3621=CONICAL_SURFACE ( 'NONE', #5416, 2.524999999999999467, 0.7853981633974482790 ) ;
#3622=CARTESIAN_POINT ( 'NONE',  ( 13.00000000000024336, -2.516660498395250745, 105.0000000000000142 ) ) ;
#3624=CARTESIAN_POINT ( 'NONE',  ( 19.80330599461103702, 22.93419722094642310, 60.57506235960030239 ) ) ;
#3634=AXIS2_PLACEMENT_3D ( 'NONE', #3461, #20534, #4836 ) ;
#3637=CARTESIAN_POINT ( 'NONE',  ( -34.99999999999980815, 40.00000000000000711, 57.52499999999922409 ) ) ;
#3640=CARTESIAN_POINT ( 'NONE',  ( 3.069013497901954324, 39.94370175202870854, 50.97148194424899970 ) ) ;
#3641=AXIS2_PLACEMENT_3D ( 'NONE', #12545, #21617, #18050 ) ;
#3644=CARTESIAN_POINT ( 'NONE',  ( -42.50000000000000711, -12.00000000000000000, -41.00000000000000000 ) ) ;
#3645=VECTOR ( 'NONE', #10787, 1000.000000000000000 ) ;
#3646=DIRECTION ( 'NONE',  ( -0.000000000000000000, -0.000000000000000000, 1.000000000000000000 ) ) ;
#3650=FACE_OUTER_BOUND ( 'NONE', #16599, .T. ) ;
#3651=CARTESIAN_POINT ( 'NONE',  ( -6.869664380963927286, 39.72569445733122961, 53.24677099177210948 ) ) ;
#3655=ORIENTED_EDGE ( 'NONE', *, *, #10356, .F. ) ;
#3656=ORIENTED_EDGE ( 'NONE', *, *, #4032, .T. ) ;
#3657=CIRCLE ( 'NONE', #5117, 2.499999999999995115 ) ;
#3658=EDGE_CURVE ( 'NONE', #20269, #105, #12927, .T. ) ;
#3661=DIRECTION ( 'NONE',  ( 0.000000000000000000, 0.000000000000000000, -1.000000000000000000 ) ) ;
#3663=CARTESIAN_POINT ( 'NONE',  ( 15.99999999999991651, 20.00000000000000000, 102.0000000000000142 ) ) ;
#3670=CARTESIAN_POINT ( 'NONE',  ( -10.49999999999980460, -2.516660498395516310, 100.0000000000000000 ) ) ;
#3673=DIRECTION ( 'NONE',  ( -0.000000000000000000, 1.000000000000000000, -0.000000000000000000 ) ) ;
#3674=DIRECTION ( 'NONE',  ( 0.000000000000000000, 0.000000000000000000, -1.000000000000000000 ) ) ;
#3675=EDGE_LOOP ( 'NONE', ( #17661, #14381, #14341 ) ) ;
#3676=DIRECTION ( 'NONE',  ( 0.000000000000000000, 0.000000000000000000, -1.000000000000000000 ) ) ;
#3677=DIRECTION ( 'NONE',  ( 0.000000000000000000, 0.000000000000000000, -1.000000000000000000 ) ) ;
#3684=EDGE_CURVE ( 'NONE', #1286, #9683, #16381, .T. ) ;
#3688=VERTEX_POINT ( 'NONE', #696 ) ;
#3691=ORIENTED_EDGE ( 'NONE', *, *, #22016, .F. ) ;
#3696=DIRECTION ( 'NONE',  ( -1.000000000000000000, 0.000000000000000000, 0.000000000000000000 ) ) ;
#3697=ORIENTED_EDGE ( 'NONE', *, *, #21032, .T. ) ;
#3698=DIRECTION ( 'NONE',  ( 0.000000000000000000, 0.000000000000000000, 1.000000000000000000 ) ) ;
#3700=CARTESIAN_POINT ( 'NONE',  ( -2.098978802144722877, 39.97352552835178585, -50.29629877501648849 ) ) ;
#3704=CARTESIAN_POINT ( 'NONE',  ( -35.00000000000058265, 40.00000000000000711, -57.52500000000076597 ) ) ;
#3708=ORIENTED_EDGE ( 'NONE', *, *, #13091, .T. ) ;
#3713=CARTESIAN_POINT ( 'NONE',  ( 4.995691471223772773, 39.84469977656465289, -52.21048576823625353 ) ) ;
#3714=CARTESIAN_POINT ( 'NONE',  ( 1.679961057847793704, 39.99999999999999289, 49.78369069256650192 ) ) ;
#3717=DIRECTION ( 'NONE',  ( -0.000000000000000000, 1.000000000000000000, -0.000000000000000000 ) ) ;
#3718=ORIENTED_EDGE ( 'NONE', *, *, #17841, .T. ) ;
#3720=CARTESIAN_POINT ( 'NONE',  ( -18.83430946916727322, 32.25183488571026658, -57.78319592314316822 ) ) ;
#3724=ORIENTED_EDGE ( 'NONE', *, *, #1340, .F. ) ;
#3726=CARTESIAN_POINT ( 'NONE',  ( -0.6233897118003940419, 39.99089506582289744, 49.47139888151596665 ) ) ;
#3728=EDGE_CURVE ( 'NONE', #4117, #15875, #11441, .T. ) ;
#3729=CARTESIAN_POINT ( 'NONE',  ( 19.65511384563453490, 23.80142929986463329, 60.53962097676932075 ) ) ;
#3734=VERTEX_POINT ( 'NONE', #13488 ) ;
#3735=ADVANCED_FACE ( 'NONE', ( #1246 ), #8465, .F. ) ;
#3737=EDGE_LOOP ( 'NONE', ( #6138, #7809 ) ) ;
#3739=ORIENTED_EDGE ( 'NONE', *, *, #7664, .T. ) ;
#3740=DIRECTION ( 'NONE',  ( 0.000000000000000000, 0.000000000000000000, -1.000000000000000000 ) ) ;
#3745=CARTESIAN_POINT ( 'NONE',  ( 0.01154789369496759741, 39.99999926358022861, 48.74295989195564971 ) ) ;
#3747=CARTESIAN_POINT ( 'NONE',  ( 9.857944917841363619, 0.2919354798322448263, -54.29891737064843937 ) ) ;
#3750=DIRECTION ( 'NONE',  ( 0.000000000000000000, -1.000000000000000000, 0.000000000000000000 ) ) ;
#3751=CARTESIAN_POINT ( 'NONE',  ( -8.916870955515580732, 2.080241304161461358, -56.50845996868350340 ) ) ;
#3760=VERTEX_POINT ( 'NONE', #17389 ) ;
#3762=CONICAL_SURFACE ( 'NONE', #2281, 2.099999999999997868, 1.029744258676653867 ) ;
#3764=CARTESIAN_POINT ( 'NONE',  ( 11.12223430625389753, 40.00000000000000000, -54.01173000072967056 ) ) ;
#3769=CARTESIAN_POINT ( 'NONE',  ( -20.00000000000001421, 20.00000000000000355, 60.62177826491070931 ) ) ;
#3770=CARTESIAN_POINT ( 'NONE',  ( -10.50000000000012079, 42.51666049839536043, -105.0010000000000048 ) ) ;
#3773=CARTESIAN_POINT ( 'NONE',  ( -20.00000000000001421, 20.00000000000000355, 98.00000000000000000 ) ) ;
#3774=CARTESIAN_POINT ( 'NONE',  ( -35.00000000000058265, 28.00000000000000000, -55.00000000000076028 ) ) ;
#3775=CARTESIAN_POINT ( 'NONE',  ( 35.00000000000000000, 0.000000000000000000, 4.258610482196280173E-15 ) ) ;
#3781=CARTESIAN_POINT ( 'NONE',  ( 14.69246073108732631, 6.394048232432887779, -56.48929660089486049 ) ) ;
#3786=CARTESIAN_POINT ( 'NONE',  ( 0.09368790929011092117, 39.99996055670441564, -48.80680027770784335 ) ) ;
#3791=VERTEX_POINT ( 'NONE', #8576 ) ;
#3793=AXIS2_PLACEMENT_3D ( 'NONE', #3218, #6646, #4821 ) ;
#3794=CARTESIAN_POINT ( 'NONE',  ( -7.531924820109092700, 39.99999999999999289, 52.77310267448202552 ) ) ;
#3798=CARTESIAN_POINT ( 'NONE',  ( 22.32664865868312276, 17.89874346835044960, -58.64628984943159651 ) ) ;
#3799=CARTESIAN_POINT ( 'NONE',  ( -1.387778780781445518E-14, 20.00000000000000355, 102.0000000000000142 ) ) ;
#3800=ORIENTED_EDGE ( 'NONE', *, *, #4187, .T. ) ;
#3802=CARTESIAN_POINT ( 'NONE',  ( -11.68090480754625027, 3.765577839755239076, 57.90797000640172598 ) ) ;
#3803=CARTESIAN_POINT ( 'NONE',  ( -4.585174533585286483, 39.86909732232018655, -51.95486270304797216 ) ) ;
#3804=ADVANCED_FACE ( 'NONE', ( #15549 ), #9950, .T. ) ;
#3809=EDGE_CURVE ( 'NONE', #7645, #10705, #191, .T. ) ;
#3810=EDGE_CURVE ( 'NONE', #6428, #19994, #12129, .T. ) ;
#3811=CIRCLE ( 'NONE', #21753, 2.499999999999995115 ) ;
#3817=CARTESIAN_POINT ( 'NONE',  ( -42.50000000000000711, -12.00000000000012434, 50.02500000000011937 ) ) ;
#3818=FACE_OUTER_BOUND ( 'NONE', #18240, .T. ) ;
#3820=CARTESIAN_POINT ( 'NONE',  ( 9.952189117650823036, 40.00000000000000000, 53.64426396172073197 ) ) ;
#3824=LINE ( 'NONE', #4059, #3645 ) ;
#3828=CARTESIAN_POINT ( 'NONE',  ( -20.16756852208517259, 29.88972976525007397, -58.13897502025236719 ) ) ;
#3829=CARTESIAN_POINT ( 'NONE',  ( -35.00000000000058265, 40.00000000000000000, -52.50000000000076739 ) ) ;
#3834=EDGE_CURVE ( 'NONE', #4643, #16803, #18900, .T. ) ;
#3839=CARTESIAN_POINT ( 'NONE',  ( 18.64599517736090917, 12.71385791664973652, 57.77541544179720745 ) ) ;
#3840=FACE_OUTER_BOUND ( 'NONE', #12988, .T. ) ;
#3841=EDGE_CURVE ( 'NONE', #12228, #4040, #14716, .T. ) ;
#3842=CARTESIAN_POINT ( 'NONE',  ( 9.165377225651162973, 37.79989650906289711, -54.16098472236620864 ) ) ;
#3844=CIRCLE ( 'NONE', #14432, 2.499999999999998668 ) ;
#3850=DIRECTION ( 'NONE',  ( 0.000000000000000000, 0.000000000000000000, 1.000000000000000000 ) ) ;
#3851=EDGE_CURVE ( 'NONE', #4605, #17185, #19492, .T. ) ;
#3853=CARTESIAN_POINT ( 'NONE',  ( 0.3255751848036408935, 39.99938829199252410, 48.98576722398500038 ) ) ;
#3854=CIRCLE ( 'NONE', #9697, 10.00000000000000178 ) ;
#3862=DIRECTION ( 'NONE',  ( -0.000000000000000000, -1.000000000000000000, -0.000000000000000000 ) ) ;
#3863=AXIS2_PLACEMENT_3D ( 'NONE', #10380, #6970, #77 ) ;
#3867=LINE ( 'NONE', #7409, #15598 ) ;
#3875=AXIS2_PLACEMENT_3D ( 'NONE', #16531, #16874, #2678 ) ;
#3878=CARTESIAN_POINT ( 'NONE',  ( 42.50000000000000711, -12.00000000000000000, 45.40000000000001279 ) ) ;
#3880=DIRECTION ( 'NONE',  ( -0.000000000000000000, 1.000000000000000000, -0.000000000000000000 ) ) ;
#3882=DIRECTION ( 'NONE',  ( 0.7752116086454778898, 0.5577761202038522548, 0.2965345874457622211 ) ) ;
#3883=CARTESIAN_POINT ( 'NONE',  ( -12.30135915900901011, 4.212003844039742262, 58.16904039079302180 ) ) ;
#3884=CIRCLE ( 'NONE', #6453, 10.00000000000000178 ) ;
#3885=CARTESIAN_POINT ( 'NONE',  ( -12.72045107882562220, 38.45933137995365314, -55.71167848415556278 ) ) ;
#3890=FACE_BOUND ( 'NONE', #11880, .T. ) ;
#3892=CARTESIAN_POINT ( 'NONE',  ( 12.68897045256291811, 11.99170770793163321, -44.74667050109238176 ) ) ;
#3893=EDGE_CURVE ( 'NONE', #19116, #6177, #17051, .T. ) ;
#3897=DIRECTION ( 'NONE',  ( -0.000000000000000000, 1.000000000000000000, -0.000000000000000000 ) ) ;
#3898=CARTESIAN_POINT ( 'NONE',  ( 35.00000000000000000, 40.00000000000000000, 4.258610482196280173E-15 ) ) ;
#3901=AXIS2_PLACEMENT_3D ( 'NONE', #297, #14690, #5237 ) ;
#3902=ORIENTED_EDGE ( 'NONE', *, *, #12487, .F. ) ;
#3903=VECTOR ( 'NONE', #1289, 1000.000000000000000 ) ;
#3905=VERTEX_POINT ( 'NONE', #15887 ) ;
#3911=CARTESIAN_POINT ( 'NONE',  ( -6.094648662765727920, 40.00000000000000000, 52.13898825983068974 ) ) ;
#3912=EDGE_LOOP ( 'NONE', ( #4536, #17484, #16535, #851 ) ) ;
#3915=CARTESIAN_POINT ( 'NONE',  ( 19.46387463785189809, 8.808008015900604448, -57.95411844647834698 ) ) ;
#3921=EDGE_CURVE ( 'NONE', #6468, #19936, #14844, .T. ) ;
#3923=CARTESIAN_POINT ( 'NONE',  ( 12.84005703549854616, 1.693876179613353017, 55.76322220629359094 ) ) ;
#3926=AXIS2_PLACEMENT_3D ( 'NONE', #15020, #12966, #733 ) ;
#3927=EDGE_CURVE ( 'NONE', #3415, #8689, #19240, .T. ) ;
#3928=VERTEX_POINT ( 'NONE', #7081 ) ;
#3931=ORIENTED_EDGE ( 'NONE', *, *, #17148, .F. ) ;
#3934=CARTESIAN_POINT ( 'NONE',  ( 19.99999999999998579, 20.00000000000000000, 60.62177826491070221 ) ) ;
#3936=CARTESIAN_POINT ( 'NONE',  ( -3.777351397511341336E-15, 39.99999999999997158, -48.73397172404481381 ) ) ;
#3937=CARTESIAN_POINT ( 'NONE',  ( 7.287850628716163293, 40.00000000000000711, 52.67053206792662934 ) ) ;
#3941=VERTEX_POINT ( 'NONE', #425 ) ;
#3943=CARTESIAN_POINT ( 'NONE',  ( -22.41121774633938912, 19.23761757294739283, -58.66449182057564116 ) ) ;
#3945=DIRECTION ( 'NONE',  ( 0.000000000000000000, 0.7071067811865474617, 0.7071067811865474617 ) ) ;
#3946=ORIENTED_EDGE ( 'NONE', *, *, #3921, .T. ) ;
#3949=VERTEX_POINT ( 'NONE', #1927 ) ;
#3951=FACE_OUTER_BOUND ( 'NONE', #17332, .T. ) ;
#3957=CARTESIAN_POINT ( 'NONE',  ( 18.02527238916047381, 28.84533800490727629, 60.11925852858798436 ) ) ;
#3960=CARTESIAN_POINT ( 'NONE',  ( 13.23602284716676358, 35.01773851405933868, -58.53880247431292361 ) ) ;
#3961=EDGE_LOOP ( 'NONE', ( #12443, #21933, #14021, #5013 ) ) ;
#3962=EDGE_LOOP ( 'NONE', ( #5065, #20527 ) ) ;
#3965=B_SPLINE_CURVE_WITH_KNOTS ( 'NONE', 3,
 ( #1586, #10053, #17165, #20732, #4918, #17273, #20502, #5036, #8463, #12021, #13834, #3429, #17054, #15432, #19015, #1478, #18780, #20394, #6747, #18898, #8575, #11893 ),
 .UNSPECIFIED., .F., .F.,
 ( 4, 2, 2, 2, 2, 2, 2, 2, 2, 2, 4 ),
 ( 0.007712149587921395336, 0.01231940472852629045, 0.01347121851367751727, 0.01462303229882874062, 0.01692665986913119425, 0.01807847365428242453, 0.01923028743943365482, 0.02153391500973611539, 0.02268572879488733873, 0.02383754258003856208, 0.02614117015034102265 ),
 .UNSPECIFIED. ) ;
#3968=CARTESIAN_POINT ( 'NONE',  ( 42.50000000000000711, -12.00000000000000000, -47.50000000000000000 ) ) ;
#3969=CARTESIAN_POINT ( 'NONE',  ( -10.81645871527333114, 39.16817317915248253, -54.94897387134643196 ) ) ;
#3971=CARTESIAN_POINT ( 'NONE',  ( -1.387778780781445518E-14, 20.00000000000000355, -105.0000000000000142 ) ) ;
#3972=CIRCLE ( 'NONE', #4330, 2.499999999999998668 ) ;
#3973=EDGE_LOOP ( 'NONE', ( #6740, #403, #15276, #5398 ) ) ;
#3975=DIRECTION ( 'NONE',  ( 0.000000000000000000, 1.000000000000000000, 0.000000000000000000 ) ) ;
#3980=CARTESIAN_POINT ( 'NONE',  ( 42.50000000000000711, -12.00000000000000000, 47.50000000000000711 ) ) ;
#3986=CARTESIAN_POINT ( 'NONE',  ( -5.702716825709945425, 39.17357718829533297, 54.58701425223461712 ) ) ;
#3987=EDGE_CURVE ( 'NONE', #4421, #6249, #15199, .T. ) ;
#3990=ORIENTED_EDGE ( 'NONE', *, *, #12780, .T. ) ;
#3992=EDGE_CURVE ( 'NONE', #11258, #922, #6090, .T. ) ;
#3995=( GEOMETRIC_REPRESENTATION_CONTEXT ( 3 ) GLOBAL_UNCERTAINTY_ASSIGNED_CONTEXT ( ( #5978 ) ) GLOBAL_UNIT_ASSIGNED_CONTEXT ( ( #6729, #21162, #15867 ) ) REPRESENTATION_CONTEXT ( 'NONE', 'WORKASPACE' ) );
#3998=CARTESIAN_POINT ( 'NONE',  ( 5.511499161258694102, 0.6970817516955201132, -52.42185088606010623 ) ) ;
#4002=CARTESIAN_POINT ( 'NONE',  ( -15.39832585462821868, 32.77960222724827588, -56.73873823673314831 ) ) ;
#4008=FACE_BOUND ( 'NONE', #9604, .T. ) ;
#4009=CARTESIAN_POINT ( 'NONE',  ( -3.210598435713526211, 39.75302854575187439, -52.30739040051270905 ) ) ;
#4016=EDGE_CURVE ( 'NONE', #14214, #8612, #16697, .T. ) ;
#4020=CARTESIAN_POINT ( 'NONE',  ( 14.30107462755360537, 5.991811841696046415, -58.93430465799249163 ) ) ;
#4021=ADVANCED_FACE ( 'NONE', ( #18302 ), #4564, .F. ) ;
#4026=EDGE_CURVE ( 'NONE', #22156, #7926, #19958, .T. ) ;
#4027=ORIENTED_EDGE ( 'NONE', *, *, #17960, .T. ) ;
#4029=FACE_OUTER_BOUND ( 'NONE', #21345, .T. ) ;
#4032=EDGE_CURVE ( 'NONE', #6302, #8864, #2842, .T. ) ;
#4034=CARTESIAN_POINT ( 'NONE',  ( -8.219889501007404675, 1.750964516535594040, -56.08920281152427378 ) ) ;
#4035=ORIENTED_EDGE ( 'NONE', *, *, #19026, .T. ) ;
#4038=CARTESIAN_POINT ( 'NONE',  ( -9.505536299094565322, 39.99999999999999289, 53.50900092114397921 ) ) ;
#4040=VERTEX_POINT ( 'NONE', #11316 ) ;
#4042=CARTESIAN_POINT ( 'NONE',  ( -8.219889500999224552, 1.750964516532281356, 56.08920281153879017 ) ) ;
#4043=CARTESIAN_POINT ( 'NONE',  ( -0.2640866027062644950, 39.99958921875370521, -48.93844571589828263 ) ) ;
#4046=DIRECTION ( 'NONE',  ( 0.000000000000000000, 1.000000000000000000, 0.000000000000000000 ) ) ;
#4047=ORIENTED_EDGE ( 'NONE', *, *, #9212, .T. ) ;
#4048=ORIENTED_EDGE ( 'NONE', *, *, #12656, .F. ) ;
#4049=EDGE_LOOP ( 'NONE', ( #12134, #11751 ) ) ;
#4054=AXIS2_PLACEMENT_3D ( 'NONE', #11963, #3274, #19190 ) ;
#4055=CARTESIAN_POINT ( 'NONE',  ( 1.486416059063909278, 39.99051308249325842, -49.86506293652772115 ) ) ;
#4056=EDGE_CURVE ( 'NONE', #18787, #13935, #2382, .T. ) ;
#4058=ORIENTED_EDGE ( 'NONE', *, *, #10987, .F. ) ;
#4059=CARTESIAN_POINT ( 'NONE',  ( 5.833333333333329485, 40.00000000000000000, -40.61164310337066041 ) ) ;
#4065=CARTESIAN_POINT ( 'NONE',  ( 2.589862425843441063, 0.1394011931331439469, 50.61994180263811671 ) ) ;
#4066=EDGE_CURVE ( 'NONE', #18872, #19255, #4263, .T. ) ;
#4067=ORIENTED_EDGE ( 'NONE', *, *, #4272, .F. ) ;
#4068=CARTESIAN_POINT ( 'NONE',  ( 8.970852013922840484, 37.88903915979515347, 54.67447700193728366 ) ) ;
#4072=CARTESIAN_POINT ( 'NONE',  ( 22.20997089757253207, 23.22761694305071245, 58.62102808997010328 ) ) ;
#4075=CARTESIAN_POINT ( 'NONE',  ( 13.87722263113801802, 34.42803545437053003, -58.77926695580346461 ) ) ;
#4076=ORIENTED_EDGE ( 'NONE', *, *, #7958, .F. ) ;
#4077=EDGE_CURVE ( 'NONE', #12705, #3042, #13810, .T. ) ;
#4078=ORIENTED_EDGE ( 'NONE', *, *, #22403, .T. ) ;
#4079=ORIENTED_EDGE ( 'NONE', *, *, #14617, .F. ) ;
#4082=CARTESIAN_POINT ( 'NONE',  ( -10.08226496024166430, 39.27879523455747091, -54.68359763800749818 ) ) ;
#4083=CARTESIAN_POINT ( 'NONE',  ( -34.99999999999980815, 40.00000000000000711, 54.99999999999922551 ) ) ;
#4084=ORIENTED_EDGE ( 'NONE', *, *, #12745, .F. ) ;
#4086=CARTESIAN_POINT ( 'NONE',  ( -3.235223465815322719, -4.647308930658608617, 47.76313845446109951 ) ) ;
#4087=ORIENTED_EDGE ( 'NONE', *, *, #17634, .F. ) ;
#4088=DIRECTION ( 'NONE',  ( -0.000000000000000000, -1.000000000000000000, -0.000000000000000000 ) ) ;
#4090=DIRECTION ( 'NONE',  ( -0.000000000000000000, 1.000000000000000000, -0.000000000000000000 ) ) ;
#4091=DIRECTION ( 'NONE',  ( -0.000000000000000000, -0.000000000000000000, -1.000000000000000000 ) ) ;
#4092=CARTESIAN_POINT ( 'NONE',  ( 35.00000000000058265, 39.97500000000000142, -55.00000000000076028 ) ) ;
#4094=CIRCLE ( 'NONE', #9200, 2.099999999999997868 ) ;
#4095=DIRECTION ( 'NONE',  ( -0.000000000000000000, -0.000000000000000000, -1.000000000000000000 ) ) ;
#4098=ADVANCED_FACE ( 'NONE', ( #16922 ), #20728, .T. ) ;
#4100=ORIENTED_EDGE ( 'NONE', *, *, #6274, .F. ) ;
#4103=CARTESIAN_POINT ( 'NONE',  ( 4.664549341139476724, 0.4975632029830715508, -53.81030450292873013 ) ) ;
#4104=AXIS2_PLACEMENT_3D ( 'NONE', #11985, #5007, #5229 ) ;
#4105=EDGE_CURVE ( 'NONE', #16638, #11727, #16321, .T. ) ;
#4108=CARTESIAN_POINT ( 'NONE',  ( -2.039347869096966038E-14, 40.00000000000000000, -48.73397172404482092 ) ) ;
#4111=ORIENTED_EDGE ( 'NONE', *, *, #13673, .T. ) ;
#4112=FACE_BOUND ( 'NONE', #15145, .T. ) ;
#4113=CARTESIAN_POINT ( 'NONE',  ( -42.50000000000000711, -12.00000000000000000, -47.50000000000000000 ) ) ;
#4115=EDGE_CURVE ( 'NONE', #19351, #5750, #19686, .T. ) ;
#4117=VERTEX_POINT ( 'NONE', #7716 ) ;
#4119=CYLINDRICAL_SURFACE ( 'NONE', #9690, 2.499999999999996891 ) ;
#4124=CARTESIAN_POINT ( 'NONE',  ( -90.00000000000000000, 26.00000000000000355, 2.099999999999989875 ) ) ;
#4125=CYLINDRICAL_SURFACE ( 'NONE', #9423, 2.500000000000002220 ) ;
#4127=CARTESIAN_POINT ( 'NONE',  ( 9.177445128772406591, 39.41890422686074658, -54.36989725583298849 ) ) ;
#4129=EDGE_CURVE ( 'NONE', #10068, #18626, #8283, .T. ) ;
#4130=DIRECTION ( 'NONE',  ( 0.000000000000000000, 0.000000000000000000, -1.000000000000000000 ) ) ;
#4131=VERTEX_POINT ( 'NONE', #19979 ) ;
#4134=ORIENTED_EDGE ( 'NONE', *, *, #12249, .F. ) ;
#4138=EDGE_LOOP ( 'NONE', ( #20614, #21838 ) ) ;
#4140=DIRECTION ( 'NONE',  ( 0.000000000000000000, 0.000000000000000000, 1.000000000000000000 ) ) ;
#4141=ADVANCED_FACE ( 'NONE', ( #20938 ), #10486, .F. ) ;
#4143=CARTESIAN_POINT ( 'NONE',  ( -4.273193112870391275, 39.88698587828563547, -51.75894944362807593 ) ) ;
#4145=EDGE_CURVE ( 'NONE', #18626, #6724, #12968, .T. ) ;
#4149=DIRECTION ( 'NONE',  ( -1.000000000000000000, 0.000000000000000000, 0.000000000000000000 ) ) ;
#4152=AXIS2_PLACEMENT_3D ( 'NONE', #12645, #16201, #511 ) ;
#4156=ORIENTED_EDGE ( 'NONE', *, *, #19194, .F. ) ;
#4158=DIRECTION ( 'NONE',  ( -0.000000000000000000, -0.000000000000000000, -1.000000000000000000 ) ) ;
#4159=CARTESIAN_POINT ( 'NONE',  ( 1.387778780781445676E-14, 40.00000000000000000, 48.73397172404482802 ) ) ;
#4160=DIRECTION ( 'NONE',  ( -0.000000000000000000, -0.000000000000000000, 1.000000000000000000 ) ) ;
#4161=CARTESIAN_POINT ( 'NONE',  ( 10.49999999999994316, 42.51666049839543149, -105.0010000000000048 ) ) ;
#4167=CARTESIAN_POINT ( 'NONE',  ( 10.50000000000024514, -2.516660498395250301, 105.0000000000000142 ) ) ;
#4170=CARTESIAN_POINT ( 'NONE',  ( 19.99999999999998579, 20.00000000000000355, -98.00000000000000000 ) ) ;
#4172=CARTESIAN_POINT ( 'NONE',  ( 6.869621667053231739, 39.72564009089534665, 53.24680777370071638 ) ) ;
#4178=DIRECTION ( 'NONE',  ( 0.000000000000000000, 0.000000000000000000, 1.000000000000000000 ) ) ;
#4179=CARTESIAN_POINT ( 'NONE',  ( -15.50000000000011013, 42.51666049839536043, 105.0000000000000142 ) ) ;
#4183=EDGE_CURVE ( 'NONE', #3398, #20205, #13753, .T. ) ;
#4184=FACE_BOUND ( 'NONE', #8347, .T. ) ;
#4187=EDGE_CURVE ( 'NONE', #7505, #2375, #5722, .T. ) ;
#4188=ORIENTED_EDGE ( 'NONE', *, *, #14281, .T. ) ;
#4190=CARTESIAN_POINT ( 'NONE',  ( -1.387778780781445676E-14, 20.00000000000000000, -100.0000000000000000 ) ) ;
#4191=CARTESIAN_POINT ( 'NONE',  ( -10.49999999999980460, -2.516660498395516310, -105.0010000000000048 ) ) ;
#4193=DIRECTION ( 'NONE',  ( 0.000000000000000000, 0.000000000000000000, 1.000000000000000000 ) ) ;
#4195=CARTESIAN_POINT ( 'NONE',  ( -10.43027093729396526, 39.22757009021463404, -54.80615623442352558 ) ) ;
#4197=CIRCLE ( 'NONE', #22478, 15.99999999999998579 ) ;
#4199=CARTESIAN_POINT ( 'NONE',  ( 11.99035502499705430, 39.33333333333332860, -55.05149724789898613 ) ) ;
#4203=AXIS2_PLACEMENT_3D ( 'NONE', #4400, #9886, #4511 ) ;
#4206=CARTESIAN_POINT ( 'NONE',  ( -3.244689583143795186, 39.74755540027226886, 52.34195286440937167 ) ) ;
#4212=CARTESIAN_POINT ( 'NONE',  ( 35.00000000000000000, 40.00000000000000000, 4.258610482196280173E-15 ) ) ;
#4215=CARTESIAN_POINT ( 'NONE',  ( 0.1564864144766087983, 40.00000000000000000, 48.92140276528778031 ) ) ;
#4217=CARTESIAN_POINT ( 'NONE',  ( -5.617742387210350685, 39.81211049013471381, -52.56498094152444622 ) ) ;
#4220=DIRECTION ( 'NONE',  ( -1.000000000000000000, 0.000000000000000000, 0.000000000000000000 ) ) ;
#4223=B_SPLINE_CURVE_WITH_KNOTS ( 'NONE', 3,
 ( #9534, #8153, #20307, #7810, #2895, #18345, #15118, #9425, #4386, #11361, #7932, #2665 ),
 .UNSPECIFIED., .F., .F.,
 ( 4, 1, 1, 1, 1, 2, 2, 4 ),
 ( 0.000000000000000000, 0.2499999999999911182, 0.3749999999999869549, 0.4374999999999852340, 0.4687499999999832911, 0.4843749999999822919, 0.4999999999999812927, 1.000000000000000000 ),
 .UNSPECIFIED. ) ;
#4233=DIRECTION ( 'NONE',  ( 0.000000000000000000, -1.000000000000000000, 0.000000000000000000 ) ) ;
#4234=LINE ( 'NONE', #7670, #19621 ) ;
#4237=DIRECTION ( 'NONE',  ( 0.000000000000000000, 0.000000000000000000, -1.000000000000000000 ) ) ;
#4238=CARTESIAN_POINT ( 'NONE',  ( 2.478389530992044065, 40.00000000000000000, -50.25195279936158954 ) ) ;
#4239=CIRCLE ( 'NONE', #13000, 2.524999999999999467 ) ;
#4240=ADVANCED_FACE ( 'NONE', ( #7170 ), #7604, .F. ) ;
#4241=ORIENTED_EDGE ( 'NONE', *, *, #4066, .T. ) ;
#4242=CARTESIAN_POINT ( 'NONE',  ( 2.105505840716530574, 39.97335763330380587, -50.30092836639100540 ) ) ;
#4248=ORIENTED_EDGE ( 'NONE', *, *, #22394, .T. ) ;
#4251=LINE ( 'NONE', #5961, #22162 ) ;
#4252=EDGE_CURVE ( 'NONE', #22506, #2582, #20413, .T. ) ;
#4253=AXIS2_PLACEMENT_3D ( 'NONE', #11439, #2743, #2635 ) ;
#4255=ORIENTED_EDGE ( 'NONE', *, *, #18899, .T. ) ;
#4256=DIRECTION ( 'NONE',  ( -0.000000000000000000, 1.000000000000000000, -0.000000000000000000 ) ) ;
#4258=CARTESIAN_POINT ( 'NONE',  ( -0.1139232394121202224, 39.99992693198588967, -48.82246310442314297 ) ) ;
#4261=CARTESIAN_POINT ( 'NONE',  ( -1.387778780781445676E-14, 20.00000000000000000, -101.0000000000000284 ) ) ;
#4263=CIRCLE ( 'NONE', #22573, 49.99999999999998579 ) ;
#4264=CONICAL_SURFACE ( 'NONE', #6831, 2.099999999999997868, 1.029744258676652091 ) ;
#4267=VERTEX_POINT ( 'NONE', #7059 ) ;
#4272=EDGE_CURVE ( 'NONE', #17695, #862, #16420, .T. ) ;
#4277=FACE_OUTER_BOUND ( 'NONE', #19436, .T. ) ;
#4278=CARTESIAN_POINT ( 'NONE',  ( 1.833353995796188407, 5.110175324539462771, -38.89995731584652106 ) ) ;
#4279=ORIENTED_EDGE ( 'NONE', *, *, #5478, .T. ) ;
#4283=CARTESIAN_POINT ( 'NONE',  ( -11.84374239103370741, 10.78799321809639800, -44.31542800769554447 ) ) ;
#4286=CARTESIAN_POINT ( 'NONE',  ( 19.99999999999998579, 20.00000000000000711, -60.62177826491069510 ) ) ;
#4287=ORIENTED_EDGE ( 'NONE', *, *, #20018, .T. ) ;
#4290=ORIENTED_EDGE ( 'NONE', *, *, #3552, .F. ) ;
#4291=CARTESIAN_POINT ( 'NONE',  ( 8.957563853402323417, 39.56956388360624288, 54.21303480198576352 ) ) ;
#4292=EDGE_CURVE ( 'NONE', #8817, #18681, #6505, .T. ) ;
#4306=EDGE_LOOP ( 'NONE', ( #6372, #8866, #818, #13623 ) ) ;
#4310=( BOUNDED_SURFACE ( )  B_SPLINE_SURFACE ( 3, 2, ( 
 ( #1485, #8363, #10061 ),
 ( #4925, #8469, #15438 ),
 ( #4816, #15332, #17171 ),
 ( #6639, #22350, #13599 ),
 ( #18905, #3212, #22460 ),
 ( #10178, #6756, #13492 ),
 ( #18786, #20509, #3091 ),
 ( #1367, #2832, #8212 ),
 ( #21978, #13568, #18645 ),
 ( #14837, #16807, #4442 ),
 ( #15171, #4783, #994 ),
 ( #15296, #7993, #22320 ),
 ( #16689, #22081, #20138 ),
 ( #2950, #9819, #6604 ),
 ( #878, #18748, #17020 ),
 ( #6268, #16912, #14953 ),
 ( #11754, #11416, #1330 ),
 ( #1112, #8321, #9699 ),
 ( #3054, #16572, #20580 ),
 ( #10028, #7870, #9924 ),
 ( #20476, #11308, #18297 ),
 ( #13124, #9585, #2609 ),
 ( #4555, #21860, #6160 ),
 ( #18400, #22197, #6375 ),
 ( #13227, #20248, #11534 ),
 ( #2723, #18521, #13338 ),
 ( #8103, #15061, #1212 ),
 ( #20365, #4667, #6489 ),
 ( #11646, #13456, #1450 ),
 ( #3400, #7160, #10479 ),
 ( #8435, #13681, #6952 ),
 ( #10255, #8879, #15405 ) ),
 .UNSPECIFIED., .F., .F., .F. ) 
 B_SPLINE_SURFACE_WITH_KNOTS ( ( 4, 2, 2, 2, 2, 2, 2, 2, 2, 2, 2, 2, 2, 2, 2, 4 ),
 ( 3, 3 ),
 ( 0.000000000000000000, 0.005810029919203039614, 0.008715044878804558554, 0.01162005983840607923, 0.01452507479800759817, 0.01743008975760911711, 0.02033510471721063778, 0.02324011967681215846, 0.02614513463641367913, 0.02905014959601519633, 0.03486017951521823421, 0.03631268699501899455, 0.03776519447481975489, 0.04067020943442127556, 0.04357522439402279624, 0.04648023935362431691 ),
 ( 0.000000000000000000, 1.000000000000000000 ),
 .UNSPECIFIED. ) 
 GEOMETRIC_REPRESENTATION_ITEM ( )  RATIONAL_B_SPLINE_SURFACE ( (
 ( 1.000000000000000000, 0.6428092274089118874, 1.000000000000000000),
 ( 1.000000000000000000, 0.6349692141176791482, 1.000000000000000000),
 ( 1.000000000000000000, 0.6297610438357627016, 1.000000000000000000),
 ( 1.000000000000000000, 0.6250724677584068578, 1.000000000000000000),
 ( 1.000000000000000000, 0.6240291009521158339, 1.000000000000000000),
 ( 1.000000000000000000, 0.6228114827670508946, 1.000000000000000000),
 ( 1.000000000000000000, 0.6226217323249613189, 1.000000000000000000),
 ( 1.000000000000000000, 0.6227877533346651839, 1.000000000000000000),
 ( 1.000000000000000000, 0.6231437405068817048, 1.000000000000000000),
 ( 1.000000000000000000, 0.6241327156851853575, 1.000000000000000000),
 ( 1.000000000000000000, 0.6247528374331501322, 1.000000000000000000),
 ( 1.000000000000000000, 0.6259854008234480016, 1.000000000000000000),
 ( 1.000000000000000000, 0.6265990906533466243, 1.000000000000000000),
 ( 1.000000000000000000, 0.6276348137172499397, 1.000000000000000000),
 ( 1.000000000000000000, 0.6280565648727459704, 1.000000000000000000),
 ( 1.000000000000000000, 0.6285705475697730416, 1.000000000000000000),
 ( 1.000000000000000000, 0.6286676444199297276, 1.000000000000000000),
 ( 1.000000000000000000, 0.6285219413518228215, 1.000000000000000000),
 ( 1.000000000000000000, 0.6282782847626313671, 1.000000000000000000),
 ( 1.000000000000000000, 0.6271139948532048480, 1.000000000000000000),
 ( 1.000000000000000000, 0.6257653971626693234, 1.000000000000000000),
 ( 1.000000000000000000, 0.6242767683748037255, 1.000000000000000000),
 ( 1.000000000000000000, 0.6239908339060202813, 1.000000000000000000),
 ( 1.000000000000000000, 0.6234800620765024171, 1.000000000000000000),
 ( 1.000000000000000000, 0.6232570855776793373, 1.000000000000000000),
 ( 1.000000000000000000, 0.6227348070543635705, 1.000000000000000000),
 ( 1.000000000000000000, 0.6225812994814358126, 1.000000000000000000),
 ( 1.000000000000000000, 0.6229454059004365662, 1.000000000000000000),
 ( 1.000000000000000000, 0.6234652178690811564, 1.000000000000000000),
 ( 1.000000000000000000, 0.6254772350196486919, 1.000000000000000000),
 ( 1.000000000000000000, 0.6269570472271859263, 1.000000000000000000),
 ( 1.000000000000000000, 0.6290213284793358950, 1.000000000000000000) ) ) 
 REPRESENTATION_ITEM ( '' )  SURFACE ( )  );
#4319=CIRCLE ( 'NONE', #8324, 17.00000000000001421 ) ;
#4323=ADVANCED_FACE ( 'NONE', ( #3818 ), #19854, .F. ) ;
#4324=DIRECTION ( 'NONE',  ( -0.000000000000000000, -1.000000000000000000, -0.000000000000000000 ) ) ;
#4326=CARTESIAN_POINT ( 'NONE',  ( 42.50000000000000711, -12.00000000000012434, 47.50000000000000711 ) ) ;
#4327=ORIENTED_EDGE ( 'NONE', *, *, #16684, .F. ) ;
#4330=AXIS2_PLACEMENT_3D ( 'NONE', #7171, #3646, #20939 ) ;
#4331=ORIENTED_EDGE ( 'NONE', *, *, #21833, .T. ) ;
#4334=CARTESIAN_POINT ( 'NONE',  ( 1.145276119298441975, 0.005126887280125313681, -49.65522505679928855 ) ) ;
#4336=AXIS2_PLACEMENT_3D ( 'NONE', #20180, #18000, #19844 ) ;
#4339=DIRECTION ( 'NONE',  ( 0.000000000000000000, 0.000000000000000000, -1.000000000000000000 ) ) ;
#4342=AXIS2_PLACEMENT_3D ( 'NONE', #21017, #9195, #16170 ) ;
#4346=AXIS2_PLACEMENT_3D ( 'NONE', #11743, #2939, #8530 ) ;
#4347=CARTESIAN_POINT ( 'NONE',  ( 13.00000000000024336, -2.516660498395250745, -100.0000000000000000 ) ) ;
#4350=CIRCLE ( 'NONE', #20817, 2.499999999999998668 ) ;
#4353=CARTESIAN_POINT ( 'NONE',  ( 90.00000000000000000, 40.00000000000000000, 2.099999999999989875 ) ) ;
#4360=DIRECTION ( 'NONE',  ( -0.000000000000000000, -1.000000000000000000, -0.000000000000000000 ) ) ;
#4361=ADVANCED_FACE ( 'NONE', ( #17786 ), #8962, .T. ) ;
#4364=CARTESIAN_POINT ( 'NONE',  ( 0.3359095670093927288, 39.99934629023403687, -48.99369681844596869 ) ) ;
#4367=DIRECTION ( 'NONE',  ( 0.000000000000000000, 0.000000000000000000, -1.000000000000000000 ) ) ;
#4369=CARTESIAN_POINT ( 'NONE',  ( -2.777956037036614756, 39.99999999999999289, 50.42551054490269991 ) ) ;
#4371=TOROIDAL_SURFACE ( 'NONE', #17158, 22.00000000000000000, 2.000000000000000000 ) ;
#4375=CARTESIAN_POINT ( 'NONE',  ( -0.03435155977924175819, 39.99999305009784223, -48.76069593537407343 ) ) ;
#4377=CARTESIAN_POINT ( 'NONE',  ( -11.84669267190940722, 29.23061840495885733, 44.31876460048059840 ) ) ;
#4382=EDGE_CURVE ( 'NONE', #21335, #16994, #6134, .T. ) ;
#4386=CARTESIAN_POINT ( 'NONE',  ( 11.09836907989742905, 40.00000000000000000, 54.00358115607141229 ) ) ;
#4389=CARTESIAN_POINT ( 'NONE',  ( -34.99999999999980815, 26.00000000000000355, 52.89999999999922409 ) ) ;
#4390=CARTESIAN_POINT ( 'NONE',  ( -5.011587927596626635, 5.833858253127846893, -40.02147800532274147 ) ) ;
#4394=ORIENTED_EDGE ( 'NONE', *, *, #17169, .F. ) ;
#4395=CARTESIAN_POINT ( 'NONE',  ( -8.188149873056877581, 7.413691783916331879, -42.20917188641858075 ) ) ;
#4398=CARTESIAN_POINT ( 'NONE',  ( 1.570149971351546103, 40.00000000000000000, 49.72616472077324801 ) ) ;
#4400=CARTESIAN_POINT ( 'NONE',  ( -1.387778780781445518E-14, 20.00000000000000355, 103.0000000000000284 ) ) ;
#4401=EDGE_CURVE ( 'NONE', #4117, #17014, #19680, .T. ) ;
#4402=CARTESIAN_POINT ( 'NONE',  ( 3.315551171824481003, 0.2472631163781295605, 51.08212483309238650 ) ) ;
#4404=CARTESIAN_POINT ( 'NONE',  ( 8.123071147678585291, 39.63120350560809868, 53.85470533195105958 ) ) ;
#4412=DIRECTION ( 'NONE',  ( 8.659560562355083235E-17, 0.7071067811865352493, -0.7071067811865597852 ) ) ;
#4413=CARTESIAN_POINT ( 'NONE',  ( 19.43475998741689281, 8.756352882854699260, -57.94642939675669169 ) ) ;
#4414=VERTEX_POINT ( 'NONE', #1161 ) ;
#4416=ORIENTED_EDGE ( 'NONE', *, *, #21182, .F. ) ;
#4420=DIRECTION ( 'NONE',  ( 0.000000000000000000, 0.000000000000000000, 1.000000000000000000 ) ) ;
#4421=VERTEX_POINT ( 'NONE', #6099 ) ;
#4424=ORIENTED_EDGE ( 'NONE', *, *, #18472, .F. ) ;
#4427=ORIENTED_EDGE ( 'NONE', *, *, #18915, .T. ) ;
#4430=DIRECTION ( 'NONE',  ( 0.000000000000000000, 0.000000000000000000, -1.000000000000000000 ) ) ;
#4431=CARTESIAN_POINT ( 'NONE',  ( -1.387778780781445676E-14, 20.00000000000000000, -98.00000000000000000 ) ) ;
#4432=CIRCLE ( 'NONE', #12824, 2.099999999999997868 ) ;
#4435=EDGE_CURVE ( 'NONE', #17014, #18120, #22621, .T. ) ;
#4436=CARTESIAN_POINT ( 'NONE',  ( -3.630529889112771524, 39.68566040249004345, 51.94953878410922954 ) ) ;
#4439=VERTEX_POINT ( 'NONE', #16749 ) ;
#4442=CARTESIAN_POINT ( 'NONE',  ( -20.25803107563953631, 29.70716601075176300, 58.16264420749882191 ) ) ;
#4447=DIRECTION ( 'NONE',  ( 0.000000000000000000, 0.000000000000000000, -1.000000000000000000 ) ) ;
#4450=CARTESIAN_POINT ( 'NONE',  ( -8.970854721945018539, 37.88903791882350447, -54.67446985351440958 ) ) ;
#4452=CIRCLE ( 'NONE', #797, 2.499999999999995115 ) ;
#4455=CARTESIAN_POINT ( 'NONE',  ( 42.50000000000000711, -5.000000000000000000, -49.60000000000000142 ) ) ;
#4456=CARTESIAN_POINT ( 'NONE',  ( 34.99999999999980815, 28.00000000000000000, 54.99999999999922551 ) ) ;
#4457=CARTESIAN_POINT ( 'NONE',  ( 14.31754202316508540, 5.927758996453707852, 58.94936959136226307 ) ) ;
#4461=VERTEX_POINT ( 'NONE', #20422 ) ;
#4462=CARTESIAN_POINT ( 'NONE',  ( -35.00000000000000000, -4.928932188134504955, 1.387778780781445676E-14 ) ) ;
#4464=EDGE_CURVE ( 'NONE', #12113, #20626, #15765, .T. ) ;
#4466=ORIENTED_EDGE ( 'NONE', *, *, #2324, .T. ) ;
#4467=LINE ( 'NONE', #4124, #7832 ) ;
#4469=EDGE_CURVE ( 'NONE', #5777, #16804, #2624, .T. ) ;
#4471=ORIENTED_EDGE ( 'NONE', *, *, #5213, .T. ) ;
#4479=DIRECTION ( 'NONE',  ( 0.000000000000000000, 0.000000000000000000, -1.000000000000000000 ) ) ;
#4480=DIRECTION ( 'NONE',  ( 8.659560562353731078E-17, 0.7071067811866457165, -0.7071067811864494290 ) ) ;
#4481=CARTESIAN_POINT ( 'NONE',  ( 42.50000000000000711, -12.00000000000000000, -41.00000000000000000 ) ) ;
#4482=CARTESIAN_POINT ( 'NONE',  ( -0.01280385524457875075, 39.99999915041527743, -48.74393752659626955 ) ) ;
#4488=DIRECTION ( 'NONE',  ( 0.000000000000000000, 0.000000000000000000, -1.000000000000000000 ) ) ;
#4490=EDGE_LOOP ( 'NONE', ( #4871, #17342 ) ) ;
#4493=CARTESIAN_POINT ( 'NONE',  ( 15.58352763714662892, 32.54529335663308132, 59.37339313163358412 ) ) ;
#4496=CONICAL_SURFACE ( 'NONE', #9232, 2.525000000000110489, 0.7853981633971014453 ) ;
#4497=CARTESIAN_POINT ( 'NONE',  ( -1.387778780781445518E-14, 20.00000000000000355, 103.0000000000000284 ) ) ;
#4498=DIRECTION ( 'NONE',  ( 0.000000000000000000, 0.000000000000000000, 1.000000000000000000 ) ) ;
#4499=DIRECTION ( 'NONE',  ( 0.000000000000000000, -1.000000000000000000, 0.000000000000000000 ) ) ;
#4500=EDGE_LOOP ( 'NONE', ( #1973, #10839, #16806, #19862 ) ) ;
#4505=AXIS2_PLACEMENT_3D ( 'NONE', #1667, #10584, #21030 ) ;
#4507=CARTESIAN_POINT ( 'NONE',  ( -18.49252681899431039, 7.260825773989761700, -57.68517796515786245 ) ) ;
#4511=DIRECTION ( 'NONE',  ( 1.000000000000000000, 0.000000000000000000, 0.000000000000000000 ) ) ;
#4514=DIRECTION ( 'NONE',  ( -0.000000000000000000, 1.000000000000000000, -0.000000000000000000 ) ) ;
#4518=ADVANCED_FACE ( 'NONE', ( #18696 ), #22170, .T. ) ;
#4519=CARTESIAN_POINT ( 'NONE',  ( 10.88890858922251326, 36.78121034548748014, 57.56873443369040189 ) ) ;
#4520=CYLINDRICAL_SURFACE ( 'NONE', #9268, 2.500000000000002220 ) ;
#4522=CARTESIAN_POINT ( 'NONE',  ( 18.69481036107318417, 7.531781294123580217, -57.74428367179856281 ) ) ;
#4523=AXIS2_PLACEMENT_3D ( 'NONE', #270, #14233, #17920 ) ;
#4525=ORIENTED_EDGE ( 'NONE', *, *, #18092, .T. ) ;
#4532=AXIS2_PLACEMENT_3D ( 'NONE', #2953, #9927, #1456 ) ;
#4533=ORIENTED_EDGE ( 'NONE', *, *, #20797, .T. ) ;
#4534=DIRECTION ( 'NONE',  ( -0.000000000000000000, 1.000000000000000000, -0.000000000000000000 ) ) ;
#4536=ORIENTED_EDGE ( 'NONE', *, *, #22202, .F. ) ;
#4542=CIRCLE ( 'NONE', #9283, 14.00000000000000000 ) ;
#4545=CARTESIAN_POINT ( 'NONE',  ( -14.32898074910540842, 33.98521869245691107, -58.94425321795623063 ) ) ;
#4546=AXIS2_PLACEMENT_3D ( 'NONE', #3898, #12362, #5385 ) ;
#4552=ORIENTED_EDGE ( 'NONE', *, *, #13457, .F. ) ;
#4555=CARTESIAN_POINT ( 'NONE',  ( -17.83526554138388676, 10.93913794110440207, 60.06225905488084749 ) ) ;
#4560=FACE_OUTER_BOUND ( 'NONE', #18214, .T. ) ;
#4564=CYLINDRICAL_SURFACE ( 'NONE', #9751, 2.499999999999995115 ) ;
#4566=CARTESIAN_POINT ( 'NONE',  ( 4.084299015952138845, -4.682619376883142337, 48.27507093818913120 ) ) ;
#4567=CARTESIAN_POINT ( 'NONE',  ( -35.00000000000000000, 38.99999999999999289, 1.387778780781445676E-14 ) ) ;
#4568=ORIENTED_EDGE ( 'NONE', *, *, #20919, .T. ) ;
#4569=FACE_OUTER_BOUND ( 'NONE', #8724, .T. ) ;
#4572=CARTESIAN_POINT ( 'NONE',  ( 13.06496334681581395, 4.761428254737779753, 58.49034434780526936 ) ) ;
#4573=CARTESIAN_POINT ( 'NONE',  ( -26.00000000000001421, 19.99999999999982947, -100.0000000000000000 ) ) ;
#4574=VECTOR ( 'NONE', #1750, 1000.000000000000000 ) ;
#4575=EDGE_LOOP ( 'NONE', ( #2774, #6353 ) ) ;
#4576=FACE_OUTER_BOUND ( 'NONE', #16265, .T. ) ;
#4581=AXIS2_PLACEMENT_3D ( 'NONE', #17378, #5147, #8679 ) ;
#4583=CARTESIAN_POINT ( 'NONE',  ( 2.580936905856439978, 40.00000000000000711, -50.31086268949886176 ) ) ;
#4589=CARTESIAN_POINT ( 'NONE',  ( 10.78076590486229058, 39.17366535989027199, -54.93576791445503460 ) ) ;
#4591=LINE ( 'NONE', #8136, #15907 ) ;
#4596=CARTESIAN_POINT ( 'NONE',  ( 7.577104390335129835, -0.4826542685317783410, 53.01683071947729076 ) ) ;
#4597=CARTESIAN_POINT ( 'NONE',  ( 12.10743492718046532, 1.299801688895073637, -55.43551573823121004 ) ) ;
#4601=ADVANCED_FACE ( 'NONE', ( #20754 ), #22040, .F. ) ;
#4605=VERTEX_POINT ( 'NONE', #12896 ) ;
#4611=CARTESIAN_POINT ( 'NONE',  ( 18.31820558117432896, 28.04217374067966162, 60.19578215372065699 ) ) ;
#4612=AXIS2_PLACEMENT_3D ( 'NONE', #22677, #12218, #17146 ) ;
#4613=DIRECTION ( 'NONE',  ( -0.000000000000000000, 1.000000000000000000, -0.000000000000000000 ) ) ;
#4615=CARTESIAN_POINT ( 'NONE',  ( 11.68090480754630178, 3.765577839755386069, 57.90797000640142045 ) ) ;
#4616=CARTESIAN_POINT ( 'NONE',  ( -35.00000000000000000, 2.142135623730931471, -59.99999999999998579 ) ) ;
#4620=ORIENTED_EDGE ( 'NONE', *, *, #20136, .F. ) ;
#4621=CARTESIAN_POINT ( 'NONE',  ( -14.98515767422211198, 19.22844023086510745, -45.81928800960655224 ) ) ;
#4625=CARTESIAN_POINT ( 'NONE',  ( 12.30135915900896215, 4.212003844039729827, -58.16904039079300759 ) ) ;
#4627=DIRECTION ( 'NONE',  ( -1.000000000000000000, 0.000000000000000000, 0.000000000000000000 ) ) ;
#4631=AXIS2_PLACEMENT_3D ( 'NONE', #5212, #15732, #8761 ) ;
#4632=CARTESIAN_POINT ( 'NONE',  ( -7.545322633886957675, -0.4933377206467728926, -52.99899216500660515 ) ) ;
#4634=ORIENTED_EDGE ( 'NONE', *, *, #16184, .T. ) ;
#4635=CARTESIAN_POINT ( 'NONE',  ( 19.99999999999998579, 20.00000000000000355, 60.00200000000000244 ) ) ;
#4637=CARTESIAN_POINT ( 'NONE',  ( -1.387778780781445518E-14, 20.00000000000000355, 105.0000000000000142 ) ) ;
#4639=CARTESIAN_POINT ( 'NONE',  ( 18.34034842040247426, 28.02508533842880212, -60.20240101109772723 ) ) ;
#4642=ORIENTED_EDGE ( 'NONE', *, *, #22627, .T. ) ;
#4643=VERTEX_POINT ( 'NONE', #16229 ) ;
#4645=ORIENTED_EDGE ( 'NONE', *, *, #10715, .T. ) ;
#4648=EDGE_CURVE ( 'NONE', #12070, #5859, #13205, .T. ) ;
#4649=ORIENTED_EDGE ( 'NONE', *, *, #21516, .T. ) ;
#4651=CARTESIAN_POINT ( 'NONE',  ( -7.682546357470768861, -2.941798577935520687, -52.37062424970645225 ) ) ;
#4652=ORIENTED_EDGE ( 'NONE', *, *, #3921, .F. ) ;
#4655=DIRECTION ( 'NONE',  ( 0.000000000000000000, 0.000000000000000000, -1.000000000000000000 ) ) ;
#4656=ORIENTED_EDGE ( 'NONE', *, *, #1484, .F. ) ;
#4658=DIRECTION ( 'NONE',  ( -0.000000000000000000, -1.000000000000000000, -0.000000000000000000 ) ) ;
#4659=CARTESIAN_POINT ( 'NONE',  ( 1.325309500316239511E-14, -1.568768580316543204, -48.07879409069925458 ) ) ;
#4660=DIRECTION ( 'NONE',  ( -1.000000000000000000, 0.000000000000000000, 0.000000000000000000 ) ) ;
#4661=AXIS2_PLACEMENT_3D ( 'NONE', #20065, #7917, #7686 ) ;
#4663=EDGE_CURVE ( 'NONE', #10478, #10048, #2179, .T. ) ;
#4664=ORIENTED_EDGE ( 'NONE', *, *, #7731, .F. ) ;
#4666=ORIENTED_EDGE ( 'NONE', *, *, #15942, .T. ) ;
#4667=CARTESIAN_POINT ( 'NONE',  ( -15.23870778338556775, 7.010517948056213200, 56.68442755504044328 ) ) ;
#4668=EDGE_CURVE ( 'NONE', #18864, #7376, #11750, .T. ) ;
#4673=DIRECTION ( 'NONE',  ( -0.000000000000000000, -1.000000000000000000, -0.000000000000000000 ) ) ;
#4685=CARTESIAN_POINT ( 'NONE',  ( -42.50000000000000711, -12.00000000000000000, -47.50000000000000000 ) ) ;
#4686=ORIENTED_EDGE ( 'NONE', *, *, #11357, .T. ) ;
#4688=CARTESIAN_POINT ( 'NONE',  ( 6.696867368503558448E-15, 40.00000000000000000, 48.73397172404481381 ) ) ;
#4690=AXIS2_PLACEMENT_3D ( 'NONE', #4791, #17367, #15527 ) ;
#4693=EDGE_CURVE ( 'NONE', #19784, #14544, #14297, .T. ) ;
#4694=AXIS2_PLACEMENT_3D ( 'NONE', #12344, #19355, #3661 ) ;
#4706=DIRECTION ( 'NONE',  ( 0.000000000000000000, 0.000000000000000000, 1.000000000000000000 ) ) ;
#4707=DIRECTION ( 'NONE',  ( -0.000000000000000000, -0.000000000000000000, -1.000000000000000000 ) ) ;
#4708=AXIS2_PLACEMENT_3D ( 'NONE', #3296, #8547, #13459 ) ;
#4709=CARTESIAN_POINT ( 'NONE',  ( -13.76792553423404541, 26.00189441538237745, -45.26963775109936705 ) ) ;
#4710=CARTESIAN_POINT ( 'NONE',  ( -10.49999999999980460, -2.516660498395515866, 60.00099999999999767 ) ) ;
#4712=ORIENTED_EDGE ( 'NONE', *, *, #21402, .T. ) ;
#4714=CARTESIAN_POINT ( 'NONE',  ( -4.295527433237782828E-15, -1.236374842841486021, 48.24164917503448180 ) ) ;
#4721=ADVANCED_FACE ( 'NONE', ( #15064 ), #13564, .F. ) ;
#4722=ADVANCED_FACE ( 'NONE', ( #13342 ), #18649, .F. ) ;
#4723=EDGE_CURVE ( 'NONE', #1751, #15249, #20264, .T. ) ;
#4725=AXIS2_PLACEMENT_3D ( 'NONE', #18838, #6582, #19064 ) ;
#4728=EDGE_CURVE ( 'NONE', #6038, #7926, #6526, .T. ) ;
#4732=CARTESIAN_POINT ( 'NONE',  ( 18.87121696173697316, 26.69448804128720809, -60.34297443853446197 ) ) ;
#4733=CARTESIAN_POINT ( 'NONE',  ( -13.33780792070361443, 2.142135623730931471, 45.06383732350886362 ) ) ;
#4734=LINE ( 'NONE', #20423, #6260 ) ;
#4737=DIRECTION ( 'NONE',  ( -0.000000000000000000, 1.000000000000000000, -0.000000000000000000 ) ) ;
#4744=FACE_OUTER_BOUND ( 'NONE', #10514, .T. ) ;
#4745=CARTESIAN_POINT ( 'NONE',  ( 9.728382623732244383, 39.99999999999997868, 53.57939893017088195 ) ) ;
#4747=CARTESIAN_POINT ( 'NONE',  ( -7.766911017765431247, 39.99999999999999289, -52.87044927329080934 ) ) ;
#4752=DIRECTION ( 'NONE',  ( -0.000000000000000000, -1.000000000000000000, -0.000000000000000000 ) ) ;
#4753=CARTESIAN_POINT ( 'NONE',  ( 34.99999999999980815, 40.00000000000000000, 57.09999999999921982 ) ) ;
#4755=CARTESIAN_POINT ( 'NONE',  ( 19.45266119884270495, 15.02268094490047368, -60.49039575453066675 ) ) ;
#4759=VERTEX_POINT ( 'NONE', #18278 ) ;
#4763=CARTESIAN_POINT ( 'NONE',  ( 14.99999999999998579, 20.00000000000000000, 45.82575694955838230 ) ) ;
#4764=EDGE_CURVE ( 'NONE', #2374, #21198, #6137, .T. ) ;
#4766=DIRECTION ( 'NONE',  ( 0.000000000000000000, 0.000000000000000000, 1.000000000000000000 ) ) ;
#4771=ORIENTED_EDGE ( 'NONE', *, *, #3851, .F. ) ;
#4772=CARTESIAN_POINT ( 'NONE',  ( 90.00000000000000000, 26.00000000000000355, -9.108981535246192915E-16 ) ) ;
#4773=CARTESIAN_POINT ( 'NONE',  ( 42.50000000000000711, -5.000000000000000000, 47.50000000000000711 ) ) ;
#4775=CARTESIAN_POINT ( 'NONE',  ( -19.64447802513834063, 23.87744830687368491, -60.53680291695862081 ) ) ;
#4778=CARTESIAN_POINT ( 'NONE',  ( -12.70473862104220153, 11.99136930790643163, 44.75655646380171504 ) ) ;
#4780=ORIENTED_EDGE ( 'NONE', *, *, #12686, .T. ) ;
#4782=EDGE_LOOP ( 'NONE', ( #10278, #9271, #17612, #1740 ) ) ;
#4783=CARTESIAN_POINT ( 'NONE',  ( -18.43720426449199223, 27.80056269872155283, 57.71457384195534956 ) ) ;
#4784=DIRECTION ( 'NONE',  ( -0.000000000000000000, -0.000000000000000000, -1.000000000000000000 ) ) ;
#4785=CARTESIAN_POINT ( 'NONE',  ( -14.06256854266897705, 5.693415384482571895, -58.85512087818929672 ) ) ;
#4788=ORIENTED_EDGE ( 'NONE', *, *, #423, .T. ) ;
#4790=CARTESIAN_POINT ( 'NONE',  ( -4.465627739065156199, 40.00000000000001421, -51.33835364202109020 ) ) ;
#4791=CARTESIAN_POINT ( 'NONE',  ( -1.387778780781445518E-14, 20.00000000000000355, -102.9999999999999716 ) ) ;
#4792=FACE_OUTER_BOUND ( 'NONE', #14709, .T. ) ;
#4801=VERTEX_POINT ( 'NONE', #634 ) ;
#4803=ORIENTED_EDGE ( 'NONE', *, *, #22363, .T. ) ;
#4804=CARTESIAN_POINT ( 'NONE',  ( -5.761861175224586518, -0.6790081076912936053, 52.02240682770946023 ) ) ;
#4805=ADVANCED_FACE ( 'NONE', ( #19667 ), #7440, .T. ) ;
#4808=EDGE_LOOP ( 'NONE', ( #10933, #17855 ) ) ;
#4810=AXIS2_PLACEMENT_3D ( 'NONE', #10260, #18752, #8106 ) ;
#4811=DIRECTION ( 'NONE',  ( -0.000000000000000000, 1.000000000000000000, -0.000000000000000000 ) ) ;
#4813=ADVANCED_FACE ( 'NONE', ( #2591 ), #11098, .F. ) ;
#4814=CARTESIAN_POINT ( 'NONE',  ( -20.00401474702687921, 19.84140115762917489, -58.14847693657501537 ) ) ;
#4815=DIRECTION ( 'NONE',  ( -0.000000000000000000, -0.000000000000000000, -1.000000000000000000 ) ) ;
#4816=CARTESIAN_POINT ( 'NONE',  ( -11.24990497772101605, 36.62343892044449234, 57.74518096503233267 ) ) ;
#4817=ORIENTED_EDGE ( 'NONE', *, *, #22265, .T. ) ;
#4818=CARTESIAN_POINT ( 'NONE',  ( -35.00000000000000000, -5.000000000000000000, 1.387778780781445676E-14 ) ) ;
#4819=FACE_BOUND ( 'NONE', #22108, .T. ) ;
#4820=CARTESIAN_POINT ( 'NONE',  ( -35.00000000000000000, -5.000000000000000888, -17.99999999999998934 ) ) ;
#4821=DIRECTION ( 'NONE',  ( 0.000000000000000000, 0.000000000000000000, 1.000000000000000000 ) ) ;
#4822=EDGE_LOOP ( 'NONE', ( #5242, #20888, #14382, #3515 ) ) ;
#4826=CARTESIAN_POINT ( 'NONE',  ( 35.00000000000058265, 28.00000000000000000, -52.50000000000076739 ) ) ;
#4827=VECTOR ( 'NONE', #17904, 1000.000000000000000 ) ;
#4830=EDGE_LOOP ( 'NONE', ( #1185, #5337, #82, #725 ) ) ;
#4836=DIRECTION ( 'NONE',  ( 1.000000000000000000, 0.000000000000000000, 0.000000000000000000 ) ) ;
#4839=DIRECTION ( 'NONE',  ( 0.000000000000000000, 0.000000000000000000, -1.000000000000000000 ) ) ;
#4840=ORIENTED_EDGE ( 'NONE', *, *, #9555, .F. ) ;
#4844=DIRECTION ( 'NONE',  ( 0.000000000000000000, 0.000000000000000000, 1.000000000000000000 ) ) ;
#4851=CARTESIAN_POINT ( 'NONE',  ( -35.00000000000058265, 26.00000000000000355, -55.00000000000076028 ) ) ;
#4852=CARTESIAN_POINT ( 'NONE',  ( -14.34650594848455896, 37.25275621493270251, 56.33443587181654522 ) ) ;
#4857=CARTESIAN_POINT ( 'NONE',  ( 16.64903669412982978, 31.11586081922178337, -59.71532480898645900 ) ) ;
#4862=ORIENTED_EDGE ( 'NONE', *, *, #15313, .F. ) ;
#4865=ORIENTED_EDGE ( 'NONE', *, *, #9290, .F. ) ;
#4868=ORIENTED_EDGE ( 'NONE', *, *, #17392, .T. ) ;
#4870=CARTESIAN_POINT ( 'NONE',  ( -9.327259721472405118, -2.742977016014211511, -53.40697688051520942 ) ) ;
#4871=ORIENTED_EDGE ( 'NONE', *, *, #22619, .F. ) ;
#4873=ORIENTED_EDGE ( 'NONE', *, *, #171, .F. ) ;
#4874=CARTESIAN_POINT ( 'NONE',  ( 7.073833244813752863, 38.72384638770318332, -54.13588498570150165 ) ) ;
#4877=CARTESIAN_POINT ( 'NONE',  ( -18.85684496195311866, 26.68267098057082976, -60.33873919100125960 ) ) ;
#4880=EDGE_CURVE ( 'NONE', #21115, #17014, #16910, .T. ) ;
#4882=CARTESIAN_POINT ( 'NONE',  ( 9.689843208404422370, 39.33333333333334281, -54.54983754392748097 ) ) ;
#4888=FACE_OUTER_BOUND ( 'NONE', #21108, .T. ) ;
#4890=AXIS2_PLACEMENT_3D ( 'NONE', #2626, #21874, #11324 ) ;
#4891=CIRCLE ( 'NONE', #21004, 16.99999999999998579 ) ;
#4892=CARTESIAN_POINT ( 'NONE',  ( 2.247165119384746834, 39.96957922271067787, -50.40104177638675509 ) ) ;
#4894=DIRECTION ( 'NONE',  ( -0.000000000000000000, -1.000000000000000000, -0.000000000000000000 ) ) ;
#4898=CARTESIAN_POINT ( 'NONE',  ( -2.026529067239271509, 40.00000000000000711, -49.98891171552928370 ) ) ;
#4900=CARTESIAN_POINT ( 'NONE',  ( 10.43027093729823562, 39.22757009021513142, -54.80615623442508877 ) ) ;
#4901=AXIS2_PLACEMENT_3D ( 'NONE', #765, #647, #7748 ) ;
#4908=CARTESIAN_POINT ( 'NONE',  ( 34.99999999999980105, 24.73819270004212356, 54.99999999999922551 ) ) ;
#4911=ADVANCED_FACE ( 'NONE', ( #18732 ), #16496, .F. ) ;
#4913=CARTESIAN_POINT ( 'NONE',  ( -3.021476695451119188, -1.097455775060080407, 50.32853965771198546 ) ) ;
#4916=ORIENTED_EDGE ( 'NONE', *, *, #4129, .T. ) ;
#4918=CARTESIAN_POINT ( 'NONE',  ( 9.852267639826642665, 8.683574217357131531, 43.21671877549180607 ) ) ;
#4919=AXIS2_PLACEMENT_3D ( 'NONE', #18298, #20477, #9820 ) ;
#4922=CARTESIAN_POINT ( 'NONE',  ( -22.29034605647555978, 17.39518641927480047, -58.63862881473036026 ) ) ;
#4924=CARTESIAN_POINT ( 'NONE',  ( -11.38359864655678777, 29.79463497853557996, -44.07478837098127400 ) ) ;
#4925=CARTESIAN_POINT ( 'NONE',  ( -9.829668860677969633, 37.49547983895929804, 57.11616152306119432 ) ) ;
#4926=ORIENTED_EDGE ( 'NONE', *, *, #4032, .F. ) ;
#4927=CARTESIAN_POINT ( 'NONE',  ( 6.426802710256914963, 33.56875711009141838, 41.03786381671501005 ) ) ;
#4928=CARTESIAN_POINT ( 'NONE',  ( 11.05758567243059609, 3.294696707144193493, -55.18338768060583277 ) ) ;
#4931=CIRCLE ( 'NONE', #19946, 1.999999999999999778 ) ;
#4933=DIRECTION ( 'NONE',  ( 8.659560562354892183E-17, 0.7071067811865507924, -0.7071067811865441310 ) ) ;
#4940=ORIENTED_EDGE ( 'NONE', *, *, #15419, .F. ) ;
#4946=DIRECTION ( 'NONE',  ( -0.000000000000000000, -1.000000000000000000, -0.000000000000000000 ) ) ;
#4947=EDGE_LOOP ( 'NONE', ( #21975, #2184, #13909, #4047, #7264 ) ) ;
#4948=DIRECTION ( 'NONE',  ( 0.000000000000000000, 0.5150380749100562650, 0.8571673007021111124 ) ) ;
#4951=CARTESIAN_POINT ( 'NONE',  ( 34.99999999999980815, 40.00000000000000000, 54.99999999999922551 ) ) ;
#4953=CIRCLE ( 'NONE', #17383, 2.000000000000001776 ) ;
#4955=EDGE_LOOP ( 'NONE', ( #12141, #20649, #6787, #14295 ) ) ;
#4956=CARTESIAN_POINT ( 'NONE',  ( 14.92530643917651823, 21.54450079162174347, -45.79309713780074986 ) ) ;
#4959=CARTESIAN_POINT ( 'NONE',  ( -20.89512770937652775, 28.22558907592242150, 58.31975796628790931 ) ) ;
#4966=CIRCLE ( 'NONE', #19955, 60.00000000000000000 ) ;
#4967=CARTESIAN_POINT ( 'NONE',  ( 13.03660953228075492, 4.807999378483715169, -58.46122805341365591 ) ) ;
#4969=EDGE_CURVE ( 'NONE', #21483, #14094, #22406, .T. ) ;
#4970=EDGE_LOOP ( 'NONE', ( #16703, #7390, #4111, #15223 ) ) ;
#4976=CARTESIAN_POINT ( 'NONE',  ( 17.21639554191072818, 34.43961005730907488, 57.30688911148507714 ) ) ;
#4977=CARTESIAN_POINT ( 'NONE',  ( 9.727694841165407169, 39.99999999999998579, -53.57919902740184881 ) ) ;
#4978=ADVANCED_FACE ( 'NONE', ( #15387 ), #12063, .T. ) ;
#4984=FACE_OUTER_BOUND ( 'NONE', #990, .T. ) ;
#4986=CONICAL_SURFACE ( 'NONE', #2409, 2.524999999999999467, 0.7853981633973095011 ) ;
#4989=DIRECTION ( 'NONE',  ( -0.000000000000000000, 1.000000000000000000, -0.000000000000000000 ) ) ;
#4990=EDGE_CURVE ( 'NONE', #15385, #548, #10897, .T. ) ;
#4992=CARTESIAN_POINT ( 'NONE',  ( 42.50000000000000711, -5.000000000000000000, 54.00000000000000711 ) ) ;
#4996=CARTESIAN_POINT ( 'NONE',  ( -15.00000000000001421, 19.61444766276327556, 45.82575694955841072 ) ) ;
#4998=VECTOR ( 'NONE', #14731, 1000.000000000000000 ) ;
#5007=DIRECTION ( 'NONE',  ( -0.000000000000000000, -1.000000000000000000, -0.000000000000000000 ) ) ;
#5009=DIRECTION ( 'NONE',  ( -1.000000000000000000, 0.000000000000000000, 0.000000000000000000 ) ) ;
#5011=DIRECTION ( 'NONE',  ( 0.000000000000000000, 0.000000000000000000, -1.000000000000000000 ) ) ;
#5013=ORIENTED_EDGE ( 'NONE', *, *, #2072, .F. ) ;
#5015=CARTESIAN_POINT ( 'NONE',  ( -4.719078656571195296, 39.99999999999999289, -51.46810812756150000 ) ) ;
#5023=VECTOR ( 'NONE', #20204, 1000.000000000000000 ) ;
#5030=CONICAL_SURFACE ( 'NONE', #18186, 2.524999999999999467, 0.7853981633973095011 ) ;
#5031=ADVANCED_FACE ( 'NONE', ( #259, #5210, #8860 ), #20793, .F. ) ;
#5032=ORIENTED_EDGE ( 'NONE', *, *, #777, .T. ) ;
#5033=CARTESIAN_POINT ( 'NONE',  ( -8.526039741978737041, -2.856534014484948258, 52.89583463521491780 ) ) ;
#5035=ORIENTED_EDGE ( 'NONE', *, *, #4401, .F. ) ;
#5036=CARTESIAN_POINT ( 'NONE',  ( 11.38359864655677711, 10.20536502146444313, 44.07478837098129532 ) ) ;
#5037=( BOUNDED_SURFACE ( )  B_SPLINE_SURFACE ( 3, 2, ( 
 ( #18850, #20568, #18736 ),
 ( #8196, #1545, #22525 ),
 ( #3157, #22648, #6821 ),
 ( #13784, #8645, #20800 ),
 ( #20916, #4874, #5112 ),
 ( #11741, #15620, #13442 ),
 ( #19079, #3386, #11630 ),
 ( #9911, #18633, #2938 ),
 ( #1315, #8308, #7379 ),
 ( #385, #10920, #10676 ),
 ( #21352, #15737, #12191 ),
 ( #21134, #14459, #7489 ),
 ( #3619, #17682, #3501 ),
 ( #19310, #5217, #9102 ) ),
 .UNSPECIFIED., .F., .F., .F. ) 
 B_SPLINE_SURFACE_WITH_KNOTS ( ( 4, 2, 2, 2, 2, 2, 4 ),
 ( 3, 3 ),
 ( 0.004259382447192485224, 0.005809352080732410606, 0.007359321714272335120, 0.008909291347812259634, 0.01045926098135218502, 0.01355920024843203578, 0.01665913951551188654 ),
 ( 0.1636502049369185086, 1.000000000000000000 ),
 .UNSPECIFIED. ) 
 GEOMETRIC_REPRESENTATION_ITEM ( )  RATIONAL_B_SPLINE_SURFACE ( (
 ( 0.9022234441951376693, 0.7012635705450175339, 1.000000000000000000),
 ( 0.9123774980386742950, 0.7322872220199752036, 1.000000000000000000),
 ( 0.9211831106396635160, 0.7591909848486969592, 1.000000000000000000),
 ( 0.9369226144573956638, 0.8072798455494799574, 1.000000000000000000),
 ( 0.9438532932728125324, 0.8284551285810179966, 1.000000000000000000),
 ( 0.9562652441348715726, 0.8663773263162527494, 1.000000000000000000),
 ( 0.9617542084831443017, 0.8831477432869754285, 1.000000000000000000),
 ( 0.9714480778053882215, 0.9127653943188843710, 1.000000000000000000),
 ( 0.9756417576472291575, 0.9255783322661890189, 1.000000000000000000),
 ( 0.9865757101953547270, 0.9589848060079729786, 1.000000000000000000),
 ( 0.9916868072432731829, 0.9746007261037917813, 1.000000000000000000),
 ( 0.9984050148984049411, 0.9951268466110081423, 1.000000000000000000),
 ( 0.9999940431410754282, 0.9999818000260773943, 1.000000000000000000),
 ( 1.000000000000000000, 1.000000000000000000, 1.000000000000000000) ) ) 
 REPRESENTATION_ITEM ( '' )  SURFACE ( )  );
#5039=EDGE_CURVE ( 'NONE', #3941, #8689, #18560, .T. ) ;
#5040=AXIS2_PLACEMENT_3D ( 'NONE', #16164, #4613, #16633 ) ;
#5041=CARTESIAN_POINT ( 'NONE',  ( -0.5279010140432128795, 35.00028092684671321, -38.73355033370099676 ) ) ;
#5043=CARTESIAN_POINT ( 'NONE',  ( -16.71858216490109328, 8.984148545335303382, -57.18548413420069210 ) ) ;
#5044=FACE_OUTER_BOUND ( 'NONE', #12991, .T. ) ;
#5050=FACE_BOUND ( 'NONE', #7550, .T. ) ;
#5055=CARTESIAN_POINT ( 'NONE',  ( -35.00000000000058265, 40.00000000000000711, -55.00000000000076028 ) ) ;
#5057=EDGE_CURVE ( 'NONE', #4131, #3734, #6491, .T. ) ;
#5061=AXIS2_PLACEMENT_3D ( 'NONE', #20760, #15802, #17196 ) ;
#5065=ORIENTED_EDGE ( 'NONE', *, *, #20954, .F. ) ;
#5066=CARTESIAN_POINT ( 'NONE',  ( 13.00000000000024336, -2.516660498395250745, 60.00099999999999767 ) ) ;
#5068=DIRECTION ( 'NONE',  ( 0.000000000000000000, -1.000000000000000000, 0.000000000000000000 ) ) ;
#5069=LINE ( 'NONE', #19267, #15993 ) ;
#5072=DIRECTION ( 'NONE',  ( -1.000000000000000000, 0.000000000000000000, 0.000000000000000000 ) ) ;
#5073=CARTESIAN_POINT ( 'NONE',  ( -11.89435616776549232, 40.00000000000000000, -54.28884887643229007 ) ) ;
#5078=CARTESIAN_POINT ( 'NONE',  ( 3.801357092295314821, 39.91216781786773282, 51.45795407606280492 ) ) ;
#5079=CARTESIAN_POINT ( 'NONE',  ( 14.87996495114178153, 21.93329436794036269, -45.77322900830822761 ) ) ;
#5080=AXIS2_PLACEMENT_3D ( 'NONE', #5853, #576, #21431 ) ;
#5083=CARTESIAN_POINT ( 'NONE',  ( -21.07599011712229853, 12.09199673218657622, 58.36745205258139890 ) ) ;
#5084=EDGE_CURVE ( 'NONE', #20516, #11968, #22519, .T. ) ;
#5087=LINE ( 'NONE', #17096, #12345 ) ;
#5091=ADVANCED_FACE ( 'NONE', ( #3381 ), #16741, .F. ) ;
#5092=B_SPLINE_SURFACE_WITH_KNOTS ( 'NONE', 1, 3, ( 
 ( #12049, #3351, #114, #7107, #12376, #19386 ),
 ( #17305, #1395, #11928, #1622, #8603, #453 ) ),
 .UNSPECIFIED., .F., .F., .F.,
 ( 2, 2 ),
 ( 4, 2, 4 ),
 ( 0.000000000000000000, 1.000000000000000000 ),
 ( 0.000000000000000000, 0.001214050925806517758, 0.002428101851613035517 ),
 .UNSPECIFIED. ) ;
#5095=ORIENTED_EDGE ( 'NONE', *, *, #1897, .T. ) ;
#5097=B_SPLINE_CURVE_WITH_KNOTS ( 'NONE', 3,
 ( #4615, #15011, #18810, #22027, #11595, #17077, #18589, #16865, #15354, #22373, #6660, #2898, #9874, #8156, #13618, #18923 ),
 .UNSPECIFIED., .F., .F.,
 ( 4, 2, 2, 2, 2, 2, 2, 4 ),
 ( 0.000000000000000000, 0.004782611835060866790, 0.005978264793826080885, 0.007173917752591294113, 0.009565223670121721436, 0.01195652958765214442, 0.01434783550518256914, 0.01913044734024342899 ),
 .UNSPECIFIED. ) ;
#5098=ORIENTED_EDGE ( 'NONE', *, *, #775, .T. ) ;
#5099=FACE_OUTER_BOUND ( 'NONE', #1982, .T. ) ;
#5102=CARTESIAN_POINT ( 'NONE',  ( 20.16756852208514772, 29.88972976525005976, 58.13897502025236719 ) ) ;
#5103=CARTESIAN_POINT ( 'NONE',  ( -13.00000000000011546, 42.51666049839536043, -105.0010000000000048 ) ) ;
#5107=CARTESIAN_POINT ( 'NONE',  ( -18.00000000000001421, 20.00000000000000711, 102.0000000000000142 ) ) ;
#5112=CARTESIAN_POINT ( 'NONE',  ( 6.433485051968857782, 38.94088993357618733, -55.16018527339313238 ) ) ;
#5117=AXIS2_PLACEMENT_3D ( 'NONE', #4456, #6051, #11432 ) ;
#5122=VERTEX_POINT ( 'NONE', #14572 ) ;
#5125=CARTESIAN_POINT ( 'NONE',  ( 13.00000000000024336, -2.516660498395250745, -105.0000000000000142 ) ) ;
#5127=AXIS2_PLACEMENT_3D ( 'NONE', #7091, #19132, #14171 ) ;
#5130=CARTESIAN_POINT ( 'NONE',  ( 6.675595648756416089, 39.71118687073258258, 53.17234506582082787 ) ) ;
#5133=CARTESIAN_POINT ( 'NONE',  ( -2.274190298599449100, 40.00000000000000000, -50.13372678551965578 ) ) ;
#5134=ADVANCED_FACE ( 'NONE', ( #2097 ), #18133, .T. ) ;
#5143=CARTESIAN_POINT ( 'NONE',  ( -15.58771758597476875, 32.56665981830160916, 59.37826087086043714 ) ) ;
#5144=ORIENTED_EDGE ( 'NONE', *, *, #15319, .T. ) ;
#5145=DIRECTION ( 'NONE',  ( 0.000000000000000000, 0.000000000000000000, -1.000000000000000000 ) ) ;
#5146=VECTOR ( 'NONE', #15309, 1000.000000000000000 ) ;
#5147=DIRECTION ( 'NONE',  ( -0.000000000000000000, -0.000000000000000000, -1.000000000000000000 ) ) ;
#5148=DIRECTION ( 'NONE',  ( 0.000000000000000000, 0.000000000000000000, -1.000000000000000000 ) ) ;
#5150=ORIENTED_EDGE ( 'NONE', *, *, #11126, .T. ) ;
#5155=ORIENTED_EDGE ( 'NONE', *, *, #20962, .F. ) ;
#5157=CARTESIAN_POINT ( 'NONE',  ( -5.422195817667174289, 33.99281763503099540, -40.31637036980814770 ) ) ;
#5159=CARTESIAN_POINT ( 'NONE',  ( -19.02718446893024762, 26.17927818496970716, -57.88297158504751394 ) ) ;
#5163=CARTESIAN_POINT ( 'NONE',  ( -1.387778780781445518E-14, 20.00000000000000355, -105.0000000000000142 ) ) ;
#5164=LINE ( 'NONE', #19135, #5610 ) ;
#5168=CARTESIAN_POINT ( 'NONE',  ( 25.99999999999998579, 19.99999999999999645, -105.0000000000000142 ) ) ;
#5171=ORIENTED_EDGE ( 'NONE', *, *, #17634, .T. ) ;
#5173=ORIENTED_EDGE ( 'NONE', *, *, #4764, .F. ) ;
#5177=CARTESIAN_POINT ( 'NONE',  ( -35.00000000000058975, 24.73819270004212356, -55.00000000000076028 ) ) ;
#5179=ORIENTED_EDGE ( 'NONE', *, *, #10704, .F. ) ;
#5183=CARTESIAN_POINT ( 'NONE',  ( 10.27431133777637484, -4.928932188134504955, -51.43682631505696179 ) ) ;
#5184=CARTESIAN_POINT ( 'NONE',  ( 20.34735785252014395, 29.47800210776922469, -58.18363580933384327 ) ) ;
#5185=DIRECTION ( 'NONE',  ( 0.000000000000000000, 0.5150380749100562650, 0.8571673007021111124 ) ) ;
#5186=CARTESIAN_POINT ( 'NONE',  ( 8.118562860349435084, 39.55762401320047417, 53.90122740908830679 ) ) ;
#5188=ORIENTED_EDGE ( 'NONE', *, *, #4077, .F. ) ;
#5189=CARTESIAN_POINT ( 'NONE',  ( -42.50000000000000711, -12.00000000000000000, 47.50000000000000711 ) ) ;
#5190=DIRECTION ( 'NONE',  ( 0.000000000000000000, 1.000000000000000000, 0.000000000000000000 ) ) ;
#5196=DIRECTION ( 'NONE',  ( -0.000000000000000000, 1.000000000000000000, -0.000000000000000000 ) ) ;
#5197=PLANE ( 'NONE',  #7478 ) ;
#5198=ORIENTED_EDGE ( 'NONE', *, *, #10974, .T. ) ;
#5199=ORIENTED_EDGE ( 'NONE', *, *, #15001, .F. ) ;
#5203=ORIENTED_EDGE ( 'NONE', *, *, #16776, .F. ) ;
#5204=CARTESIAN_POINT ( 'NONE',  ( 17.96165932904279572, 6.521477064918314248, 57.53061250216241973 ) ) ;
#5206=CARTESIAN_POINT ( 'NONE',  ( 6.910515180469714913, 40.00000000000002132, -52.51112560306592059 ) ) ;
#5207=CARTESIAN_POINT ( 'NONE',  ( 3.397749794379752331, 40.00000000000000000, 50.77335383852931727 ) ) ;
#5208=ORIENTED_EDGE ( 'NONE', *, *, #11829, .T. ) ;
#5209=LINE ( 'NONE', #1539, #5790 ) ;
#5210=FACE_BOUND ( 'NONE', #2225, .T. ) ;
#5212=CARTESIAN_POINT ( 'NONE',  ( 35.00000000000058265, 40.00000000000000000, -55.00000000000076028 ) ) ;
#5213=EDGE_CURVE ( 'NONE', #16803, #13092, #2479, .T. ) ;
#5215=CARTESIAN_POINT ( 'NONE',  ( 7.776554266669417956E-15, -4.648749848372173865, -45.43309249825056639 ) ) ;
#5216=ORIENTED_EDGE ( 'NONE', *, *, #10356, .T. ) ;
#5217=CARTESIAN_POINT ( 'NONE',  ( -2.782727930551067045E-14, 40.00000000000000000, -48.73397172404478539 ) ) ;
#5218=CARTESIAN_POINT ( 'NONE',  ( -35.00000000000000000, 40.00000000000000000, 1.387778780781445676E-14 ) ) ;
#5219=CARTESIAN_POINT ( 'NONE',  ( -0.7618512339543030976, 39.99660974252569901, 49.31784456962214591 ) ) ;
#5226=ORIENTED_EDGE ( 'NONE', *, *, #7212, .F. ) ;
#5228=EDGE_LOOP ( 'NONE', ( #12581, #8173, #21367, #17267 ) ) ;
#5229=DIRECTION ( 'NONE',  ( 0.000000000000000000, 0.000000000000000000, -1.000000000000000000 ) ) ;
#5230=DIRECTION ( 'NONE',  ( -1.000000000000000000, 0.000000000000000000, 0.000000000000000000 ) ) ;
#5232=CARTESIAN_POINT ( 'NONE',  ( 0.09252246807544707574, 39.99995033533620870, 48.80586619582643237 ) ) ;
#5235=ORIENTED_EDGE ( 'NONE', *, *, #17003, .F. ) ;
#5237=DIRECTION ( 'NONE',  ( 0.000000000000000000, 0.000000000000000000, 1.000000000000000000 ) ) ;
#5242=ORIENTED_EDGE ( 'NONE', *, *, #15883, .F. ) ;
#5247=FACE_BOUND ( 'NONE', #17588, .T. ) ;
#5248=B_SPLINE_CURVE_WITH_KNOTS ( 'NONE', 3,
 ( #10425, #12159, #9065, #19606, #5507, #12479, #234, #17647, #351, #14309, #3915, #10643, #8607, #17424, #7009, #10540, #19491, #7228, #3798, #15585, #17765, #6904, #16041, #5616, #13866, #13965, #20882, #5184, #1743, #8726, #8833, #15703, #18, #20989, #5294, #17544, #118, #11223, #16386, #7683 ),
 .UNSPECIFIED., .F., .F.,
 ( 4, 2, 2, 2, 2, 2, 2, 2, 2, 2, 2, 2, 2, 2, 2, 2, 2, 2, 2, 4 ),
 ( 0.000000000000000000, 0.002766773850155581499, 0.004150160775233378320, 0.005533547700311174274, 0.008300321550466765314, 0.009683708475544557798, 0.01106709540062235028, 0.01660064310093351328, 0.01798403002601130229, 0.01936741695108909131, 0.02213419080124466587, 0.02490096465140024390, 0.02766773850155581846, 0.03043451235171139649, 0.03181789927678917856, 0.03320128620186695717, 0.03873483390217812017, 0.04011822082725590571, 0.04150160775233369126, 0.04426838160248925541 ),
 .UNSPECIFIED. ) ;
#5250=ORIENTED_EDGE ( 'NONE', *, *, #431, .F. ) ;
#5256=CARTESIAN_POINT ( 'NONE',  ( 2.419767991124955664, -3.149022461041079968, -49.02154318835233227 ) ) ;
#5257=DIRECTION ( 'NONE',  ( 0.000000000000000000, 0.000000000000000000, 1.000000000000000000 ) ) ;
#5258=ORIENTED_EDGE ( 'NONE', *, *, #20161, .T. ) ;
#5259=CARTESIAN_POINT ( 'NONE',  ( -28.50000000000001421, 19.99999999999982947, 105.0000000000000142 ) ) ;
#5262=CARTESIAN_POINT ( 'NONE',  ( -17.35828117057637954, 30.07901706856257817, -57.39628071425624256 ) ) ;
#5263=DIRECTION ( 'NONE',  ( 0.000000000000000000, 0.000000000000000000, -1.000000000000000000 ) ) ;
#5264=B_SPLINE_SURFACE_WITH_KNOTS ( 'NONE', 1, 3, ( 
 ( #21434, #9620, #4038, #579, #11453, #18102, #12823, #19836, #11114, #806, #12932, #2418, #9407, #19942, #14766, #6077, #4369, #11346, #16613, #7913 ),
 ( #14873, #21899, #6195, #13159, #22234, #1250, #13598, #11898, #13491, #20736, #6300, #18903, #2757, #17058, #8468, #9953, #15437, #8243, #3090, #6754 ) ),
 .UNSPECIFIED., .F., .F., .F.,
 ( 2, 2 ),
 ( 4, 2, 2, 2, 2, 2, 2, 2, 2, 4 ),
 ( 0.000000000000000000, 1.000000000000000000 ),
 ( -4.246609446761914828E-05, 0.0006546318687081847335, 0.001351729831883988642, 0.002048827795059792768, 0.002745925758235596460, 0.004140121684587204712, 0.005534317610938812096, 0.006928513537290420347, 0.008322709463642028599, 0.01111110131634524337 ),
 .UNSPECIFIED. ) ;
#5265=AXIS2_PLACEMENT_3D ( 'NONE', #2512, #11200, #16704 ) ;
#5269=CIRCLE ( 'NONE', #22105, 49.99999999999998579 ) ;
#5274=ORIENTED_EDGE ( 'NONE', *, *, #364, .F. ) ;
#5276=PLANE ( 'NONE',  #1316 ) ;
#5277=CARTESIAN_POINT ( 'NONE',  ( -35.00000000000058265, 28.00000000000000000, -55.00000000000076028 ) ) ;
#5280=AXIS2_PLACEMENT_3D ( 'NONE', #17506, #8803, #17384 ) ;
#5282=ADVANCED_FACE ( 'NONE', ( #9649 ), #15259, .T. ) ;
#5285=CARTESIAN_POINT ( 'NONE',  ( -1.039655021832126547, -3.147609295952968456, 46.52691668518833268 ) ) ;
#5287=CARTESIAN_POINT ( 'NONE',  ( -10.99584631063772378, 3.272668205460793178, 57.61971594758626480 ) ) ;
#5289=VERTEX_POINT ( 'NONE', #16640 ) ;
#5290=DIRECTION ( 'NONE',  ( 0.000000000000000000, 0.000000000000000000, -1.000000000000000000 ) ) ;
#5294=CARTESIAN_POINT ( 'NONE',  ( 15.34956869069047869, 36.37910824616916017, -56.69201590313573291 ) ) ;
#5295=DIRECTION ( 'NONE',  ( -0.4166911066143236253, 0.000000000000000000, 0.9090481404571104651 ) ) ;
#5297=CARTESIAN_POINT ( 'NONE',  ( 7.017626609043924546, 33.27455722914837821, -41.44244536674933244 ) ) ;
#5298=ORIENTED_EDGE ( 'NONE', *, *, #13947, .F. ) ;
#5301=CARTESIAN_POINT ( 'NONE',  ( -21.63981290377905253, 13.82170478134237612, 58.49475859713705006 ) ) ;
#5304=CARTESIAN_POINT ( 'NONE',  ( 12.10743492717617364, 1.299801688893591267, 55.43551573822927026 ) ) ;
#5306=FACE_OUTER_BOUND ( 'NONE', #5955, .T. ) ;
#5307=ORIENTED_EDGE ( 'NONE', *, *, #11043, .F. ) ;
#5313=AXIS2_PLACEMENT_3D ( 'NONE', #15586, #2385, #7113 ) ;
#5314=CARTESIAN_POINT ( 'NONE',  ( 20.89754528720908411, 28.21939688025627291, 58.32034131438403790 ) ) ;
#5320=CARTESIAN_POINT ( 'NONE',  ( -7.505578006075204200, 1.461761173328241847, 55.63523492904089096 ) ) ;
#5328=CARTESIAN_POINT ( 'NONE',  ( -6.696867368503558448E-15, 40.00000000000000000, -48.73397172404479960 ) ) ;
#5330=CARTESIAN_POINT ( 'NONE',  ( 17.18568680885866584, 30.37812028685803156, 59.88587632367774205 ) ) ;
#5334=CARTESIAN_POINT ( 'NONE',  ( 15.50000000000024336, -2.516660498395250745, -105.0010000000000048 ) ) ;
#5337=ORIENTED_EDGE ( 'NONE', *, *, #20910, .F. ) ;
#5338=EDGE_LOOP ( 'NONE', ( #21977, #8939 ) ) ;
#5341=FACE_OUTER_BOUND ( 'NONE', #14223, .T. ) ;
#5344=DIRECTION ( 'NONE',  ( 0.000000000000000000, 0.000000000000000000, -1.000000000000000000 ) ) ;
#5346=AXIS2_PLACEMENT_3D ( 'NONE', #5168, #3676, #14059 ) ;
#5347=CARTESIAN_POINT ( 'NONE',  ( 1.943361993987648306, 39.97741573862661824, 50.18563611142815972 ) ) ;
#5353=CYLINDRICAL_SURFACE ( 'NONE', #19254, 18.00000000000000000 ) ;
#5357=CARTESIAN_POINT ( 'NONE',  ( -9.375631618502383802, 39.53999972426225185, 54.37753810704350599 ) ) ;
#5358=CARTESIAN_POINT ( 'NONE',  ( -34.99999999999980815, 26.00000000000000355, 54.99999999999922551 ) ) ;
#5359=DIRECTION ( 'NONE',  ( 0.000000000000000000, 0.000000000000000000, -1.000000000000000000 ) ) ;
#5360=VERTEX_POINT ( 'NONE', #15015 ) ;
#5367=AXIS2_PLACEMENT_3D ( 'NONE', #15335, #6641, #17520 ) ;
#5369=EDGE_CURVE ( 'NONE', #11978, #1700, #1279, .T. ) ;
#5374=AXIS2_PLACEMENT_3D ( 'NONE', #14380, #3540, #12550 ) ;
#5381=CARTESIAN_POINT ( 'NONE',  ( 14.68506606271058956, 16.91806408329021494, -45.68712064066588141 ) ) ;
#5383=CARTESIAN_POINT ( 'NONE',  ( 34.99999999999980815, 39.97500000000000142, 57.49999999999921840 ) ) ;
#5385=DIRECTION ( 'NONE',  ( 0.000000000000000000, 0.000000000000000000, -1.000000000000000000 ) ) ;
#5386=VERTEX_POINT ( 'NONE', #6442 ) ;
#5389=AXIS2_PLACEMENT_3D ( 'NONE', #11598, #6325, #10087 ) ;
#5392=EDGE_CURVE ( 'NONE', #18704, #13273, #18202, .T. ) ;
#5398=ORIENTED_EDGE ( 'NONE', *, *, #6147, .F. ) ;
#5399=CARTESIAN_POINT ( 'NONE',  ( 90.00000000000000000, 40.00000000000000000, -9.108981535246192915E-16 ) ) ;
#5401=CARTESIAN_POINT ( 'NONE',  ( -22.00000000000001421, 20.00000000000000355, 98.00000000000000000 ) ) ;
#5402=CARTESIAN_POINT ( 'NONE',  ( -9.952189117650787509, 40.00000000000000000, -53.64426396172093092 ) ) ;
#5405=EDGE_CURVE ( 'NONE', #15800, #19371, #2112, .T. ) ;
#5407=EDGE_CURVE ( 'NONE', #22593, #15748, #21137, .T. ) ;
#5409=AXIS2_PLACEMENT_3D ( 'NONE', #15480, #1636, #6914 ) ;
#5412=DIRECTION ( 'NONE',  ( -0.000000000000000000, -1.000000000000000000, -0.000000000000000000 ) ) ;
#5413=VECTOR ( 'NONE', #915, 1000.000000000000000 ) ;
#5414=AXIS2_PLACEMENT_3D ( 'NONE', #3527, #17487, #176 ) ;
#5416=AXIS2_PLACEMENT_3D ( 'NONE', #826, #14790, #6102 ) ;
#5419=ORIENTED_EDGE ( 'NONE', *, *, #4728, .T. ) ;
#5420=VERTEX_POINT ( 'NONE', #1850 ) ;
#5422=CARTESIAN_POINT ( 'NONE',  ( 22.41556111754670866, 20.62010838399688240, 58.66542762804075295 ) ) ;
#5423=CARTESIAN_POINT ( 'NONE',  ( 4.407762377731845760, 40.00000000000000711, -51.31072002866562798 ) ) ;
#5424=CARTESIAN_POINT ( 'NONE',  ( 5.708997389694868474, 39.99999999999998579, 51.95724523303017861 ) ) ;
#5425=CIRCLE ( 'NONE', #9088, 49.99999999999998579 ) ;
#5426=ORIENTED_EDGE ( 'NONE', *, *, #9879, .F. ) ;
#5427=CYLINDRICAL_SURFACE ( 'NONE', #14558, 6.499999999999999112 ) ;
#5429=ORIENTED_EDGE ( 'NONE', *, *, #4990, .T. ) ;
#5430=CARTESIAN_POINT ( 'NONE',  ( -17.21639554191075305, 34.43961005730908198, -57.30688911148506293 ) ) ;
#5433=EDGE_LOOP ( 'NONE', ( #8062, #555, #8875, #15349 ) ) ;
#5434=CARTESIAN_POINT ( 'NONE',  ( 8.349099696857463115, 1.803277857257797656, 53.93591755799671006 ) ) ;
#5438=CARTESIAN_POINT ( 'NONE',  ( -1.575045212608098932, 39.94053886632075745, 50.55745523153140653 ) ) ;
#5439=AXIS2_PLACEMENT_3D ( 'NONE', #22086, #20368, #6272 ) ;
#5440=CARTESIAN_POINT ( 'NONE',  ( -9.689843208404443686, 39.33333333333332860, 54.54983754392751649 ) ) ;
#5442=CARTESIAN_POINT ( 'NONE',  ( 15.91596560756312151, 32.12719615765404768, 56.91747558599882240 ) ) ;
#5448=ORIENTED_EDGE ( 'NONE', *, *, #13764, .F. ) ;
#5449=ORIENTED_EDGE ( 'NONE', *, *, #2466, .F. ) ;
#5456=DIRECTION ( 'NONE',  ( 0.000000000000000000, 0.000000000000000000, -1.000000000000000000 ) ) ;
#5457=LINE ( 'NONE', #19214, #19709 ) ;
#5458=CARTESIAN_POINT ( 'NONE',  ( 0.03495034244140499818, 39.99999280692916415, 48.76116143213860710 ) ) ;
#5460=ORIENTED_EDGE ( 'NONE', *, *, #9253, .F. ) ;
#5462=CARTESIAN_POINT ( 'NONE',  ( 90.00000000000000000, 40.00000000000000000, -9.108981535246192915E-16 ) ) ;
#5464=DIRECTION ( 'NONE',  ( 0.000000000000000000, 0.000000000000000000, 1.000000000000000000 ) ) ;
#5465=CARTESIAN_POINT ( 'NONE',  ( -90.00000000000000000, 40.00000000000000711, -9.108981535246192915E-16 ) ) ;
#5466=CARTESIAN_POINT ( 'NONE',  ( -8.215393105055671441, 1.749144060402865186, -56.08634520686066338 ) ) ;
#5476=CARTESIAN_POINT ( 'NONE',  ( 5.770190843054305851, -4.767707482279640807, -49.21533144468782695 ) ) ;
#5478=EDGE_CURVE ( 'NONE', #19994, #19216, #7609, .T. ) ;
#5479=AXIS2_PLACEMENT_3D ( 'NONE', #5730, #19381, #10636 ) ;
#5483=LINE ( 'NONE', #3770, #20780 ) ;
#5484=CARTESIAN_POINT ( 'NONE',  ( -14.68506606271061443, 23.08193591670982059, -45.68712064066588852 ) ) ;
#5485=EDGE_CURVE ( 'NONE', #19292, #6464, #22250, .T. ) ;
#5487=DIRECTION ( 'NONE',  ( -0.000000000000000000, 1.000000000000000000, -0.000000000000000000 ) ) ;
#5488=DIRECTION ( 'NONE',  ( -0.000000000000000000, -0.000000000000000000, -1.000000000000000000 ) ) ;
#5490=CARTESIAN_POINT ( 'NONE',  ( 35.00000000000000711, 2.142135623730931471, 50.00000000000000711 ) ) ;
#5491=EDGE_LOOP ( 'NONE', ( #11037, #12057, #20420, #21919 ) ) ;
#5493=CARTESIAN_POINT ( 'NONE',  ( 35.00000000000000000, 39.00000000000000711, 4.258610482196280173E-15 ) ) ;
#5494=CIRCLE ( 'NONE', #9883, 2.500000000000002220 ) ;
#5495=EDGE_CURVE ( 'NONE', #5750, #1187, #8997, .T. ) ;
#5498=ORIENTED_EDGE ( 'NONE', *, *, #18889, .F. ) ;
#5499=DIRECTION ( 'NONE',  ( 0.000000000000000000, -1.000000000000000000, 0.000000000000000000 ) ) ;
#5501=DIRECTION ( 'NONE',  ( 0.000000000000000000, 0.000000000000000000, 1.000000000000000000 ) ) ;
#5503=ORIENTED_EDGE ( 'NONE', *, *, #17511, .T. ) ;
#5507=CARTESIAN_POINT ( 'NONE',  ( 16.23964334364511686, 4.495128156857200352, -56.99255277661108465 ) ) ;
#5509=DIRECTION ( 'NONE',  ( 0.000000000000000000, 0.000000000000000000, -1.000000000000000000 ) ) ;
#5511=CARTESIAN_POINT ( 'NONE',  ( -1.387778780781445676E-14, 20.00000000000000000, -98.00000000000000000 ) ) ;
#5512=CARTESIAN_POINT ( 'NONE',  ( -1.387778780781445676E-14, 20.00000000000000000, -102.0000000000000142 ) ) ;
#5517=CARTESIAN_POINT ( 'NONE',  ( -5.004946378181865718, 0.5943096879531011290, 54.03132084814318858 ) ) ;
#5519=ORIENTED_EDGE ( 'NONE', *, *, #9290, .T. ) ;
#5525=CARTESIAN_POINT ( 'NONE',  ( 8.115805981708332340, 39.55796044940698408, -53.89994356748307780 ) ) ;
#5526=CARTESIAN_POINT ( 'NONE',  ( 6.043799192484581084, 40.00000000000000000, 52.11526431830142059 ) ) ;
#5527=ORIENTED_EDGE ( 'NONE', *, *, #22501, .T. ) ;
#5534=LINE ( 'NONE', #3829, #245 ) ;
#5538=ADVANCED_FACE ( 'NONE', ( #13743 ), #5092, .T. ) ;
#5539=DIRECTION ( 'NONE',  ( 0.000000000000000000, 0.000000000000000000, -1.000000000000000000 ) ) ;
#5541=ADVANCED_FACE ( 'NONE', ( #19938 ), #8843, .F. ) ;
#5543=CARTESIAN_POINT ( 'NONE',  ( 19.93949378746059864, 21.61607484719042205, 60.60748883510628104 ) ) ;
#5551=ORIENTED_EDGE ( 'NONE', *, *, #11758, .F. ) ;
#5552=ORIENTED_EDGE ( 'NONE', *, *, #1245, .F. ) ;
#5554=DIRECTION ( 'NONE',  ( 0.000000000000000000, -1.000000000000000000, 0.000000000000000000 ) ) ;
#5555=CARTESIAN_POINT ( 'NONE',  ( 5.833333333333328596, 33.81926995981416439, -40.61164310337066041 ) ) ;
#5557=CARTESIAN_POINT ( 'NONE',  ( 1.107481208796976979, 39.99270069324596477, 49.57628741752042600 ) ) ;
#5559=ADVANCED_FACE ( 'NONE', ( #17881 ), #5958, .F. ) ;
#5561=CARTESIAN_POINT ( 'NONE',  ( 10.60627602730578900, 0.5940385038083370040, -54.69850067894228118 ) ) ;
#5562=CARTESIAN_POINT ( 'NONE',  ( -9.193775066140551289, 40.00000000000001421, -53.40447181574799629 ) ) ;
#5564=CARTESIAN_POINT ( 'NONE',  ( 13.56354382738798847, 2.142135623730931471, -56.03997097393683191 ) ) ;
#5567=CIRCLE ( 'NONE', #9945, 2.524999999999999467 ) ;
#5568=EDGE_CURVE ( 'NONE', #10048, #7926, #14127, .T. ) ;
#5571=CYLINDRICAL_SURFACE ( 'NONE', #17335, 15.00000000000000000 ) ;
#5572=B_SPLINE_CURVE_WITH_KNOTS ( 'NONE', 3,
 ( #22188, #4996, #11527, #1207, #18978, #22416, #13448, #6262, #10021, #8205, #18857, #20470, #4778, #18743, #3049, #6709, #21972, #17013, #1323, #15285, #9692, #16679, #2826, #22312 ),
 .UNSPECIFIED., .F., .F.,
 ( 4, 2, 2, 2, 2, 2, 2, 2, 2, 2, 2, 4 ),
 ( 0.02614117015034102612, 0.02729036340605314401, 0.02843955666176526190, 0.03073794317318948727, 0.03188713642890159822, 0.03303632968461370917, 0.03533471619603793107, 0.03648390945175004896, 0.03763310270746215991, 0.03993148921888638181, 0.04222987573031060371, 0.04452826224173483255 ),
 .UNSPECIFIED. ) ;
#5573=CARTESIAN_POINT ( 'NONE',  ( -35.00000000000000000, 40.00000000000000000, 51.00000000000002842 ) ) ;
#5575=EDGE_LOOP ( 'NONE', ( #9937, #7329, #9315 ) ) ;
#5576=ORIENTED_EDGE ( 'NONE', *, *, #20522, .T. ) ;
#5577=CONICAL_SURFACE ( 'NONE', #5946, 2.525000000000110489, 0.7853981633971014453 ) ;
#5578=DIRECTION ( 'NONE',  ( 1.000000000000000000, 0.000000000000000000, 0.000000000000000000 ) ) ;
#5579=VECTOR ( 'NONE', #11270, 1000.000000000000000 ) ;
#5583=CARTESIAN_POINT ( 'NONE',  ( -14.04165170564761311, 5.752764646445623242, 58.83649392397244071 ) ) ;
#5584=CARTESIAN_POINT ( 'NONE',  ( -15.06716847275263937, 33.15945890355343550, -59.19951139074274238 ) ) ;
#5585=DIRECTION ( 'NONE',  ( -0.000000000000000000, -0.000000000000000000, -1.000000000000000000 ) ) ;
#5586=ORIENTED_EDGE ( 'NONE', *, *, #17086, .F. ) ;
#5587=DIRECTION ( 'NONE',  ( 0.000000000000000000, -1.000000000000000000, 0.000000000000000000 ) ) ;
#5588=DIRECTION ( 'NONE',  ( -0.000000000000000000, 1.000000000000000000, -0.000000000000000000 ) ) ;
#5589=CARTESIAN_POINT ( 'NONE',  ( -7.538500903810553488, 38.52938254314624800, -55.92181088654619714 ) ) ;
#5591=DIRECTION ( 'NONE',  ( 0.000000000000000000, -1.000000000000000000, 0.000000000000000000 ) ) ;
#5592=ORIENTED_EDGE ( 'NONE', *, *, #17408, .T. ) ;
#5594=DIRECTION ( 'NONE',  ( 0.8391477167891896460, 0.3845457931435838361, -0.3846500258456542198 ) ) ;
#5598=CARTESIAN_POINT ( 'NONE',  ( -42.50000000000000711, -12.00000000000000000, 47.50000000000000711 ) ) ;
#5599=B_SPLINE_CURVE_WITH_KNOTS ( 'NONE', 3,
 ( #8952, #588, #5517, #244, #12602, #7578 ),
 .UNSPECIFIED., .F., .F.,
 ( 4, 2, 4 ),
 ( 0.000000000000000000, 0.004604358499702467140, 0.009208716999404934281 ),
 .UNSPECIFIED. ) ;
#5600=EDGE_LOOP ( 'NONE', ( #17503, #10626, #9470, #219 ) ) ;
#5601=EDGE_CURVE ( 'NONE', #13103, #22583, #12352, .T. ) ;
#5604=CARTESIAN_POINT ( 'NONE',  ( -6.696867368503558448E-15, 0.000000000000000000, -48.73397172404479960 ) ) ;
#5606=VECTOR ( 'NONE', #1425, 1000.000000000000000 ) ;
#5608=ORIENTED_EDGE ( 'NONE', *, *, #2035, .F. ) ;
#5609=DIRECTION ( 'NONE',  ( 0.000000000000000000, 0.000000000000000000, -1.000000000000000000 ) ) ;
#5610=VECTOR ( 'NONE', #3443, 1000.000000000000000 ) ;
#5611=CARTESIAN_POINT ( 'NONE',  ( -12.10743492717932313, 1.299801688895240837, -55.43551573823073397 ) ) ;
#5614=CARTESIAN_POINT ( 'NONE',  ( -22.00000000000001421, 20.00000000000000000, -100.0000000000000000 ) ) ;
#5616=CARTESIAN_POINT ( 'NONE',  ( 21.93942599038054908, 24.73590942562830008, -58.56147853046843466 ) ) ;
#5618=ORIENTED_EDGE ( 'NONE', *, *, #3841, .T. ) ;
#5621=CARTESIAN_POINT ( 'NONE',  ( -6.264962414979408756, 39.74816732676359976, -52.94809031933390742 ) ) ;
#5622=ORIENTED_EDGE ( 'NONE', *, *, #15348, .F. ) ;
#5624=( BOUNDED_SURFACE ( )  B_SPLINE_SURFACE ( 3, 2, ( 
 ( #3590, #19613, #19397 ),
 ( #3923, #1752, #1860 ),
 ( #5304, #10549, #8841 ),
 ( #2305, #13050, #2655 ),
 ( #5864, #8036, #16508 ),
 ( #9630, #2544, #16277 ) ),
 .UNSPECIFIED., .F., .F., .F. ) 
 B_SPLINE_SURFACE_WITH_KNOTS ( ( 4, 2, 4 ),
 ( 3, 3 ),
 ( 0.000000000000000000, 0.002858401832368546482, 0.005716803664737092963 ),
 ( 0.000000000000000000, 1.000000000000000000 ),
 .UNSPECIFIED. ) 
 GEOMETRIC_REPRESENTATION_ITEM ( )  RATIONAL_B_SPLINE_SURFACE ( (
 ( 1.000000000000000000, 0.6290213284793376713, 1.000000000000000000),
 ( 1.000000000000000000, 0.6455195629501313537, 1.000000000000000000),
 ( 1.000000000000000000, 0.6615687397059663022, 1.000000000000000000),
 ( 1.000000000000000000, 0.6920701670989356513, 1.000000000000000000),
 ( 1.000000000000000000, 0.7065285139746015908, 1.000000000000000000),
 ( 1.000000000000000000, 0.7200096751079870794, 1.000000000000000000) ) ) 
 REPRESENTATION_ITEM ( '' )  SURFACE ( )  );
#5627=ADVANCED_FACE ( 'NONE', ( #16943 ), #11680, .F. ) ;
#5629=AXIS2_PLACEMENT_3D ( 'NONE', #16504, #2539, #9957 ) ;
#5631=EDGE_CURVE ( 'NONE', #11797, #10749, #20415, .T. ) ;
#5632=EDGE_LOOP ( 'NONE', ( #3691, #20196, #6618, #20738 ) ) ;
#5639=CARTESIAN_POINT ( 'NONE',  ( 7.325661905094778881, 40.00000000000000711, 52.68655283169726999 ) ) ;
#5646=CARTESIAN_POINT ( 'NONE',  ( -22.30616949375637503, 22.91984106672850174, -58.64191913087365293 ) ) ;
#5648=VERTEX_POINT ( 'NONE', #21776 ) ;
#5649=EDGE_CURVE ( 'NONE', #10179, #5750, #13030, .T. ) ;
#5651=EDGE_LOOP ( 'NONE', ( #1175, #11374, #16172, #18724 ) ) ;
#5655=CARTESIAN_POINT ( 'NONE',  ( 1.591932335265033587E-15, -4.923002280079127832E-27, 50.50395615645412306 ) ) ;
#5657=CARTESIAN_POINT ( 'NONE',  ( 90.00000000000000000, 40.00000000000000711, -9.108981535246192915E-16 ) ) ;
#5658=CARTESIAN_POINT ( 'NONE',  ( 20.00401474702854543, 19.84140115762890133, 58.14847693657672778 ) ) ;
#5662=CARTESIAN_POINT ( 'NONE',  ( 9.998533603140314696, 40.00000000000000000, -54.54288842742649734 ) ) ;
#5665=VECTOR ( 'NONE', #677, 1000.000000000000000 ) ;
#5669=ORIENTED_EDGE ( 'NONE', *, *, #13612, .T. ) ;
#5670=CYLINDRICAL_SURFACE ( 'NONE', #11792, 60.00000000000000000 ) ;
#5673=EDGE_CURVE ( 'NONE', #15024, #8904, #22644, .T. ) ;
#5679=VERTEX_POINT ( 'NONE', #7788 ) ;
#5680=LINE ( 'NONE', #14137, #19244 ) ;
#5682=FACE_OUTER_BOUND ( 'NONE', #13070, .T. ) ;
#5683=CARTESIAN_POINT ( 'NONE',  ( -20.00000000000002132, 20.48974789854086254, -60.62177826491083721 ) ) ;
#5684=AXIS2_PLACEMENT_3D ( 'NONE', #20645, #1514, #10427 ) ;
#5686=EDGE_CURVE ( 'NONE', #7816, #19292, #11451, .T. ) ;
#5688=CARTESIAN_POINT ( 'NONE',  ( -1.268121568164027657, 39.97056933375353083, 50.22305475358200511 ) ) ;
#5689=DIRECTION ( 'NONE',  ( 0.000000000000000000, 0.000000000000000000, 1.000000000000000000 ) ) ;
#5691=EDGE_CURVE ( 'NONE', #5386, #20516, #20795, .T. ) ;
#5692=ORIENTED_EDGE ( 'NONE', *, *, #18498, .T. ) ;
#5693=AXIS2_PLACEMENT_3D ( 'NONE', #16797, #11294, #12994 ) ;
#5695=EDGE_CURVE ( 'NONE', #16203, #19009, #1026, .T. ) ;
#5703=CARTESIAN_POINT ( 'NONE',  ( -19.74829075628835895, 16.81150045999882892, 60.56179516789185868 ) ) ;
#5704=CARTESIAN_POINT ( 'NONE',  ( -11.93214024655444838, 36.05624711372846036, -58.01435237789498700 ) ) ;
#5707=AXIS2_PLACEMENT_3D ( 'NONE', #1040, #13603, #8474 ) ;
#5710=DIRECTION ( 'NONE',  ( -1.000000000000000000, 0.000000000000000000, 0.000000000000000000 ) ) ;
#5713=DIRECTION ( 'NONE',  ( -0.000000000000000000, -0.000000000000000000, 1.000000000000000000 ) ) ;
#5720=CARTESIAN_POINT ( 'NONE',  ( 42.50000000000000711, -12.00000000000000000, -45.40000000000000568 ) ) ;
#5722=CIRCLE ( 'NONE', #22190, 2.499999999999998668 ) ;
#5724=CIRCLE ( 'NONE', #18535, 6.499999999999999112 ) ;
#5730=CARTESIAN_POINT ( 'NONE',  ( -42.50000000000000711, -12.00000000000000000, -47.50000000000000000 ) ) ;
#5740=ORIENTED_EDGE ( 'NONE', *, *, #4183, .F. ) ;
#5741=DIRECTION ( 'NONE',  ( 0.000000000000000000, -1.000000000000000000, 0.000000000000000000 ) ) ;
#5742=CARTESIAN_POINT ( 'NONE',  ( -9.062586715433361917, 2.130694986431509452, 54.31128890271796195 ) ) ;
#5743=CARTESIAN_POINT ( 'NONE',  ( -0.3255759151790424410, 39.99938828955776415, -48.98576778550931010 ) ) ;
#5744=AXIS2_PLACEMENT_3D ( 'NONE', #12715, #810, #7794 ) ;
#5748=DIRECTION ( 'NONE',  ( 0.4166911066143264564, 0.000000000000000000, -0.9090481404571091328 ) ) ;
#5750=VERTEX_POINT ( 'NONE', #3087 ) ;
#5757=EDGE_LOOP ( 'NONE', ( #19066, #16404 ) ) ;
#5762=ORIENTED_EDGE ( 'NONE', *, *, #18578, .T. ) ;
#5763=DIRECTION ( 'NONE',  ( 0.000000000000000000, 0.000000000000000000, 1.000000000000000000 ) ) ;
#5766=CARTESIAN_POINT ( 'NONE',  ( -1.143118858956962969, 0.005001482714649774057, 49.65374274205655780 ) ) ;
#5771=DIRECTION ( 'NONE',  ( 0.000000000000000000, 0.000000000000000000, 1.000000000000000000 ) ) ;
#5772=EDGE_LOOP ( 'NONE', ( #4067, #9159, #597 ) ) ;
#5777=VERTEX_POINT ( 'NONE', #17390 ) ;
#5779=CARTESIAN_POINT ( 'NONE',  ( 17.96644252022819188, 11.16803817567472201, 57.57522208103243599 ) ) ;
#5780=LINE ( 'NONE', #15964, #7778 ) ;
#5784=ORIENTED_EDGE ( 'NONE', *, *, #6712, .F. ) ;
#5790=VECTOR ( 'NONE', #17568, 1000.000000000000000 ) ;
#5791=CARTESIAN_POINT ( 'NONE',  ( -10.95789470854538372, 39.14627205512025654, -55.00167764528740122 ) ) ;
#5793=FACE_BOUND ( 'NONE', #19042, .T. ) ;
#5794=CIRCLE ( 'NONE', #12008, 58.99999999999994316 ) ;
#5795=ORIENTED_EDGE ( 'NONE', *, *, #18779, .F. ) ;
#5796=CARTESIAN_POINT ( 'NONE',  ( 10.30713387248560231, 2.842164160679857332, 57.27491564205545416 ) ) ;
#5797=CARTESIAN_POINT ( 'NONE',  ( 7.325260514639500961E-15, -4.648749848371387827, 45.43309249825157536 ) ) ;
#5801=CARTESIAN_POINT ( 'NONE',  ( 42.50000000000000711, -9.600000000000001421, 49.60000000000000853 ) ) ;
#5802=DIRECTION ( 'NONE',  ( 0.000000000000000000, 0.000000000000000000, 1.000000000000000000 ) ) ;
#5806=VECTOR ( 'NONE', #17418, 1000.000000000000000 ) ;
#5808=CARTESIAN_POINT ( 'NONE',  ( -3.981170799216933176, 39.90684832978752183, 51.58237208215641090 ) ) ;
#5813=EDGE_CURVE ( 'NONE', #862, #3734, #19017, .T. ) ;
#5817=AXIS2_PLACEMENT_3D ( 'NONE', #8053, #2561, #7817 ) ;
#5818=FACE_OUTER_BOUND ( 'NONE', #2469, .T. ) ;
#5824=CARTESIAN_POINT ( 'NONE',  ( -11.87139216507977224, 36.11857111619887206, -55.37976054165662987 ) ) ;
#5826=DIRECTION ( 'NONE',  ( -0.000000000000000000, -1.000000000000000000, -0.000000000000000000 ) ) ;
#5830=EDGE_LOOP ( 'NONE', ( #7004, #17103, #16908, #20604 ) ) ;
#5831=CARTESIAN_POINT ( 'NONE',  ( 35.00000000000058265, 26.00000000000000355, -55.00000000000076028 ) ) ;
#5836=ORIENTED_EDGE ( 'NONE', *, *, #22331, .F. ) ;
#5843=CARTESIAN_POINT ( 'NONE',  ( 6.257506482006864879, 40.00000000000000000, -52.21447511918912454 ) ) ;
#5845=CARTESIAN_POINT ( 'NONE',  ( 0.6620738645431283320, 39.99747006418269279, -49.24250857139721660 ) ) ;
#5846=CARTESIAN_POINT ( 'NONE',  ( 9.689843208404402830, 39.33333333333334991, 54.54983754392742412 ) ) ;
#5848=LINE ( 'NONE', #14189, #21913 ) ;
#5850=CARTESIAN_POINT ( 'NONE',  ( 14.99999999999998579, 20.00000000000000000, 101.0000000000000568 ) ) ;
#5851=CARTESIAN_POINT ( 'NONE',  ( -10.31465995609250186, 2.846668092512739001, -57.27881138849976139 ) ) ;
#5853=CARTESIAN_POINT ( 'NONE',  ( -90.00000000000000000, 26.00000000000000355, -9.108981535246192915E-16 ) ) ;
#5855=EDGE_CURVE ( 'NONE', #2582, #3905, #3227, .T. ) ;
#5858=FACE_OUTER_BOUND ( 'NONE', #2819, .T. ) ;
#5859=VERTEX_POINT ( 'NONE', #19361 ) ;
#5860=CYLINDRICAL_SURFACE ( 'NONE', #19284, 20.00000000000000000 ) ;
#5861=CARTESIAN_POINT ( 'NONE',  ( -11.05758567243163348, 3.294696707140393421, 55.18338768059884103 ) ) ;
#5862=CARTESIAN_POINT ( 'NONE',  ( -0.1974767274569673714, 39.99977542932850127, -48.88709713040997684 ) ) ;
#5864=CARTESIAN_POINT ( 'NONE',  ( 9.867969867544811535, 0.2954100743844931820, 54.30456930252214676 ) ) ;
#5866=EDGE_CURVE ( 'NONE', #9501, #14814, #11077, .T. ) ;
#5867=CARTESIAN_POINT ( 'NONE',  ( -9.852267639826644441, 31.31642578264289156, 43.21671877549179897 ) ) ;
#5868=DIRECTION ( 'NONE',  ( -0.000000000000000000, -0.000000000000000000, 1.000000000000000000 ) ) ;
#5869=CONICAL_SURFACE ( 'NONE', #9893, 57.00000000000002132, 0.7853981633974437271 ) ;
#5870=EDGE_LOOP ( 'NONE', ( #21915, #4926, #10252, #8989 ) ) ;
#5872=ORIENTED_EDGE ( 'NONE', *, *, #10237, .F. ) ;
#5878=CARTESIAN_POINT ( 'NONE',  ( -12.99999999999980282, -2.516660498395516310, -105.0010000000000048 ) ) ;
#5879=CARTESIAN_POINT ( 'NONE',  ( -42.50000000000000711, -9.600000000000001421, 49.60000000000000853 ) ) ;
#5881=DIRECTION ( 'NONE',  ( 0.000000000000000000, 0.000000000000000000, -1.000000000000000000 ) ) ;
#5888=ORIENTED_EDGE ( 'NONE', *, *, #14810, .F. ) ;
#5889=CARTESIAN_POINT ( 'NONE',  ( 3.171143452058838186, 39.94219392501161536, 51.05053595446507586 ) ) ;
#5891=EDGE_LOOP ( 'NONE', ( #22001, #12669 ) ) ;
#5893=CARTESIAN_POINT ( 'NONE',  ( 6.696867368503558448E-15, 39.00000000000000711, 48.73397172404481381 ) ) ;
#5898=ADVANCED_FACE ( 'NONE', ( #12676 ), #17622, .T. ) ;
#5901=ORIENTED_EDGE ( 'NONE', *, *, #637, .F. ) ;
#5902=ORIENTED_EDGE ( 'NONE', *, *, #16886, .F. ) ;
#5903=DIRECTION ( 'NONE',  ( -0.000000000000000000, -1.000000000000000000, -0.000000000000000000 ) ) ;
#5907=CARTESIAN_POINT ( 'NONE',  ( -32.89999999999981384, 28.00000000000000000, 54.99999999999922551 ) ) ;
#5912=DIRECTION ( 'NONE',  ( 8.659560562351929024E-17, -0.7071067811867928210, 0.7071067811863022134 ) ) ;
#5919=DIRECTION ( 'NONE',  ( -0.9012767464701780806, -2.276634065091486700E-15, -0.4332438415859253267 ) ) ;
#5921=VERTEX_POINT ( 'NONE', #10616 ) ;
#5927=VECTOR ( 'NONE', #19943, 1000.000000000000000 ) ;
#5928=CARTESIAN_POINT ( 'NONE',  ( 6.775279300855725495, 38.82186504314601194, 55.41168644275258970 ) ) ;
#5929=CARTESIAN_POINT ( 'NONE',  ( -10.60627602730584407, 0.5940385038083494385, -54.69850067894230250 ) ) ;
#5930=CARTESIAN_POINT ( 'NONE',  ( -1.575019415474304463, 39.98856485926602744, -49.93405284605607619 ) ) ;
#5934=EDGE_LOOP ( 'NONE', ( #22485, #16323 ) ) ;
#5936=CARTESIAN_POINT ( 'NONE',  ( -0.1564864144765418241, 40.00000000000000711, -48.92140276528787268 ) ) ;
#5942=DIRECTION ( 'NONE',  ( -1.000000000000000000, -0.000000000000000000, -0.000000000000000000 ) ) ;
#5943=EDGE_CURVE ( 'NONE', #10163, #7430, #12235, .T. ) ;
#5946=AXIS2_PLACEMENT_3D ( 'NONE', #16091, #19545, #400 ) ;
#5951=ORIENTED_EDGE ( 'NONE', *, *, #13007, .F. ) ;
#5952=CARTESIAN_POINT ( 'NONE',  ( 1.044236013776834060, 39.99351860983329487, -49.52927844032964089 ) ) ;
#5954=CARTESIAN_POINT ( 'NONE',  ( -35.00000000000000000, -5.000000000000000000, 1.387778780781445676E-14 ) ) ;
#5955=EDGE_LOOP ( 'NONE', ( #4087, #11962, #5551, #11753, #4287 ) ) ;
#5958=CYLINDRICAL_SURFACE ( 'NONE', #15278, 18.00000000000000000 ) ;
#5959=ORIENTED_EDGE ( 'NONE', *, *, #18442, .F. ) ;
#5961=CARTESIAN_POINT ( 'NONE',  ( -90.00000000000000000, 40.00000000000000711, -2.525000000000000355 ) ) ;
#5964=ORIENTED_EDGE ( 'NONE', *, *, #17873, .T. ) ;
#5965=CARTESIAN_POINT ( 'NONE',  ( -12.10743492717950609, 1.299801688895098506, 55.43551573823082634 ) ) ;
#5966=DIRECTION ( 'NONE',  ( -0.4332438415860033198, 0.000000000000000000, 0.9012767464701406661 ) ) ;
#5967=AXIS2_PLACEMENT_3D ( 'NONE', #21598, #9211, #19653 ) ;
#5968=ORIENTED_EDGE ( 'NONE', *, *, #9129, .T. ) ;
#5971=ORIENTED_EDGE ( 'NONE', *, *, #3335, .T. ) ;
#5973=AXIS2_PLACEMENT_3D ( 'NONE', #6839, #17477, #5230 ) ;
#5978=UNCERTAINTY_MEASURE_WITH_UNIT (LENGTH_MEASURE( 1.000000000000000082E-05 ), #6729, 'distance_accuracy_value', 'NONE');
#5981=CARTESIAN_POINT ( 'NONE',  ( 19.92971843794354214, 21.94076660514457444, -60.60536071356334276 ) ) ;
#5983=DIRECTION ( 'NONE',  ( -0.000000000000000000, -1.000000000000000000, -0.000000000000000000 ) ) ;
#5986=VERTEX_POINT ( 'NONE', #7760 ) ;
#5989=ORIENTED_EDGE ( 'NONE', *, *, #1104, .F. ) ;
#5992=CARTESIAN_POINT ( 'NONE',  ( 19.80871821058214266, 17.21148610482000407, -60.57629886234794014 ) ) ;
#5994=CARTESIAN_POINT ( 'NONE',  ( -9.952189117650851458, 40.00000000000000000, -53.64426396172072486 ) ) ;
#5998=CARTESIAN_POINT ( 'NONE',  ( -1.265314100866710527E-14, 40.00000000000000000, 48.73397172404481381 ) ) ;
#6001=ORIENTED_EDGE ( 'NONE', *, *, #7330, .F. ) ;
#6004=CARTESIAN_POINT ( 'NONE',  ( 15.91103418227299215, 35.86133518681679533, 56.88632568426859137 ) ) ;
#6005=FACE_OUTER_BOUND ( 'NONE', #14704, .T. ) ;
#6008=DIRECTION ( 'NONE',  ( -0.000000000000000000, -1.000000000000000000, -0.000000000000000000 ) ) ;
#6009=ORIENTED_EDGE ( 'NONE', *, *, #14053, .F. ) ;
#6010=EDGE_CURVE ( 'NONE', #7482, #5420, #19910, .T. ) ;
#6011=ORIENTED_EDGE ( 'NONE', *, *, #13624, .T. ) ;
#6018=CONICAL_SURFACE ( 'NONE', #15139, 2.524999999999999467, 0.7853981633974482790 ) ;
#6019=ADVANCED_FACE ( 'NONE', ( #16471 ), #11283, .F. ) ;
#6024=ORIENTED_EDGE ( 'NONE', *, *, #15419, .T. ) ;
#6026=DIRECTION ( 'NONE',  ( -0.000000000000000000, -1.000000000000000000, -0.000000000000000000 ) ) ;
#6027=CARTESIAN_POINT ( 'NONE',  ( 90.00000000000000000, 40.00000000000000000, -9.108981535246192915E-16 ) ) ;
#6033=CARTESIAN_POINT ( 'NONE',  ( -5.340789179572045242, 39.27722415257186839, 54.28402915905244441 ) ) ;
#6037=AXIS2_PLACEMENT_3D ( 'NONE', #9836, #16706, #1126 ) ;
#6038=VERTEX_POINT ( 'NONE', #18410 ) ;
#6039=DIRECTION ( 'NONE',  ( 0.000000000000000000, 0.000000000000000000, 1.000000000000000000 ) ) ;
#6043=CARTESIAN_POINT ( 'NONE',  ( 7.928388824789353251, 38.36675580713608014, 56.15749817958555923 ) ) ;
#6044=CARTESIAN_POINT ( 'NONE',  ( -12.82970538955584772, 1.687462484003157126, -55.75926248610263514 ) ) ;
#6045=CARTESIAN_POINT ( 'NONE',  ( -8.123074520535881859, 39.63120893085925189, -53.85470301846236651 ) ) ;
#6047=EDGE_CURVE ( 'NONE', #14638, #9888, #291, .T. ) ;
#6050=CARTESIAN_POINT ( 'NONE',  ( -11.68090480754633553, 3.765577839755389622, 57.90797000640144176 ) ) ;
#6051=DIRECTION ( 'NONE',  ( -0.000000000000000000, 1.000000000000000000, -0.000000000000000000 ) ) ;
#6062=DIRECTION ( 'NONE',  ( 0.000000000000000000, -1.000000000000000000, 0.000000000000000000 ) ) ;
#6067=VERTEX_POINT ( 'NONE', #8002 ) ;
#6070=CARTESIAN_POINT ( 'NONE',  ( 11.51194040401120056, 39.05862814753015044, 55.21283662269279091 ) ) ;
#6075=FACE_OUTER_BOUND ( 'NONE', #11465, .T. ) ;
#6077=CARTESIAN_POINT ( 'NONE',  ( -3.182710733240893486, 40.00000000000000711, 50.65274140376491374 ) ) ;
#6078=AXIS2_PLACEMENT_3D ( 'NONE', #1576, #8455, #5148 ) ;
#6079=DIRECTION ( 'NONE',  ( 0.000000000000000000, 0.000000000000000000, 1.000000000000000000 ) ) ;
#6082=CARTESIAN_POINT ( 'NONE',  ( 42.50000000000000711, -9.600000000000001421, 45.00000000000000711 ) ) ;
#6083=DIRECTION ( 'NONE',  ( 0.000000000000000000, 0.000000000000000000, -1.000000000000000000 ) ) ;
#6087=CARTESIAN_POINT ( 'NONE',  ( -9.579024991656975629, 31.54842267267896716, 43.05667825653220149 ) ) ;
#6090=CIRCLE ( 'NONE', #18894, 8.999999999999966249 ) ;
#6097=VERTEX_POINT ( 'NONE', #2619 ) ;
#6098=CARTESIAN_POINT ( 'NONE',  ( 19.98183132229265269, 20.98212305896295149, 60.61750244562277601 ) ) ;
#6099=CARTESIAN_POINT ( 'NONE',  ( -4.295527433237782828E-15, -1.236374842841486021, 48.24164917503448180 ) ) ;
#6101=CARTESIAN_POINT ( 'NONE',  ( 12.24744603029285273, 40.00000000000000000, 54.43639671998466412 ) ) ;
#6102=DIRECTION ( 'NONE',  ( 0.000000000000000000, 0.000000000000000000, 1.000000000000000000 ) ) ;
#6110=CARTESIAN_POINT ( 'NONE',  ( -21.43973101033765261, 13.38729130222877650, -58.44776001661259812 ) ) ;
#6111=DIRECTION ( 'NONE',  ( 1.768737661780273138E-15, 0.000000000000000000, 1.000000000000000000 ) ) ;
#6116=CARTESIAN_POINT ( 'NONE',  ( -1.437422297277388872E-14, 40.00000000000000000, 48.73397172404481381 ) ) ;
#6118=CARTESIAN_POINT ( 'NONE',  ( -3.230019253414518669E-15, -0.1273124286837649666, -49.60950288446434087 ) ) ;
#6120=EDGE_LOOP ( 'NONE', ( #8541, #17114 ) ) ;
#6121=CARTESIAN_POINT ( 'NONE',  ( 13.73196689449483721, 34.57679379660663699, 56.13071196757302772 ) ) ;
#6122=EDGE_CURVE ( 'NONE', #20378, #16159, #7397, .T. ) ;
#6124=CARTESIAN_POINT ( 'NONE',  ( 6.696867368504048330E-15, 5.000000000000000888, 38.73397172404480671 ) ) ;
#6125=PLANE ( 'NONE',  #2727 ) ;
#6127=AXIS2_PLACEMENT_3D ( 'NONE', #8350, #1136, #6522 ) ;
#6128=ORIENTED_EDGE ( 'NONE', *, *, #3298, .T. ) ;
#6130=ORIENTED_EDGE ( 'NONE', *, *, #11304, .T. ) ;
#6132=CARTESIAN_POINT ( 'NONE',  ( -8.331955809010631597, 38.18181818181817988, -56.36098470834072316 ) ) ;
#6134=CIRCLE ( 'NONE', #5040, 2.524999999999999467 ) ;
#6137=LINE ( 'NONE', #9121, #8186 ) ;
#6138=ORIENTED_EDGE ( 'NONE', *, *, #7212, .T. ) ;
#6145=DIRECTION ( 'NONE',  ( 0.000000000000000000, 0.000000000000000000, 1.000000000000000000 ) ) ;
#6146=CARTESIAN_POINT ( 'NONE',  ( -0.4445462163336120764, 39.99884035387562875, 49.07689293423401011 ) ) ;
#6147=EDGE_CURVE ( 'NONE', #15662, #20449, #21896, .T. ) ;
#6150=CARTESIAN_POINT ( 'NONE',  ( -6.450249579240430187, 39.75604022694633954, 53.02614836873388526 ) ) ;
#6151=AXIS2_PLACEMENT_3D ( 'NONE', #1274, #22258, #1163 ) ;
#6154=ORIENTED_EDGE ( 'NONE', *, *, #22279, .F. ) ;
#6155=AXIS2_PLACEMENT_3D ( 'NONE', #12265, #6665, #8386 ) ;
#6157=VECTOR ( 'NONE', #22307, 1000.000000000000000 ) ;
#6158=CIRCLE ( 'NONE', #2872, 9.000000000000003553 ) ;
#6159=EDGE_LOOP ( 'NONE', ( #18517, #19538, #7255, #22299 ) ) ;
#6160=CARTESIAN_POINT ( 'NONE',  ( -20.11496009237101745, 10.03305173526369209, 58.12476682723770693 ) ) ;
#6163=ADVANCED_FACE ( 'NONE', ( #19524 ), #6524, .F. ) ;
#6166=CARTESIAN_POINT ( 'NONE',  ( 3.581684221278998451E-14, -0.5379438610623193950, 48.80684069443805839 ) ) ;
#6168=CARTESIAN_POINT ( 'NONE',  ( -8.957567394277941020, 39.56957037178317904, -54.21303306609684114 ) ) ;
#6170=AXIS2_PLACEMENT_3D ( 'NONE', #3038, #20343, #4766 ) ;
#6172=VERTEX_POINT ( 'NONE', #3499 ) ;
#6173=CARTESIAN_POINT ( 'NONE',  ( -2.546974693918181654, 39.84782899243123921, -51.61921092574151970 ) ) ;
#6174=FACE_OUTER_BOUND ( 'NONE', #7029, .T. ) ;
#6177=VERTEX_POINT ( 'NONE', #1884 ) ;
#6185=DIRECTION ( 'NONE',  ( 0.000000000000000000, 0.000000000000000000, 1.000000000000000000 ) ) ;
#6186=CARTESIAN_POINT ( 'NONE',  ( 4.873427793009105002, 40.00000000000000000, -51.54633075627398853 ) ) ;
#6188=CARTESIAN_POINT ( 'NONE',  ( 0.2719366648872892367, 39.99956353068301240, -48.94448570199384108 ) ) ;
#6190=CARTESIAN_POINT ( 'NONE',  ( 9.952189117650823036, 40.00000000000000000, 53.64426396172073197 ) ) ;
#6192=DIRECTION ( 'NONE',  ( 0.000000000000000000, 0.000000000000000000, 1.000000000000000000 ) ) ;
#6195=CARTESIAN_POINT ( 'NONE',  ( -9.225358738174124440, 39.40776783337060607, 54.37884419088918975 ) ) ;
#6198=ORIENTED_EDGE ( 'NONE', *, *, #4183, .T. ) ;
#6201=CARTESIAN_POINT ( 'NONE',  ( -0.03103604280932474244, 39.99999434194312897, -48.75811830434601291 ) ) ;
#6204=CARTESIAN_POINT ( 'NONE',  ( -15.00000000000001066, 20.77286304060557853, 45.82575694955839651 ) ) ;
#6208=VERTEX_POINT ( 'NONE', #46 ) ;
#6212=CARTESIAN_POINT ( 'NONE',  ( 17.90966157241560452, 28.91510314404816384, -60.08313820791175885 ) ) ;
#6213=ADVANCED_FACE ( 'NONE', ( #17576 ), #6634, .F. ) ;
#6216=CARTESIAN_POINT ( 'NONE',  ( -34.99999999999999289, -5.000000000000000000, -57.00000000000000711 ) ) ;
#6219=CYLINDRICAL_SURFACE ( 'NONE', #11672, 6.499999999999999112 ) ;
#6224=DIRECTION ( 'NONE',  ( 8.659560562355114050E-17, 0.7071067811865326957, -0.7071067811865622277 ) ) ;
#6225=AXIS2_PLACEMENT_3D ( 'NONE', #1390, #11805, #6775 ) ;
#6226=CARTESIAN_POINT ( 'NONE',  ( 17.38307674301854533, 10.07685590252457253, -59.93367040492843500 ) ) ;
#6228=FACE_OUTER_BOUND ( 'NONE', #16783, .T. ) ;
#6229=CARTESIAN_POINT ( 'NONE',  ( 1.575045212608050749, 39.94053886632075745, -50.55745523153133547 ) ) ;
#6231=CARTESIAN_POINT ( 'NONE',  ( 5.702716825708685100, 39.17357718829572377, 54.58701425222751169 ) ) ;
#6232=CARTESIAN_POINT ( 'NONE',  ( 0.2893518482366595479, -0.01224439107861633597, -48.63017502620383681 ) ) ;
#6236=CIRCLE ( 'NONE', #10239, 2.525000000000110489 ) ;
#6237=CARTESIAN_POINT ( 'NONE',  ( 11.24237306623960819, 36.54654314592769282, 57.72256821685510175 ) ) ;
#6239=CARTESIAN_POINT ( 'NONE',  ( 19.66964734151795113, 9.174855960407793276, -58.00890637771954772 ) ) ;
#6245=EDGE_LOOP ( 'NONE', ( #4620, #15567, #19165, #4649 ) ) ;
#6248=ADVANCED_FACE ( 'NONE', ( #2103 ), #16787, .F. ) ;
#6249=VERTEX_POINT ( 'NONE', #21590 ) ;
#6257=DIRECTION ( 'NONE',  ( 1.049727191138618326E-16, -0.5150380749100547106, 0.8571673007021120005 ) ) ;
#6259=CARTESIAN_POINT ( 'NONE',  ( -0.2369887982023440309, 39.99966998679947494, 48.91756878588413571 ) ) ;
#6260=VECTOR ( 'NONE', #11248, 1000.000000000000000 ) ;
#6262=CARTESIAN_POINT ( 'NONE',  ( -14.17374118098246605, 15.07546459525164728, 45.45638825402603089 ) ) ;
#6265=ORIENTED_EDGE ( 'NONE', *, *, #12250, .F. ) ;
#6268=CARTESIAN_POINT ( 'NONE',  ( -19.98434069128082058, 21.18673122687496502, 60.61816909402018183 ) ) ;
#6272=DIRECTION ( 'NONE',  ( 0.000000000000000000, 0.000000000000000000, -1.000000000000000000 ) ) ;
#6274=EDGE_CURVE ( 'NONE', #3399, #18007, #2455, .T. ) ;
#6276=CARTESIAN_POINT ( 'NONE',  ( 5.666159602074075430, 39.18446031140960883, 54.55708815122284250 ) ) ;
#6277=CARTESIAN_POINT ( 'NONE',  ( -2.881553265153760979, 39.80724590269267082, -51.34430246875412962 ) ) ;
#6278=DIRECTION ( 'NONE',  ( 0.000000000000000000, 1.000000000000000000, 0.000000000000000000 ) ) ;
#6282=CARTESIAN_POINT ( 'NONE',  ( -11.17438353593063560, 39.11312751358374840, 55.08132213033135116 ) ) ;
#6283=DIRECTION ( 'NONE',  ( 0.000000000000000000, 0.000000000000000000, -1.000000000000000000 ) ) ;
#6285=ORIENTED_EDGE ( 'NONE', *, *, #21853, .T. ) ;
#6290=DIRECTION ( 'NONE',  ( -0.000000000000000000, -0.000000000000000000, -1.000000000000000000 ) ) ;
#6292=CARTESIAN_POINT ( 'NONE',  ( 6.094655612023198721, 39.99999999999999289, -52.13899149650791998 ) ) ;
#6294=CARTESIAN_POINT ( 'NONE',  ( 4.591787867733965633, 39.86870494181058433, -51.95898231442010484 ) ) ;
#6296=ADVANCED_FACE ( 'NONE', ( #11260 ), #13101, .T. ) ;
#6300=CARTESIAN_POINT ( 'NONE',  ( -6.215602297253691511, 39.75345783577535741, 52.92318667896167739 ) ) ;
#6301=CARTESIAN_POINT ( 'NONE',  ( 13.33780792070359666, 2.142135623730922589, -45.06383732350882809 ) ) ;
#6302=VERTEX_POINT ( 'NONE', #14458 ) ;
#6307=ORIENTED_EDGE ( 'NONE', *, *, #4969, .T. ) ;
#6308=CIRCLE ( 'NONE', #1186, 4.000000000000000000 ) ;
#6309=DIRECTION ( 'NONE',  ( 0.000000000000000000, 0.000000000000000000, -1.000000000000000000 ) ) ;
#6310=FACE_OUTER_BOUND ( 'NONE', #7965, .T. ) ;
#6315=VERTEX_POINT ( 'NONE', #9323 ) ;
#6316=CARTESIAN_POINT ( 'NONE',  ( 16.96028156848954183, 30.61033039275981338, -59.80781543853671423 ) ) ;
#6317=DIRECTION ( 'NONE',  ( -3.525918314278899701E-15, 0.000000000000000000, 1.000000000000000000 ) ) ;
#6323=VERTEX_POINT ( 'NONE', #4170 ) ;
#6325=DIRECTION ( 'NONE',  ( -0.000000000000000000, -1.000000000000000000, -0.000000000000000000 ) ) ;
#6327=CARTESIAN_POINT ( 'NONE',  ( -13.75658951623324455, 14.00814961052207686, -45.26303799332215050 ) ) ;
#6328=CONICAL_SURFACE ( 'NONE', #12897, 2.524999999999999467, 0.7853981633974482790 ) ;
#6331=CARTESIAN_POINT ( 'NONE',  ( -15.50000000000011013, 42.51666049839536043, 60.00099999999999767 ) ) ;
#6333=DIRECTION ( 'NONE',  ( -0.000000000000000000, 1.000000000000000000, 0.000000000000000000 ) ) ;
#6334=CARTESIAN_POINT ( 'NONE',  ( 6.775203351379166961, 38.82189279864962828, -55.41163305959238983 ) ) ;
#6338=CARTESIAN_POINT ( 'NONE',  ( -7.577104390338837980, -0.4826542685308990444, 53.01683071947941528 ) ) ;
#6340=CARTESIAN_POINT ( 'NONE',  ( 10.55176496409977283, 37.02956028564562985, 54.80914071361393525 ) ) ;
#6341=DIRECTION ( 'NONE',  ( -0.000000000000000000, 1.000000000000000000, -0.000000000000000000 ) ) ;
#6344=CARTESIAN_POINT ( 'NONE',  ( 20.01613897800084985, 20.29830884309071948, -58.15166638930550391 ) ) ;
#6345=CIRCLE ( 'NONE', #17308, 20.00000000000000000 ) ;
#6348=ORIENTED_EDGE ( 'NONE', *, *, #3893, .F. ) ;
#6350=CARTESIAN_POINT ( 'NONE',  ( 10.44987231559219509, 39.22455541040593374, 54.81340832989639722 ) ) ;
#6352=EDGE_CURVE ( 'NONE', #19351, #3791, #12570, .T. ) ;
#6353=ORIENTED_EDGE ( 'NONE', *, *, #15331, .T. ) ;
#6354=CARTESIAN_POINT ( 'NONE',  ( -42.50000000000000711, -5.000000000000000000, -47.50000000000000000 ) ) ;
#6355=DIRECTION ( 'NONE',  ( 0.000000000000000000, 0.000000000000000000, 1.000000000000000000 ) ) ;
#6356=EDGE_LOOP ( 'NONE', ( #17357, #7718 ) ) ;
#6358=CARTESIAN_POINT ( 'NONE',  ( 10.60627602730290242, 0.5940385038070811197, 54.69850067894081036 ) ) ;
#6359=VECTOR ( 'NONE', #9597, 1000.000000000000000 ) ;
#6362=CIRCLE ( 'NONE', #19173, 2.500000000000002220 ) ;
#6365=LINE ( 'NONE', #642, #21071 ) ;
#6366=EDGE_CURVE ( 'NONE', #18860, #6323, #16417, .T. ) ;
#6368=CIRCLE ( 'NONE', #2713, 2.500000000000002220 ) ;
#6369=CONICAL_SURFACE ( 'NONE', #4901, 17.00000000000001421, 0.7853981633974603804 ) ;
#6370=DIRECTION ( 'NONE',  ( -1.000000000000000000, 0.000000000000000000, 0.000000000000000000 ) ) ;
#6371=EDGE_LOOP ( 'NONE', ( #10254, #12126, #33, #7562 ) ) ;
#6372=ORIENTED_EDGE ( 'NONE', *, *, #22158, .F. ) ;
#6375=CARTESIAN_POINT ( 'NONE',  ( -19.66964734151719085, 9.174855960407388267, 58.00890637771936298 ) ) ;
#6378=CARTESIAN_POINT ( 'NONE',  ( -11.68090480754633731, 3.765577839755393619, -57.90797000640141334 ) ) ;
#6379=DIRECTION ( 'NONE',  ( 0.000000000000000000, 0.000000000000000000, -1.000000000000000000 ) ) ;
#6382=VECTOR ( 'NONE', #9045, 1000.000000000000000 ) ;
#6383=CARTESIAN_POINT ( 'NONE',  ( -23.50000000000001066, 19.99999999999982947, -100.0000000000000000 ) ) ;
#6386=ADVANCED_FACE ( 'NONE', ( #19930 ), #21419, .F. ) ;
#6387=CARTESIAN_POINT ( 'NONE',  ( 9.377138775072179300, -4.928932188134423242, 51.00555535510625305 ) ) ;
#6389=DIRECTION ( 'NONE',  ( 0.000000000000000000, 0.000000000000000000, 1.000000000000000000 ) ) ;
#6390=EDGE_CURVE ( 'NONE', #6724, #18961, #8207, .T. ) ;
#6394=CIRCLE ( 'NONE', #14373, 2.500000000000002220 ) ;
#6405=CARTESIAN_POINT ( 'NONE',  ( -10.27431133777638550, -4.928932188134511172, 51.43682631505698311 ) ) ;
#6412=CARTESIAN_POINT ( 'NONE',  ( -13.06496334682255167, 4.761428254742599897, -58.49034434778481994 ) ) ;
#6413=CARTESIAN_POINT ( 'NONE',  ( -10.63866000424708602, 30.58060543830995570, -43.66469350997155630 ) ) ;
#6417=CYLINDRICAL_SURFACE ( 'NONE', #5367, 2.099999999999997868 ) ;
#6422=ORIENTED_EDGE ( 'NONE', *, *, #6998, .F. ) ;
#6423=ADVANCED_FACE ( 'NONE', ( #14645 ), #796, .F. ) ;
#6425=DIRECTION ( 'NONE',  ( -1.000000000000000000, 0.000000000000000000, 0.000000000000000000 ) ) ;
#6427=AXIS2_PLACEMENT_3D ( 'NONE', #4637, #13420, #22622 ) ;
#6428=VERTEX_POINT ( 'NONE', #19821 ) ;
#6431=ORIENTED_EDGE ( 'NONE', *, *, #18017, .T. ) ;
#6435=CARTESIAN_POINT ( 'NONE',  ( 9.958219108218454352, 37.43657071496331668, -57.18097912447547060 ) ) ;
#6437=DIRECTION ( 'NONE',  ( -0.000000000000000000, -0.000000000000000000, 1.000000000000000000 ) ) ;
#6439=CARTESIAN_POINT ( 'NONE',  ( -42.50000000000000711, -12.00000000000000000, -45.40000000000000568 ) ) ;
#6440=ORIENTED_EDGE ( 'NONE', *, *, #8868, .T. ) ;
#6441=CARTESIAN_POINT ( 'NONE',  ( -35.00000000000000000, 40.00000000000000000, -59.99999999999998579 ) ) ;
#6442=CARTESIAN_POINT ( 'NONE',  ( 17.99999999999998579, 20.00000000000000355, 103.0000000000000284 ) ) ;
#6444=CARTESIAN_POINT ( 'NONE',  ( -11.37797799463865722, 10.21854205506534008, -44.06891764425669322 ) ) ;
#6446=EDGE_CURVE ( 'NONE', #6315, #8022, #3811, .T. ) ;
#6447=DIRECTION ( 'NONE',  ( 0.000000000000000000, 0.000000000000000000, 1.000000000000000000 ) ) ;
#6450=DIRECTION ( 'NONE',  ( 0.000000000000000000, 0.000000000000000000, 1.000000000000000000 ) ) ;
#6451=ORIENTED_EDGE ( 'NONE', *, *, #16328, .T. ) ;
#6452=CARTESIAN_POINT ( 'NONE',  ( 6.261274683082145742, 0.9579800028911629184, -54.84444022978222932 ) ) ;
#6453=AXIS2_PLACEMENT_3D ( 'NONE', #11601, #8391, #4844 ) ;
#6454=AXIS2_PLACEMENT_3D ( 'NONE', #1222, #9930, #22550 ) ;
#6456=AXIS2_PLACEMENT_3D ( 'NONE', #22586, #13843, #14172 ) ;
#6461=AXIS2_PLACEMENT_3D ( 'NONE', #5493, #440, #19818 ) ;
#6462=CARTESIAN_POINT ( 'NONE',  ( 19.66835476179213416, 23.72826198822077615, -58.05955247658420149 ) ) ;
#6463=EDGE_LOOP ( 'NONE', ( #747, #17147, #21994, #860 ) ) ;
#6464=VERTEX_POINT ( 'NONE', #13147 ) ;
#6467=EDGE_CURVE ( 'NONE', #17839, #9501, #4467, .T. ) ;
#6468=VERTEX_POINT ( 'NONE', #11445 ) ;
#6471=DIRECTION ( 'NONE',  ( -0.000000000000000000, -1.000000000000000000, -0.000000000000000000 ) ) ;
#6472=CARTESIAN_POINT ( 'NONE',  ( -10.27431133777642458, -4.928932188134513837, -51.43682631505698311 ) ) ;
#6477=EDGE_LOOP ( 'NONE', ( #18131, #3618, #5208, #606 ) ) ;
#6478=FACE_OUTER_BOUND ( 'NONE', #20915, .T. ) ;
#6482=CIRCLE ( 'NONE', #22243, 2.500000000000002220 ) ;
#6483=DIRECTION ( 'NONE',  ( -0.000000000000000000, -0.000000000000000000, -1.000000000000000000 ) ) ;
#6489=CARTESIAN_POINT ( 'NONE',  ( -16.98435752850986091, 5.286895767878122321, 57.23469700293563278 ) ) ;
#6491=CIRCLE ( 'NONE', #1732, 2.099999999999997868 ) ;
#6493=CARTESIAN_POINT ( 'NONE',  ( -20.00000000000002487, 18.38876824873586457, -60.62177826491085142 ) ) ;
#6499=CARTESIAN_POINT ( 'NONE',  ( -4.769735313644264174, 39.99999999999999289, -51.49386057199703970 ) ) ;
#6504=AXIS2_PLACEMENT_3D ( 'NONE', #11704, #9973, #4498 ) ;
#6505=CIRCLE ( 'NONE', #15272, 57.00000000000002132 ) ;
#6510=DIRECTION ( 'NONE',  ( -0.000000000000000000, 1.000000000000000000, -0.000000000000000000 ) ) ;
#6511=EDGE_CURVE ( 'NONE', #17407, #15147, #16255, .T. ) ;
#6517=ADVANCED_FACE ( 'NONE', ( #20277 ), #6018, .F. ) ;
#6518=ADVANCED_FACE ( 'NONE', ( #11674 ), #22317, .T. ) ;
#6519=EDGE_CURVE ( 'NONE', #9264, #15847, #13484, .T. ) ;
#6522=DIRECTION ( 'NONE',  ( 0.000000000000000000, 0.000000000000000000, -1.000000000000000000 ) ) ;
#6523=EDGE_LOOP ( 'NONE', ( #4100, #13192, #20535, #17542 ) ) ;
#6524=CONICAL_SURFACE ( 'NONE', #19343, 15.99999999999993072, 0.7853981633974415066 ) ;
#6526=B_SPLINE_CURVE_WITH_KNOTS ( 'NONE', 3,
 ( #8440, #1217, #8326, #22201, #15408, #6721, #15300, #19550, #5130, #15522, #15642, #19215, #1904, #20823, #8548, #13916, #22546, #17706, #8884, #14254, #14018, #6841, #13806, #293, #12102, #3640, #8786, #65, #8665, #7289, #21042, #10367, #21266, #5347, #19097, #17598, #5557, #21154, #3522, #3405, #12322, #168, #15981, #17363, #1683, #19333, #1561, #12536, #10594, #3853, #17251, #12430, #10700, #15858, #22671, #6958, #20933, #5232, #10483, #7166, #12213, #17482, #1801, #2012, #5458, #14135, #9000, #15755, #7055, #19442, #3745, #11288, #9570, #12876 ),
 .UNSPECIFIED., .F., .F.,
 ( 4, 2, 1, 2, 2, 1, 1, 2, 2, 2, 2, 1, 1, 1, 1, 1, 2, 2, 2, 1, 1, 1, 1, 1, 2, 2, 1, 1, 1, 1, 2, 2, 1, 1, 2, 2, 1, 2, 2, 2, 2, 1, 1, 2, 2, 2, 2, 4 ),
 ( 0.000000000000000000, 0.2499923706054147932, 0.2812414169310917256, 0.2851475477218011756, 0.2871006131171558451, 0.2890536785125104591, 0.2968659400939309134, 0.3124904632567707674, 0.3749885559081321817, 0.4999847412108561207, 0.5019378066062117894, 0.5038908720015674580, 0.5077970027922775742, 0.5156092643736978065, 0.5312337875365372719, 0.5624828338622163137, 0.6249809265135745084, 0.7499771118162896766, 0.7519301772116454563, 0.7538832426070012360, 0.7577893733977127955, 0.7656016349791360254, 0.7812261581419835954, 0.8124752044676776253, 0.8749732971190646857, 0.8769263625144214647, 0.8788794279097782436, 0.8827855587004908022, 0.8905978202819156975, 0.9062223434447642667, 0.9374713897704604060, 0.9413775205611728536, 0.9452836513518851902, 0.9530959129333099744, 0.9687204360961596539, 0.9726265668868717684, 0.9765326976775839940, 0.9843449592590070019, 0.9882510900497186723, 0.9921572208404302318, 0.9926454871892690379, 0.9931337535381078441, 0.9941102862357854564, 0.9960633516311395708, 0.9970398843288234003, 0.9980164170265072299, 0.9989929497241910594, 0.9999694824218750000 ),
 .UNSPECIFIED. ) ;
#6527=AXIS2_PLACEMENT_3D ( 'NONE', #16903, #6823, #8423 ) ;
#6529=CARTESIAN_POINT ( 'NONE',  ( 2.114046819835705637, 34.88523765466241855, -38.90380387758577996 ) ) ;
#6531=CARTESIAN_POINT ( 'NONE',  ( -18.94034750358418862, 13.51583961449410154, -57.85890765540866454 ) ) ;
#6534=LINE ( 'NONE', #13160, #5927 ) ;
#6538=CARTESIAN_POINT ( 'NONE',  ( 35.00000000000000000, -5.000000000000000000, 4.258610482196280173E-15 ) ) ;
#6539=DIRECTION ( 'NONE',  ( 0.000000000000000000, 0.000000000000000000, 1.000000000000000000 ) ) ;
#6540=ORIENTED_EDGE ( 'NONE', *, *, #10743, .F. ) ;
#6541=VECTOR ( 'NONE', #7566, 1000.000000000000000 ) ;
#6546=AXIS2_PLACEMENT_3D ( 'NONE', #12072, #6803, #10330 ) ;
#6550=VERTEX_POINT ( 'NONE', #20602 ) ;
#6558=ORIENTED_EDGE ( 'NONE', *, *, #2249, .T. ) ;
#6559=LINE ( 'NONE', #15464, #5806 ) ;
#6560=CARTESIAN_POINT ( 'NONE',  ( 6.696867368503558448E-15, 0.000000000000000000, 48.73397172404481381 ) ) ;
#6561=AXIS2_PLACEMENT_3D ( 'NONE', #11707, #14899, #1166 ) ;
#6565=CARTESIAN_POINT ( 'NONE',  ( 90.00000000000000000, 26.00000000000000355, -2.099999999999991651 ) ) ;
#6566=CARTESIAN_POINT ( 'NONE',  ( 9.226606573888423313, 39.40757736536860278, 54.37932754215746911 ) ) ;
#6567=ORIENTED_EDGE ( 'NONE', *, *, #10840, .F. ) ;
#6568=CARTESIAN_POINT ( 'NONE',  ( 34.99999999999980815, 39.97500000000000142, 54.99999999999922551 ) ) ;
#6569=ADVANCED_FACE ( 'NONE', ( #17161 ), #9726, .F. ) ;
#6571=DIRECTION ( 'NONE',  ( -0.000000000000000000, -1.000000000000000000, -0.000000000000000000 ) ) ;
#6572=CARTESIAN_POINT ( 'NONE',  ( -15.67632863000013188, 36.06985656533339579, 56.80410608597896527 ) ) ;
#6574=LINE ( 'NONE', #8399, #14884 ) ;
#6577=CARTESIAN_POINT ( 'NONE',  ( 17.83526554138365583, 10.93913794110402726, -60.06225905488081906 ) ) ;
#6578=AXIS2_PLACEMENT_3D ( 'NONE', #3622, #1996, #12629 ) ;
#6579=VERTEX_POINT ( 'NONE', #16716 ) ;
#6581=ORIENTED_EDGE ( 'NONE', *, *, #22627, .F. ) ;
#6582=DIRECTION ( 'NONE',  ( -0.000000000000000000, -1.000000000000000000, -0.000000000000000000 ) ) ;
#6585=LINE ( 'NONE', #20115, #10717 ) ;
#6586=DIRECTION ( 'NONE',  ( -0.000000000000000000, 1.000000000000000000, -0.000000000000000000 ) ) ;
#6594=LINE ( 'NONE', #11970, #12368 ) ;
#6596=CARTESIAN_POINT ( 'NONE',  ( -15.27654436812520977, 32.91718622474422773, -59.27094897435731014 ) ) ;
#6603=EDGE_LOOP ( 'NONE', ( #12285, #12509, #20371 ) ) ;
#6604=CARTESIAN_POINT ( 'NONE',  ( -22.04638094649398639, 24.21359277922483244, 58.58544938243663580 ) ) ;
#6607=CARTESIAN_POINT ( 'NONE',  ( -11.70544581405715512, 40.00000000000000000, 54.22116824785030076 ) ) ;
#6610=EDGE_LOOP ( 'NONE', ( #19157, #21925 ) ) ;
#6612=CARTESIAN_POINT ( 'NONE',  ( -8.604786193496984481, 40.00000000000001421, -53.19510613257067178 ) ) ;
#6614=CARTESIAN_POINT ( 'NONE',  ( 34.99999999999980815, 26.00000000000000355, 52.89999999999922409 ) ) ;
#6615=ORIENTED_EDGE ( 'NONE', *, *, #18744, .T. ) ;
#6617=EDGE_CURVE ( 'NONE', #5122, #16507, #2353, .T. ) ;
#6618=ORIENTED_EDGE ( 'NONE', *, *, #3412, .T. ) ;
#6621=DIRECTION ( 'NONE',  ( 0.000000000000000000, 0.000000000000000000, -1.000000000000000000 ) ) ;
#6622=DIRECTION ( 'NONE',  ( 0.000000000000000000, 1.000000000000000000, 0.000000000000000000 ) ) ;
#6629=CARTESIAN_POINT ( 'NONE',  ( 35.00000000000058265, 40.00000000000000711, -57.52500000000076597 ) ) ;
#6630=ORIENTED_EDGE ( 'NONE', *, *, #14554, .F. ) ;
#6633=EDGE_CURVE ( 'NONE', #15147, #11978, #18072, .T. ) ;
#6634=( BOUNDED_SURFACE ( )  B_SPLINE_SURFACE ( 3, 2, ( 
 ( #21132, #5434, #7265 ),
 ( #12411, #19422, #10674 ),
 ( #17680, #613, #19980 ),
 ( #19867, #4402, #12623 ),
 ( #490, #4065, #9440 ),
 ( #16075, #21468, #383 ),
 ( #19644, #7600, #11376 ),
 ( #14342, #7377, #7826 ) ),
 .UNSPECIFIED., .F., .F., .F. ) 
 B_SPLINE_SURFACE_WITH_KNOTS ( ( 4, 2, 2, 4 ),
 ( 3, 3 ),
 ( 0.000000000000000000, 0.005619572794280895157, 0.008429359191421343170, 0.01123914558856179031 ),
 ( 0.000000000000000000, 1.000000000000000000 ),
 .UNSPECIFIED. ) 
 GEOMETRIC_REPRESENTATION_ITEM ( )  RATIONAL_B_SPLINE_SURFACE ( (
 ( 1.000000000000000000, 0.7200096751079887447, 1.000000000000000000),
 ( 1.000000000000000000, 0.7496815117894589653, 1.000000000000000000),
 ( 1.000000000000000000, 0.7737746244353003178, 1.000000000000000000),
 ( 1.000000000000000000, 0.8024243379858346792, 1.000000000000000000),
 ( 1.000000000000000000, 0.8107154503869030693, 1.000000000000000000),
 ( 1.000000000000000000, 0.8248921579236677681, 1.000000000000000000),
 ( 1.000000000000000000, 0.8307774003432533139, 1.000000000000000000),
 ( 1.000000000000000000, 0.8354972176269003237, 1.000000000000000000) ) ) 
 REPRESENTATION_ITEM ( '' )  SURFACE ( )  );
#6635=CARTESIAN_POINT ( 'NONE',  ( 23.49999999999998579, 19.99999999999999645, -105.0010000000000048 ) ) ;
#6637=CARTESIAN_POINT ( 'NONE',  ( -19.59396665412805305, 15.89499847339672556, -60.52448832957815483 ) ) ;
#6638=DIRECTION ( 'NONE',  ( 1.049727191138618326E-16, -0.5150380749100547106, 0.8571673007021120005 ) ) ;
#6639=CARTESIAN_POINT ( 'NONE',  ( -13.23602284716360700, 35.01773851406191085, 58.53880247431295203 ) ) ;
#6640=ORIENTED_EDGE ( 'NONE', *, *, #10054, .F. ) ;
#6641=DIRECTION ( 'NONE',  ( -0.000000000000000000, -1.000000000000000000, -0.000000000000000000 ) ) ;
#6646=DIRECTION ( 'NONE',  ( -0.000000000000000000, 1.000000000000000000, -0.000000000000000000 ) ) ;
#6648=DIRECTION ( 'NONE',  ( 0.000000000000000000, 1.000000000000000000, 0.000000000000000000 ) ) ;
#6657=B_SPLINE_CURVE_WITH_KNOTS ( 'NONE', 1,
 ( #9655, #15131 ),
 .UNSPECIFIED., .F., .F.,
 ( 2, 2 ),
 ( 0.000000000000000000, 1.000000000000000000 ),
 .UNSPECIFIED. ) ;
#6658=CARTESIAN_POINT ( 'NONE',  ( 2.066061548968385786, -1.174227811083158768, 49.70141618117709470 ) ) ;
#6659=CARTESIAN_POINT ( 'NONE',  ( -1.387778780781445676E-14, 20.00000000000000000, -101.0000000000000284 ) ) ;
#6660=CARTESIAN_POINT ( 'NONE',  ( 18.43548664438524298, 12.20444905678965242, 60.22785496272550887 ) ) ;
#6661=ADVANCED_FACE ( 'NONE', ( #8570 ), #13638, .T. ) ;
#6665=DIRECTION ( 'NONE',  ( -0.000000000000000000, -0.000000000000000000, -1.000000000000000000 ) ) ;
#6667=DIRECTION ( 'NONE',  ( -0.000000000000000000, -0.000000000000000000, -1.000000000000000000 ) ) ;
#6670=CARTESIAN_POINT ( 'NONE',  ( -34.99999999999999289, -4.999999999999997335, -57.00000000000000711 ) ) ;
#6673=CARTESIAN_POINT ( 'NONE',  ( -9.226606582130424172, 39.40757736410211720, -54.37932754532841528 ) ) ;
#6674=EDGE_LOOP ( 'NONE', ( #20435, #703, #3739, #12573 ) ) ;
#6677=CARTESIAN_POINT ( 'NONE',  ( -19.46387463785194072, 8.808008015900622212, 57.95411844647836830 ) ) ;
#6680=LINE ( 'NONE', #10322, #19227 ) ;
#6681=DIRECTION ( 'NONE',  ( 1.000000000000000000, 0.000000000000000000, 0.000000000000000000 ) ) ;
#6683=DIRECTION ( 'NONE',  ( -1.000000000000000000, 0.000000000000000000, 0.000000000000000000 ) ) ;
#6688=ORIENTED_EDGE ( 'NONE', *, *, #1305, .F. ) ;
#6689=EDGE_CURVE ( 'NONE', #15831, #575, #14779, .T. ) ;
#6691=CIRCLE ( 'NONE', #22075, 2.099999999999990763 ) ;
#6694=CARTESIAN_POINT ( 'NONE',  ( 22.42346072916785360, 20.15694599340440973, 58.66711769948891231 ) ) ;
#6702=DIRECTION ( 'NONE',  ( 0.000000000000000000, 0.000000000000000000, -1.000000000000000000 ) ) ;
#6704=CARTESIAN_POINT ( 'NONE',  ( -1.095796999069928335, 39.99285418986146823, 49.56761373141846860 ) ) ;
#6708=EDGE_CURVE ( 'NONE', #121, #3042, #16237, .T. ) ;
#6709=CARTESIAN_POINT ( 'NONE',  ( -11.37797799463864479, 10.21854205506532942, 44.06891764425671454 ) ) ;
#6712=EDGE_CURVE ( 'NONE', #6550, #13970, #7413, .T. ) ;
#6713=ORIENTED_EDGE ( 'NONE', *, *, #4056, .T. ) ;
#6714=ORIENTED_EDGE ( 'NONE', *, *, #8177, .F. ) ;
#6718=CONICAL_SURFACE ( 'NONE', #7071, 57.00000000000002132, 0.7853981633974437271 ) ;
#6719=CARTESIAN_POINT ( 'NONE',  ( -10.72803533575910606, 39.99999999999999289, -53.87712872072328452 ) ) ;
#6721=CARTESIAN_POINT ( 'NONE',  ( 6.718896861934306131, 39.70714866090484918, 53.19564681394206218 ) ) ;
#6724=VERTEX_POINT ( 'NONE', #14386 ) ;
#6726=CARTESIAN_POINT ( 'NONE',  ( -8.910373547852051601, 39.99999999999999289, -53.30647736630695732 ) ) ;
#6728=CARTESIAN_POINT ( 'NONE',  ( 42.50000000000000711, -12.00000000000000000, -54.00000000000000000 ) ) ;
#6729=( LENGTH_UNIT ( ) NAMED_UNIT ( * ) SI_UNIT ( .MILLI., .METRE. ) );
#6733=DIRECTION ( 'NONE',  ( 0.000000000000000000, 0.000000000000000000, -1.000000000000000000 ) ) ;
#6737=CARTESIAN_POINT ( 'NONE',  ( -6.699391982050367567, -4.821764332415702903, -49.69317737456919559 ) ) ;
#6738=FACE_BOUND ( 'NONE', #437, .T. ) ;
#6740=ORIENTED_EDGE ( 'NONE', *, *, #3180, .F. ) ;
#6742=CARTESIAN_POINT ( 'NONE',  ( -2.085528189144346900, -1.173081074622058351, 49.71451653583131503 ) ) ;
#6747=CARTESIAN_POINT ( 'NONE',  ( 14.76055860720887658, 17.30233064284066558, 45.72055682016589628 ) ) ;
#6752=CARTESIAN_POINT ( 'NONE',  ( -19.87880993181333267, 17.63198765388839462, -60.59324977527813871 ) ) ;
#6753=CIRCLE ( 'NONE', #16626, 2.499999999999995115 ) ;
#6754=CARTESIAN_POINT ( 'NONE',  ( -2.081668171172227205E-14, 40.00000000000002132, 48.73397172404484223 ) ) ;
#6756=CARTESIAN_POINT ( 'NONE',  ( -15.40035801025640616, 32.79675990107260475, 56.74176776513680664 ) ) ;
#6758=CARTESIAN_POINT ( 'NONE',  ( 12.06668108811419238, 28.91809087000032363, 44.43106897542664058 ) ) ;
#6761=DIRECTION ( 'NONE',  ( -0.000000000000000000, 1.000000000000000000, -0.000000000000000000 ) ) ;
#6762=ORIENTED_EDGE ( 'NONE', *, *, #6366, .T. ) ;
#6764=DIRECTION ( 'NONE',  ( -0.000000000000000000, 1.000000000000000000, -0.000000000000000000 ) ) ;
#6765=B_SPLINE_CURVE_WITH_KNOTS ( 'NONE', 3,
 ( #16096, #404, #7513, #5796, #21958, #21843 ),
 .UNSPECIFIED., .F., .F.,
 ( 4, 2, 4 ),
 ( 0.000000000000000000, 0.002641318319679887301, 0.005282636639359774601 ),
 .UNSPECIFIED. ) ;
#6766=AXIS2_PLACEMENT_3D ( 'NONE', #17264, #10495, #13927 ) ;
#6772=DIRECTION ( 'NONE',  ( 8.659560562354932858E-17, 0.7071067811865474617, -0.7071067811865474617 ) ) ;
#6774=AXIS2_PLACEMENT_3D ( 'NONE', #8362, #3210, #17170 ) ;
#6775=DIRECTION ( 'NONE',  ( 0.000000000000000000, 0.000000000000000000, 1.000000000000000000 ) ) ;
#6782=CARTESIAN_POINT ( 'NONE',  ( -1.387778780781445676E-14, 20.00000000000000000, 98.00000000000000000 ) ) ;
#6783=AXIS2_PLACEMENT_3D ( 'NONE', #11965, #11847, #3275 ) ;
#6787=ORIENTED_EDGE ( 'NONE', *, *, #20750, .T. ) ;
#6788=LINE ( 'NONE', #20326, #17431 ) ;
#6789=CARTESIAN_POINT ( 'NONE',  ( 1.045712755958760010, 0.02735658877310587211, -49.70560592369783848 ) ) ;
#6794=AXIS2_PLACEMENT_3D ( 'NONE', #18113, #9299, #20071 ) ;
#6799=EDGE_LOOP ( 'NONE', ( #21845, #22689, #12168, #8121 ) ) ;
#6803=DIRECTION ( 'NONE',  ( 0.000000000000000000, -1.000000000000000000, 0.000000000000000000 ) ) ;
#6806=EDGE_CURVE ( 'NONE', #21191, #11348, #7845, .T. ) ;
#6808=CARTESIAN_POINT ( 'NONE',  ( -13.00000000000011546, 42.51666049839536043, -105.0000000000000142 ) ) ;
#6809=CARTESIAN_POINT ( 'NONE',  ( 12.23364788621108090, 38.77571842908469080, 55.51446324382119002 ) ) ;
#6810=CARTESIAN_POINT ( 'NONE',  ( -35.00000000000000000, 40.00000000000000000, 1.387778780781445676E-14 ) ) ;
#6812=FACE_OUTER_BOUND ( 'NONE', #12019, .T. ) ;
#6813=CARTESIAN_POINT ( 'NONE',  ( -5.422702462874739560, 6.007396227957873869, 40.31673423471877271 ) ) ;
#6819=CARTESIAN_POINT ( 'NONE',  ( -3.578893495154609069E-15, -4.765964690024343753, -45.28512947536507482 ) ) ;
#6821=CARTESIAN_POINT ( 'NONE',  ( 7.555723902514645651, 38.52224445567463817, -55.93227658743223429 ) ) ;
#6822=ADVANCED_FACE ( 'NONE', ( #20024 ), #9679, .T. ) ;
#6823=DIRECTION ( 'NONE',  ( -0.000000000000000000, 1.000000000000000000, -0.000000000000000000 ) ) ;
#6826=CIRCLE ( 'NONE', #2050, 4.000000000000000000 ) ;
#6830=AXIS2_PLACEMENT_3D ( 'NONE', #21065, #9144, #543 ) ;
#6831=AXIS2_PLACEMENT_3D ( 'NONE', #4851, #3248, #11821 ) ;
#6835=VERTEX_POINT ( 'NONE', #16808 ) ;
#6838=AXIS2_PLACEMENT_3D ( 'NONE', #14614, #5919, #2490 ) ;
#6839=CARTESIAN_POINT ( 'NONE',  ( -1.387778780781445518E-14, 20.00000000000000355, -102.0000000000000142 ) ) ;
#6840=LINE ( 'NONE', #10366, #10899 ) ;
#6841=CARTESIAN_POINT ( 'NONE',  ( 4.435586171696086488, 39.87782507471364823, 51.86130716576708011 ) ) ;
#6846=CARTESIAN_POINT ( 'NONE',  ( -0.3946983151935553602, 40.00000000000000000, -48.99018270876789671 ) ) ;
#6853=CARTESIAN_POINT ( 'NONE',  ( -19.29031483250425438, 25.30268833713983412, 60.44930483060160498 ) ) ;
#6855=ORIENTED_EDGE ( 'NONE', *, *, #12170, .F. ) ;
#6862=ORIENTED_EDGE ( 'NONE', *, *, #22039, .F. ) ;
#6863=CARTESIAN_POINT ( 'NONE',  ( 5.079212789377870685, -3.097595057472858127, -50.74825967503618784 ) ) ;
#6868=CARTESIAN_POINT ( 'NONE',  ( 5.011587927596622194, 34.16614174687214955, -40.02147800532275568 ) ) ;
#6870=CARTESIAN_POINT ( 'NONE',  ( -19.97049456717394378, 21.17381189076418124, -60.61481192459387302 ) ) ;
#6873=ORIENTED_EDGE ( 'NONE', *, *, #7442, .F. ) ;
#6876=CARTESIAN_POINT ( 'NONE',  ( -90.00000000000000000, 28.00000000000000000, -9.108981535246192915E-16 ) ) ;
#6877=PLANE ( 'NONE',  #10102 ) ;
#6878=CARTESIAN_POINT ( 'NONE',  ( 34.99999999999980815, 40.00000000000000000, 54.99999999999922551 ) ) ;
#6880=ORIENTED_EDGE ( 'NONE', *, *, #20667, .F. ) ;
#6886=ADVANCED_FACE ( 'NONE', ( #13228 ), #8437, .F. ) ;
#6889=CIRCLE ( 'NONE', #21894, 49.99999999999998579 ) ;
#6897=CARTESIAN_POINT ( 'NONE',  ( -7.505578006075205089, 1.461761173328240515, 55.63523492904089096 ) ) ;
#6904=CARTESIAN_POINT ( 'NONE',  ( 22.34927643452056145, 22.00360349561973194, -58.65118246389015155 ) ) ;
#6905=DIRECTION ( 'NONE',  ( -0.000000000000000000, -1.000000000000000000, -0.000000000000000000 ) ) ;
#6907=CARTESIAN_POINT ( 'NONE',  ( -4.196817137611960291, 39.89217750879657842, -51.71303688781891594 ) ) ;
#6909=AXIS2_PLACEMENT_3D ( 'NONE', #12215, #19100, #10485 ) ;
#6912=CARTESIAN_POINT ( 'NONE',  ( -12.59807286780803359, 38.55590838447053414, 55.66678043528293784 ) ) ;
#6914=DIRECTION ( 'NONE',  ( 1.000000000000000000, 0.000000000000000000, 0.000000000000000000 ) ) ;
#6916=DIRECTION ( 'NONE',  ( 8.659560562354932858E-17, 0.7071067811865474617, -0.7071067811865474617 ) ) ;
#6917=ADVANCED_FACE ( 'NONE', ( #22082 ), #19886, .F. ) ;
#6920=ORIENTED_EDGE ( 'NONE', *, *, #13041, .F. ) ;
#6922=EDGE_LOOP ( 'NONE', ( #4076, #10869, #17083, #18422 ) ) ;
#6924=ORIENTED_EDGE ( 'NONE', *, *, #21793, .T. ) ;
#6927=CARTESIAN_POINT ( 'NONE',  ( 18.83430946916724835, 32.25183488571027368, 57.78319592314319664 ) ) ;
#6928=CARTESIAN_POINT ( 'NONE',  ( 8.194251295035146043, 39.99999999999999289, -53.04030059599973157 ) ) ;
#6929=CARTESIAN_POINT ( 'NONE',  ( 2.321955323317326236, 40.00000000000000711, 50.16149361573952348 ) ) ;
#6932=CARTESIAN_POINT ( 'NONE',  ( -1.838758599476153277, 5.110847757086119714, 38.90097524723617539 ) ) ;
#6935=ORIENTED_EDGE ( 'NONE', *, *, #4880, .T. ) ;
#6937=CARTESIAN_POINT ( 'NONE',  ( 2.605854907981524526, 34.77417319504201032, 39.07589943342649974 ) ) ;
#6939=DIRECTION ( 'NONE',  ( 0.000000000000000000, 0.000000000000000000, 1.000000000000000000 ) ) ;
#6940=CARTESIAN_POINT ( 'NONE',  ( 35.00000000000000000, 2.142135623730931471, 4.258610482196280173E-15 ) ) ;
#6941=CARTESIAN_POINT ( 'NONE',  ( -2.217097371002125339, 39.97039923937872885, 50.37983947592398692 ) ) ;
#6942=CIRCLE ( 'NONE', #9503, 2.099999999999997868 ) ;
#6949=EDGE_CURVE ( 'NONE', #599, #21858, #12911, .T. ) ;
#6952=CARTESIAN_POINT ( 'NONE',  ( -14.30046708970334635, 2.690036953688593524, 56.32185947139072368 ) ) ;
#6953=CARTESIAN_POINT ( 'NONE',  ( -12.24744603030441148, 40.00000000000000000, 54.43639671998950291 ) ) ;
#6954=CIRCLE ( 'NONE', #1098, 2.099999999999997868 ) ;
#6958=CARTESIAN_POINT ( 'NONE',  ( 0.1259700001978051875, 39.99990731386942144, 48.83178812613451214 ) ) ;
#6962=CARTESIAN_POINT ( 'NONE',  ( -9.741231317622572661, 40.00000000000000711, -53.58312282093140055 ) ) ;
#6964=CARTESIAN_POINT ( 'NONE',  ( 11.49398617737438499, 39.99999999999999289, -54.13866599136454028 ) ) ;
#6970=DIRECTION ( 'NONE',  ( 0.000000000000000000, 1.000000000000000000, 0.000000000000000000 ) ) ;
#6971=CARTESIAN_POINT ( 'NONE',  ( -26.00000000000001421, 19.99999999999982947, 100.0000000000000000 ) ) ;
#6973=ORIENTED_EDGE ( 'NONE', *, *, #13379, .T. ) ;
#6976=DIRECTION ( 'NONE',  ( 0.000000000000000000, 0.000000000000000000, -1.000000000000000000 ) ) ;
#6979=CARTESIAN_POINT ( 'NONE',  ( 11.70544581405710893, 39.99999999999998579, -54.22116824785025813 ) ) ;
#6982=CARTESIAN_POINT ( 'NONE',  ( 4.108808078302957689, 34.46226780860838801, -39.55687577697710111 ) ) ;
#6984=CARTESIAN_POINT ( 'NONE',  ( -19.34774434964848666, 25.08511355156663569, -60.46357625386933421 ) ) ;
#6985=CARTESIAN_POINT ( 'NONE',  ( 42.50000000000000711, -5.000000000000000000, -49.60000000000000142 ) ) ;
#6990=DIRECTION ( 'NONE',  ( -0.8391477167891886468, 0.3845457931435830035, 0.3846500258456568289 ) ) ;
#6993=FACE_BOUND ( 'NONE', #2212, .T. ) ;
#6997=B_SPLINE_CURVE_WITH_KNOTS ( 'NONE', 3,
 ( #22651, #11632, #17007, #8199, #18972, #13327, #4659, #22308 ),
 .UNSPECIFIED., .F., .F.,
 ( 4, 2, 2, 4 ),
 ( 0.000000000000000000, 0.002219640113528450250, 0.003329460170292675592, 0.004439280227056901368 ),
 .UNSPECIFIED. ) ;
#6998=EDGE_CURVE ( 'NONE', #9194, #10478, #16399, .T. ) ;
#7000=DIRECTION ( 'NONE',  ( 0.000000000000000000, -0.000000000000000000, 1.000000000000000000 ) ) ;
#7001=CARTESIAN_POINT ( 'NONE',  ( 6.094635461684753786, 0.8905127700669610569, -54.73853566236119406 ) ) ;
#7004=ORIENTED_EDGE ( 'NONE', *, *, #22176, .F. ) ;
#7009=CARTESIAN_POINT ( 'NONE',  ( 21.63981290377902411, 13.82170478134235481, -58.49475859713702874 ) ) ;
#7011=CARTESIAN_POINT ( 'NONE',  ( 8.413264644294047301, 39.99999999999999289, 53.12447867214399366 ) ) ;
#7012=CARTESIAN_POINT ( 'NONE',  ( 13.75658951623322679, 25.99185038947793203, -45.26303799332215760 ) ) ;
#7015=CARTESIAN_POINT ( 'NONE',  ( -16.23964334364515594, 4.495128156857218116, 56.99255277661112018 ) ) ;
#7019=CARTESIAN_POINT ( 'NONE',  ( 35.00000000000058265, 40.00000000000000711, -57.52500000000076597 ) ) ;
#7020=VERTEX_POINT ( 'NONE', #12207 ) ;
#7025=FACE_OUTER_BOUND ( 'NONE', #5491, .T. ) ;
#7026=AXIS2_PLACEMENT_3D ( 'NONE', #5125, #17476, #3173 ) ;
#7027=CARTESIAN_POINT ( 'NONE',  ( 5.649796600896712206, 40.00000000000000711, -51.93142838570830122 ) ) ;
#7028=CARTESIAN_POINT ( 'NONE',  ( 9.741231313988977902, 39.99999999999997868, 53.58312281987703329 ) ) ;
#7029=EDGE_LOOP ( 'NONE', ( #18861, #4817, #10841, #2496 ) ) ;
#7030=DIRECTION ( 'NONE',  ( 0.000000000000000000, 1.000000000000000000, 0.000000000000000000 ) ) ;
#7036=CARTESIAN_POINT ( 'NONE',  ( -1.387778780781445676E-14, 20.00000000000000000, 102.0000000000000142 ) ) ;
#7041=EDGE_CURVE ( 'NONE', #3928, #1383, #19506, .T. ) ;
#7042=CARTESIAN_POINT ( 'NONE',  ( 22.42250004520295192, 20.31170080112650922, 58.66691407552199422 ) ) ;
#7048=EDGE_LOOP ( 'NONE', ( #13630, #22569, #12668, #13186 ) ) ;
#7052=DIRECTION ( 'NONE',  ( 1.000000000000000000, 0.000000000000000000, 0.000000000000000000 ) ) ;
#7055=CARTESIAN_POINT ( 'NONE',  ( 0.02110524776262648339, 39.99999746527640809, 48.75039555718117157 ) ) ;
#7059=CARTESIAN_POINT ( 'NONE',  ( -7.505578006075234399, 1.461761173328249175, -55.63523492904088386 ) ) ;
#7060=DIRECTION ( 'NONE',  ( -0.000000000000000000, -1.000000000000000000, -0.000000000000000000 ) ) ;
#7063=CARTESIAN_POINT ( 'NONE',  ( -17.68684951551754381, 29.34943212427064196, 60.02035230153434497 ) ) ;
#7064=CARTESIAN_POINT ( 'NONE',  ( -7.464643474138812351, 38.57205640809612390, 54.30629673035977589 ) ) ;
#7068=CIRCLE ( 'NONE', #12209, 58.99999999999994316 ) ;
#7069=EDGE_LOOP ( 'NONE', ( #16875, #6615, #11239 ) ) ;
#7071=AXIS2_PLACEMENT_3D ( 'NONE', #15682, #10182, #11905 ) ;
#7074=CARTESIAN_POINT ( 'NONE',  ( 5.748506628227421089, -0.6819283742231372347, -52.01451867725467793 ) ) ;
#7080=AXIS2_PLACEMENT_3D ( 'NONE', #13906, #21031, #1893 ) ;
#7081=CARTESIAN_POINT ( 'NONE',  ( -10.50000000000012079, 42.51666049839536043, -100.0000000000000000 ) ) ;
#7084=CARTESIAN_POINT ( 'NONE',  ( -15.00000000000001776, 20.77286304060558564, -45.82575694955838941 ) ) ;
#7088=CARTESIAN_POINT ( 'NONE',  ( 42.50000000000000711, -9.600000000000001421, 47.50000000000000711 ) ) ;
#7091=CARTESIAN_POINT ( 'NONE',  ( 25.99999999999998579, 19.99999999999999645, -105.0010000000000048 ) ) ;
#7093=CARTESIAN_POINT ( 'NONE',  ( 12.48541242016037955, 11.67824612544544394, -44.64471390988171606 ) ) ;
#7094=CONICAL_SURFACE ( 'NONE', #4546, 58.99999999999994316, 0.7853981633974725929 ) ;
#7097=DIRECTION ( 'NONE',  ( 0.4166911066143242914, 0.000000000000000000, 0.9090481404571101320 ) ) ;
#7101=ORIENTED_EDGE ( 'NONE', *, *, #9476, .F. ) ;
#7102=CYLINDRICAL_SURFACE ( 'NONE', #14930, 2.099999999999990763 ) ;
#7103=PLANE ( 'NONE',  #9527 ) ;
#7105=ORIENTED_EDGE ( 'NONE', *, *, #12780, .F. ) ;
#7107=CARTESIAN_POINT ( 'NONE',  ( -10.72803533576305846, 40.00000000000000711, 53.87712872072454928 ) ) ;
#7109=DIRECTION ( 'NONE',  ( -0.000000000000000000, 1.000000000000000000, -0.000000000000000000 ) ) ;
#7110=EDGE_CURVE ( 'NONE', #8965, #7701, #13999, .T. ) ;
#7113=DIRECTION ( 'NONE',  ( 0.000000000000000000, 0.000000000000000000, -1.000000000000000000 ) ) ;
#7115=CARTESIAN_POINT ( 'NONE',  ( -7.262748901058905027, 39.65386577537525170, -53.48190595416691195 ) ) ;
#7118=CIRCLE ( 'NONE', #16252, 15.99999999999998579 ) ;
#7119=CARTESIAN_POINT ( 'NONE',  ( -6.571663263633261032, 39.72078165228079882, -53.11617171249144320 ) ) ;
#7121=ORIENTED_EDGE ( 'NONE', *, *, #4648, .F. ) ;
#7122=EDGE_CURVE ( 'NONE', #20866, #6550, #17699, .T. ) ;
#7124=LINE ( 'NONE', #8402, #13267 ) ;
#7125=VERTEX_POINT ( 'NONE', #3637 ) ;
#7127=B_SPLINE_CURVE_WITH_KNOTS ( 'NONE', 3,
 ( #22515, #6809, #12400, #21012, #15610, #17222, #19410, #17447, #4976, #13653, #6927, #1535, #5102, #5314, #8519, #21121, #19182, #5422, #6694, #20672, #3375, #15494, #20903, #18957, #11957, #8754, #8631, #10335, #15722, #17334, #17563, #13886, #1872, #5204, #37, #12180, #3489, #8854 ),
 .UNSPECIFIED., .F., .F.,
 ( 4, 2, 2, 2, 2, 2, 2, 2, 2, 2, 2, 2, 2, 2, 2, 2, 2, 2, 4 ),
 ( 0.002265996298495700969, 0.003649092030476653800, 0.005032187762457607065, 0.007798379226419504054, 0.01056457069038139671, 0.01333076215434328936, 0.01609695361830517160, 0.01886314508226705558, 0.02439552801019081313, 0.02577862374217175512, 0.02716171947415269017, 0.02992791093811458455, 0.03131100667009553001, 0.03269410240207647200, 0.03546029386603836292, 0.03822648533000025384, 0.03960958106198120277, 0.04099267679396213782, 0.04652505972188593353 ),
 .UNSPECIFIED. ) ;
#7128=ORIENTED_EDGE ( 'NONE', *, *, #10883, .T. ) ;
#7129=EDGE_LOOP ( 'NONE', ( #6640, #791, #6451, #16449 ) ) ;
#7130=CARTESIAN_POINT ( 'NONE',  ( 35.00000000000000000, -5.000000000000000000, 4.258610482196280173E-15 ) ) ;
#7131=CIRCLE ( 'NONE', #5684, 57.07106781186551103 ) ;
#7135=CARTESIAN_POINT ( 'NONE',  ( 4.769735225253079136, 40.00000000000001421, 51.49386052712647199 ) ) ;
#7136=ORIENTED_EDGE ( 'NONE', *, *, #22522, .T. ) ;
#7137=DIRECTION ( 'NONE',  ( 0.000000000000000000, 0.000000000000000000, -1.000000000000000000 ) ) ;
#7138=CARTESIAN_POINT ( 'NONE',  ( -2.095812652544424282, 5.144891695986068214, 38.95253985045413714 ) ) ;
#7140=CYLINDRICAL_SURFACE ( 'NONE', #4054, 10.00000000000000178 ) ;
#7144=CARTESIAN_POINT ( 'NONE',  ( 3.604218085003671579, 34.56937985513295786, 39.39148225573723749 ) ) ;
#7145=ORIENTED_EDGE ( 'NONE', *, *, #5084, .T. ) ;
#7147=CARTESIAN_POINT ( 'NONE',  ( -4.577489642160328387, 39.86955245794722202, 51.95007345451820413 ) ) ;
#7149=CARTESIAN_POINT ( 'NONE',  ( 18.05287651232773527, 33.35671069585768578, 57.55759232970982708 ) ) ;
#7152=CARTESIAN_POINT ( 'NONE',  ( -1.387778780781445518E-14, 20.00000000000000355, -100.0000000000000000 ) ) ;
#7160=CARTESIAN_POINT ( 'NONE',  ( -13.52717286024091869, 5.231573370294034575, 56.05142967219525474 ) ) ;
#7166=CARTESIAN_POINT ( 'NONE',  ( 0.06748077356975319685, 39.99997318472687624, 48.78643326364329624 ) ) ;
#7170=FACE_OUTER_BOUND ( 'NONE', #7619, .T. ) ;
#7171=CARTESIAN_POINT ( 'NONE',  ( -12.99999999999980282, -2.516660498395516310, -100.0000000000000000 ) ) ;
#7174=EDGE_CURVE ( 'NONE', #1538, #10179, #17526, .T. ) ;
#7175=CARTESIAN_POINT ( 'NONE',  ( -14.64427171882024581, 33.62973864230776400, 59.05294378005811495 ) ) ;
#7180=CARTESIAN_POINT ( 'NONE',  ( -35.00000000000000000, 40.00000000000000000, 1.387778780781445676E-14 ) ) ;
#7182=DIRECTION ( 'NONE',  ( 1.000000000000000000, 0.000000000000000000, 0.000000000000000000 ) ) ;
#7185=CIRCLE ( 'NONE', #981, 18.00000000000000000 ) ;
#7186=ORIENTED_EDGE ( 'NONE', *, *, #21711, .T. ) ;
#7187=ORIENTED_EDGE ( 'NONE', *, *, #14848, .F. ) ;
#7189=CARTESIAN_POINT ( 'NONE',  ( 10.36558328700349563, 39.99999999999998579, -53.76404159467904265 ) ) ;
#7190=CIRCLE ( 'NONE', #13770, 57.00000000000002132 ) ;
#7194=CARTESIAN_POINT ( 'NONE',  ( -15.24242605747142143, 36.49796895611717673, -56.65858500684275612 ) ) ;
#7198=ORIENTED_EDGE ( 'NONE', *, *, #21648, .F. ) ;
#7200=FACE_BOUND ( 'NONE', #17456, .T. ) ;
#7202=DIRECTION ( 'NONE',  ( -1.000000000000000000, 0.000000000000000000, 0.000000000000000000 ) ) ;
#7208=EDGE_CURVE ( 'NONE', #21245, #22593, #18039, .T. ) ;
#7212=EDGE_CURVE ( 'NONE', #20078, #12474, #19151, .T. ) ;
#7214=ORIENTED_EDGE ( 'NONE', *, *, #17385, .T. ) ;
#7217=CARTESIAN_POINT ( 'NONE',  ( -12.82970538955583706, 1.687462484003148688, 55.75926248610267777 ) ) ;
#7221=EDGE_LOOP ( 'NONE', ( #19712, #6011, #11047, #17637, #6924, #20472, #10492, #150, #13907 ) ) ;
#7224=CARTESIAN_POINT ( 'NONE',  ( -8.923978417722670642, 2.083761144194947512, -56.51262908347766256 ) ) ;
#7227=AXIS2_PLACEMENT_3D ( 'NONE', #19570, #3880, #10613 ) ;
#7228=CARTESIAN_POINT ( 'NONE',  ( 22.27968669415837155, 17.44229586407517374, -58.63614535158252039 ) ) ;
#7229=CARTESIAN_POINT ( 'NONE',  ( -34.99999999999980815, 26.00000000000000355, 57.09999999999921982 ) ) ;
#7234=DIRECTION ( 'NONE',  ( -1.000000000000000000, 0.000000000000000000, 0.000000000000000000 ) ) ;
#7235=CARTESIAN_POINT ( 'NONE',  ( -4.435586534489145194, 39.87782505388838672, -51.86130739366951303 ) ) ;
#7239=DIRECTION ( 'NONE',  ( 0.000000000000000000, 0.5150380749100562650, 0.8571673007021111124 ) ) ;
#7245=EDGE_CURVE ( 'NONE', #9571, #10118, #11089, .T. ) ;
#7250=CARTESIAN_POINT ( 'NONE',  ( 14.99999999999998579, 20.00000000000000355, -101.0000000000000284 ) ) ;
#7252=CARTESIAN_POINT ( 'NONE',  ( 7.892682237755481722, 39.99999999999999289, 52.92195234101908596 ) ) ;
#7254=EDGE_CURVE ( 'NONE', #21483, #2902, #7068, .T. ) ;
#7255=ORIENTED_EDGE ( 'NONE', *, *, #213, .T. ) ;
#7257=CARTESIAN_POINT ( 'NONE',  ( 0.000000000000000000, 0.000000000000000000, 9.068199145005368464E-15 ) ) ;
#7260=CARTESIAN_POINT ( 'NONE',  ( -19.75454541434355349, 30.69619330606319707, -58.03277863335246423 ) ) ;
#7261=AXIS2_PLACEMENT_3D ( 'NONE', #21689, #10666, #5881 ) ;
#7262=VECTOR ( 'NONE', #2220, 1000.000000000000000 ) ;
#7264=ORIENTED_EDGE ( 'NONE', *, *, #11758, .T. ) ;
#7265=CARTESIAN_POINT ( 'NONE',  ( 7.505578006071305985, 1.461761173326673324, 55.63523492903841117 ) ) ;
#7268=CIRCLE ( 'NONE', #11123, 2.499999999999995115 ) ;
#7269=CARTESIAN_POINT ( 'NONE',  ( -34.99999999999999289, -4.928932188134504955, -57.07106781186550393 ) ) ;
#7274=CARTESIAN_POINT ( 'NONE',  ( 18.94034750358030550, 13.51583961449599336, 57.85890765540172964 ) ) ;
#7275=CARTESIAN_POINT ( 'NONE',  ( -90.00000000000000000, 28.00000000000000000, -9.108981535246192915E-16 ) ) ;
#7279=VERTEX_POINT ( 'NONE', #21840 ) ;
#7280=ADVANCED_FACE ( 'NONE', ( #3146 ), #3435, .F. ) ;
#7284=DIRECTION ( 'NONE',  ( 0.000000000000000000, -1.000000000000000000, 0.000000000000000000 ) ) ;
#7289=CARTESIAN_POINT ( 'NONE',  ( 2.229105169396924158, 39.97007249071501178, 50.38830863143780903 ) ) ;
#7292=FACE_OUTER_BOUND ( 'NONE', #1036, .T. ) ;
#7296=LINE ( 'NONE', #7402, #8625 ) ;
#7297=CARTESIAN_POINT ( 'NONE',  ( -35.00000000000058265, 28.00000000000000000, -52.50000000000076739 ) ) ;
#7300=CARTESIAN_POINT ( 'NONE',  ( 35.00000000000058265, 40.00000000000000711, -55.00000000000076028 ) ) ;
#7302=CARTESIAN_POINT ( 'NONE',  ( -42.50000000000000711, -12.00000000000000000, -49.60000000000000142 ) ) ;
#7303=CARTESIAN_POINT ( 'NONE',  ( -23.50000000000001066, 19.99999999999982947, -105.0000000000000142 ) ) ;
#7304=ORIENTED_EDGE ( 'NONE', *, *, #22658, .F. ) ;
#7306=CIRCLE ( 'NONE', #6578, 2.499999999999998668 ) ;
#7308=CARTESIAN_POINT ( 'NONE',  ( 8.306841137978913991, 0.005341471489716420606, -53.48947974212517664 ) ) ;
#7309=CARTESIAN_POINT ( 'NONE',  ( 13.00000000000024336, -2.516660498395250745, -105.0010000000000048 ) ) ;
#7312=CARTESIAN_POINT ( 'NONE',  ( -15.61498135782978558, 7.478867266539152681, 59.38575377909880615 ) ) ;
#7317=VERTEX_POINT ( 'NONE', #4763 ) ;
#7320=DIRECTION ( 'NONE',  ( 0.000000000000000000, 0.000000000000000000, 1.000000000000000000 ) ) ;
#7325=DIRECTION ( 'NONE',  ( 0.000000000000000000, 1.000000000000000000, 0.000000000000000000 ) ) ;
#7326=DIRECTION ( 'NONE',  ( 0.000000000000000000, -1.000000000000000000, 0.000000000000000000 ) ) ;
#7329=ORIENTED_EDGE ( 'NONE', *, *, #4728, .F. ) ;
#7330=EDGE_CURVE ( 'NONE', #5420, #1314, #20270, .T. ) ;
#7333=CARTESIAN_POINT ( 'NONE',  ( -9.103081159019540181, 0.03030367950604016467, 53.87333532811888404 ) ) ;
#7335=ORIENTED_EDGE ( 'NONE', *, *, #20962, .T. ) ;
#7337=CARTESIAN_POINT ( 'NONE',  ( -6.176809040140576634, 39.99999999999999289, 52.17714401493541487 ) ) ;
#7348=CARTESIAN_POINT ( 'NONE',  ( -0.3971970637539762872, 39.99908966794054521, -49.04071126575507833 ) ) ;
#7352=EDGE_CURVE ( 'NONE', #10435, #18025, #6585, .T. ) ;
#7357=ORIENTED_EDGE ( 'NONE', *, *, #11635, .T. ) ;
#7359=EDGE_LOOP ( 'NONE', ( #992, #22263, #13814, #15320 ) ) ;
#7365=CARTESIAN_POINT ( 'NONE',  ( 4.110274011050107923, 40.00000000000001421, 51.15360529889024832 ) ) ;
#7367=CARTESIAN_POINT ( 'NONE',  ( -35.00000000000058265, 28.00000000000000000, -57.10000000000076170 ) ) ;
#7371=EDGE_CURVE ( 'NONE', #12420, #16162, #861, .T. ) ;
#7373=CARTESIAN_POINT ( 'NONE',  ( -21.99996130922173876, 24.71724789032313296, -58.57718774367117476 ) ) ;
#7376=VERTEX_POINT ( 'NONE', #10565 ) ;
#7377=CARTESIAN_POINT ( 'NONE',  ( -0.2893420571180346235, -0.01224453477246113288, 48.63018218499173884 ) ) ;
#7378=ORIENTED_EDGE ( 'NONE', *, *, #5943, .T. ) ;
#7379=CARTESIAN_POINT ( 'NONE',  ( 4.278324951947162447, 39.54020021135892193, -53.33400390259981805 ) ) ;
#7381=EDGE_CURVE ( 'NONE', #18864, #19744, #15383, .T. ) ;
#7384=CARTESIAN_POINT ( 'NONE',  ( 19.87880993181303779, 17.63198765388676392, 60.59324977527815292 ) ) ;
#7386=DIRECTION ( 'NONE',  ( 0.000000000000000000, 0.000000000000000000, 1.000000000000000000 ) ) ;
#7389=VERTEX_POINT ( 'NONE', #3266 ) ;
#7390=ORIENTED_EDGE ( 'NONE', *, *, #4693, .F. ) ;
#7392=DIRECTION ( 'NONE',  ( 0.000000000000000000, 0.000000000000000000, -1.000000000000000000 ) ) ;
#7393=CARTESIAN_POINT ( 'NONE',  ( -10.80340688051430931, 39.17018323810926006, -54.94414022072520964 ) ) ;
#7396=CARTESIAN_POINT ( 'NONE',  ( -11.15511648635851039, 39.11609166919295433, -55.07420106208766697 ) ) ;
#7397=B_SPLINE_CURVE_WITH_KNOTS ( 'NONE', 3,
 ( #5215, #6819, #149, #19077 ),
 .UNSPECIFIED., .F., .F.,
 ( 4, 4 ),
 ( 0.004232217698034760993, 0.004798505571456043728 ),
 .UNSPECIFIED. ) ;
#7399=EDGE_LOOP ( 'NONE', ( #7667, #5902, #17929, #19657 ) ) ;
#7400=DIRECTION ( 'NONE',  ( -0.000000000000000000, 1.000000000000000000, -0.000000000000000000 ) ) ;
#7402=CARTESIAN_POINT ( 'NONE',  ( -5.833333333333339255, 40.00000000000000000, -40.61164310337066041 ) ) ;
#7403=CARTESIAN_POINT ( 'NONE',  ( -20.00000000000001421, 20.00000000000000000, -60.62177826491068799 ) ) ;
#7408=EDGE_CURVE ( 'NONE', #17743, #12228, #7127, .T. ) ;
#7409=CARTESIAN_POINT ( 'NONE',  ( 35.00000000000058265, 40.00000000000000711, -52.47500000000076170 ) ) ;
#7413=LINE ( 'NONE', #3878, #12567 ) ;
#7417=ADVANCED_FACE ( 'NONE', ( #7025 ), #12293, .F. ) ;
#7423=DIRECTION ( 'NONE',  ( -0.000000000000000000, 1.000000000000000000, -0.000000000000000000 ) ) ;
#7429=DIRECTION ( 'NONE',  ( 0.000000000000000000, -0.000000000000000000, -1.000000000000000000 ) ) ;
#7430=VERTEX_POINT ( 'NONE', #6050 ) ;
#7431=AXIS2_PLACEMENT_3D ( 'NONE', #16913, #14954, #3055 ) ;
#7432=DIRECTION ( 'NONE',  ( -0.000000000000000000, -1.000000000000000000, -0.000000000000000000 ) ) ;
#7435=CARTESIAN_POINT ( 'NONE',  ( 16.98435752851229452, 5.286895767878529995, -57.23469700293635753 ) ) ;
#7436=ORIENTED_EDGE ( 'NONE', *, *, #12082, .T. ) ;
#7440=CONICAL_SURFACE ( 'NONE', #20998, 57.00000000000002132, 0.7853981633974437271 ) ;
#7441=EDGE_LOOP ( 'NONE', ( #8624, #6920, #14098, #850 ) ) ;
#7442=EDGE_CURVE ( 'NONE', #6097, #6464, #11431, .T. ) ;
#7445=CARTESIAN_POINT ( 'NONE',  ( 35.00000000000000000, -9.000000000000001776, 4.258610482196280173E-15 ) ) ;
#7446=ORIENTED_EDGE ( 'NONE', *, *, #14657, .T. ) ;
#7448=CONICAL_SURFACE ( 'NONE', #22464, 2.099999999999997868, 1.029744258676653867 ) ;
#7449=CARTESIAN_POINT ( 'NONE',  ( -9.103081159019568602, 0.03030367950605284896, -53.87333532811888404 ) ) ;
#7450=ORIENTED_EDGE ( 'NONE', *, *, #4016, .T. ) ;
#7453=CIRCLE ( 'NONE', #11113, 22.00000000000000000 ) ;
#7454=CARTESIAN_POINT ( 'NONE',  ( 14.99999999999998579, 20.00000000000000355, -45.82575694955836809 ) ) ;
#7456=ORIENTED_EDGE ( 'NONE', *, *, #5673, .F. ) ;
#7457=CARTESIAN_POINT ( 'NONE',  ( -35.00000000000000000, -5.000000000000000000, 1.387778780781445676E-14 ) ) ;
#7458=CARTESIAN_POINT ( 'NONE',  ( 35.00000000000058265, 39.97500000000000142, -55.00000000000076028 ) ) ;
#7459=CARTESIAN_POINT ( 'NONE',  ( -6.687085228319380015, 39.71011799691164867, -53.17853451012708632 ) ) ;
#7467=EDGE_CURVE ( 'NONE', #3688, #18025, #19900, .T. ) ;
#7477=DIRECTION ( 'NONE',  ( 0.000000000000000000, 0.000000000000000000, -1.000000000000000000 ) ) ;
#7478=AXIS2_PLACEMENT_3D ( 'NONE', #5598, #6333, #18821 ) ;
#7480=CYLINDRICAL_SURFACE ( 'NONE', #8751, 30.00000000000000000 ) ;
#7482=VERTEX_POINT ( 'NONE', #4455 ) ;
#7483=CARTESIAN_POINT ( 'NONE',  ( 1.045507549828128990, 0.02734584580075648946, 49.70576511417586829 ) ) ;
#7484=FACE_OUTER_BOUND ( 'NONE', #9650, .T. ) ;
#7485=CARTESIAN_POINT ( 'NONE',  ( -15.00000000000001421, 20.00000000000000000, 60.00200000000000244 ) ) ;
#7487=CARTESIAN_POINT ( 'NONE',  ( -1.387778780781445676E-14, 20.00000000000000000, 98.00000000000000000 ) ) ;
#7489=CARTESIAN_POINT ( 'NONE',  ( 1.268121568163980362, 39.97056933375353793, -50.22305475356783688 ) ) ;
#7493=FACE_OUTER_BOUND ( 'NONE', #20752, .T. ) ;
#7495=CARTESIAN_POINT ( 'NONE',  ( 9.038718750511064215, 40.00000000000000000, -53.35171082564918521 ) ) ;
#7496=ADVANCED_FACE ( 'NONE', ( #4569 ), #17687, .F. ) ;
#7497=CARTESIAN_POINT ( 'NONE',  ( 22.35494499951315106, 21.77768233190464287, 58.65240855008568843 ) ) ;
#7499=CARTESIAN_POINT ( 'NONE',  ( 8.331955809010596070, 38.18181818181818699, -56.36098470834070895 ) ) ;
#7501=EDGE_CURVE ( 'NONE', #9389, #249, #15113, .T. ) ;
#7505=VERTEX_POINT ( 'NONE', #14633 ) ;
#7510=DIRECTION ( 'NONE',  ( -0.000000000000000000, 1.000000000000000000, -0.000000000000000000 ) ) ;
#7513=CARTESIAN_POINT ( 'NONE',  ( 8.916870955512969488, 2.080241304160146854, 56.50845996868202548 ) ) ;
#7516=VECTOR ( 'NONE', #18330, 1000.000000000000000 ) ;
#7519=CARTESIAN_POINT ( 'NONE',  ( -35.00000000000058265, 40.00000000000000000, -55.00000000000076028 ) ) ;
#7521=CARTESIAN_POINT ( 'NONE',  ( -10.30713387248692037, 2.842164160680663798, -57.27491564205611496 ) ) ;
#7522=AXIS2_PLACEMENT_3D ( 'NONE', #17310, #3356, #5295 ) ;
#7523=DIRECTION ( 'NONE',  ( 0.000000000000000000, -1.000000000000000000, 0.000000000000000000 ) ) ;
#7524=DIRECTION ( 'NONE',  ( 0.000000000000000000, -0.7071067811867928210, -0.7071067811863022134 ) ) ;
#7525=DIRECTION ( 'NONE',  ( -0.000000000000000000, 1.000000000000000000, -0.000000000000000000 ) ) ;
#7528=ORIENTED_EDGE ( 'NONE', *, *, #12040, .T. ) ;
#7534=EDGE_CURVE ( 'NONE', #15820, #21174, #15484, .T. ) ;
#7541=CARTESIAN_POINT ( 'NONE',  ( -8.331955809010628045, 38.18181818181818699, -56.36098470834071605 ) ) ;
#7545=CARTESIAN_POINT ( 'NONE',  ( -0.7810292038144046600, 39.98537128388858264, -49.65442669227651606 ) ) ;
#7547=CARTESIAN_POINT ( 'NONE',  ( 9.852267639826706613, 8.683574217357186598, -43.21671877549182739 ) ) ;
#7550=EDGE_LOOP ( 'NONE', ( #8836, #5298 ) ) ;
#7554=AXIS2_PLACEMENT_3D ( 'NONE', #12594, #10762, #15590 ) ;
#7555=DIRECTION ( 'NONE',  ( -0.000000000000000000, -0.000000000000000000, -1.000000000000000000 ) ) ;
#7556=DIRECTION ( 'NONE',  ( -0.000000000000000000, -1.000000000000000000, -0.000000000000000000 ) ) ;
#7561=DIRECTION ( 'NONE',  ( 0.000000000000000000, 0.7071067811865507924, 0.7071067811865441310 ) ) ;
#7562=ORIENTED_EDGE ( 'NONE', *, *, #17859, .F. ) ;
#7564=CARTESIAN_POINT ( 'NONE',  ( -8.640962819011734908, 40.00000000000000000, 53.20846273842203544 ) ) ;
#7566=DIRECTION ( 'NONE',  ( -0.000000000000000000, -0.000000000000000000, -1.000000000000000000 ) ) ;
#7572=DIRECTION ( 'NONE',  ( -0.4124789556921610312, -0.7071067811865332509, -0.5743353646704374427 ) ) ;
#7573=CARTESIAN_POINT ( 'NONE',  ( -0.2316815189680993536, 39.99968400692258541, -48.91347655445596132 ) ) ;
#7574=CIRCLE ( 'NONE', #241, 2.499999999999995115 ) ;
#7577=CARTESIAN_POINT ( 'NONE',  ( -7.033428926742895548, 33.31269054942711705, 41.47353357286039710 ) ) ;
#7578=CARTESIAN_POINT ( 'NONE',  ( 1.591932335265033587E-15, -4.923002280079127832E-27, 50.50395615645412306 ) ) ;
#7587=DIRECTION ( 'NONE',  ( 0.000000000000000000, 0.000000000000000000, 1.000000000000000000 ) ) ;
#7590=DIRECTION ( 'NONE',  ( 0.000000000000000000, 1.000000000000000000, 0.000000000000000000 ) ) ;
#7591=EDGE_CURVE ( 'NONE', #18864, #575, #2238, .T. ) ;
#7593=CARTESIAN_POINT ( 'NONE',  ( 12.24744603030438839, 40.00000000000000000, -54.43639671998947449 ) ) ;
#7600=CARTESIAN_POINT ( 'NONE',  ( 0.4211638912453626871, -0.02267170259972375174, 49.14966933622903156 ) ) ;
#7602=EDGE_LOOP ( 'NONE', ( #7121, #15782 ) ) ;
#7604=CONICAL_SURFACE ( 'NONE', #8693, 2.525000000000110489, 0.7853981633971014453 ) ;
#7607=EDGE_LOOP ( 'NONE', ( #4652, #5198, #2654, #714 ) ) ;
#7609=CIRCLE ( 'NONE', #6155, 2.499999999999998668 ) ;
#7616=EDGE_LOOP ( 'NONE', ( #1623, #20928, #495, #1635 ) ) ;
#7617=CONICAL_SURFACE ( 'NONE', #21887, 49.99999999999998579, 0.7853981633974691512 ) ;
#7619=EDGE_LOOP ( 'NONE', ( #17672, #12687, #15073, #21703 ) ) ;
#7620=DIRECTION ( 'NONE',  ( -0.000000000000000000, 1.000000000000000000, -0.000000000000000000 ) ) ;
#7625=EDGE_CURVE ( 'NONE', #21079, #15231, #13272, .T. ) ;
#7626=AXIS2_PLACEMENT_3D ( 'NONE', #3980, #9229, #21272 ) ;
#7628=CARTESIAN_POINT ( 'NONE',  ( -9.689843208404433028, 39.33333333333334991, -54.54983754392741702 ) ) ;
#7629=DIRECTION ( 'NONE',  ( -1.000000000000000000, 0.000000000000000000, 0.000000000000000000 ) ) ;
#7633=FACE_OUTER_BOUND ( 'NONE', #22221, .T. ) ;
#7637=DIRECTION ( 'NONE',  ( -1.000000000000000000, 0.000000000000000000, 0.000000000000000000 ) ) ;
#7638=DIRECTION ( 'NONE',  ( 0.000000000000000000, 0.000000000000000000, -1.000000000000000000 ) ) ;
#7645=VERTEX_POINT ( 'NONE', #5555 ) ;
#7647=EDGE_CURVE ( 'NONE', #8904, #15024, #9917, .T. ) ;
#7648=ORIENTED_EDGE ( 'NONE', *, *, #18549, .F. ) ;
#7650=EDGE_CURVE ( 'NONE', #15602, #22642, #19061, .T. ) ;
#7652=CYLINDRICAL_SURFACE ( 'NONE', #2116, 60.00000000000000000 ) ;
#7653=CARTESIAN_POINT ( 'NONE',  ( -0.05288783471925459501, -1.234056376215191486, -48.20419181041116019 ) ) ;
#7654=CARTESIAN_POINT ( 'NONE',  ( 1.007402651613724608E-12, -1.880345380268765651E-13, 50.27953280580743467 ) ) ;
#7655=CARTESIAN_POINT ( 'NONE',  ( -19.60425726290410964, 16.02072691545761174, 60.52684394361300235 ) ) ;
#7656=CARTESIAN_POINT ( 'NONE',  ( -1.510243460696181139E-14, 40.00000000000000000, -48.73397172404481381 ) ) ;
#7659=CYLINDRICAL_SURFACE ( 'NONE', #2084, 15.00000000000000000 ) ;
#7663=DIRECTION ( 'NONE',  ( 0.000000000000000000, 0.000000000000000000, 1.000000000000000000 ) ) ;
#7664=EDGE_CURVE ( 'NONE', #20382, #7125, #18331, .T. ) ;
#7667=ORIENTED_EDGE ( 'NONE', *, *, #7591, .F. ) ;
#7670=CARTESIAN_POINT ( 'NONE',  ( 35.00000000000058265, 40.00000000000000000, -52.50000000000076739 ) ) ;
#7674=EDGE_LOOP ( 'NONE', ( #18467, #8840 ) ) ;
#7675=FACE_OUTER_BOUND ( 'NONE', #3601, .T. ) ;
#7680=CARTESIAN_POINT ( 'NONE',  ( -12.84005703549979849, 1.693876179609747012, -55.76322220629404569 ) ) ;
#7683=CARTESIAN_POINT ( 'NONE',  ( 11.86180952234342278, 38.99999999999291589, -55.35904751185374550 ) ) ;
#7686=DIRECTION ( 'NONE',  ( 0.000000000000000000, 0.000000000000000000, -1.000000000000000000 ) ) ;
#7689=ADVANCED_FACE ( 'NONE', ( #5793, #12768 ), #19779, .F. ) ;
#7691=CARTESIAN_POINT ( 'NONE',  ( -34.99999999999980815, 28.00000000000000000, 57.09999999999921982 ) ) ;
#7693=CARTESIAN_POINT ( 'NONE',  ( -13.76792553423404186, 26.00189441538239876, 45.26963775109940968 ) ) ;
#7701=VERTEX_POINT ( 'NONE', #856 ) ;
#7706=LINE ( 'NONE', #9539, #10530 ) ;
#7712=CARTESIAN_POINT ( 'NONE',  ( -19.90501858586609174, 9.588439829449736607, -58.07150046051949488 ) ) ;
#7714=CARTESIAN_POINT ( 'NONE',  ( 15.61498135782973584, 7.478867266539133141, -59.38575377909876352 ) ) ;
#7716=CARTESIAN_POINT ( 'NONE',  ( -9.103081159019540181, 0.03030367950604016467, 53.87333532811888404 ) ) ;
#7718=ORIENTED_EDGE ( 'NONE', *, *, #19289, .F. ) ;
#7719=CARTESIAN_POINT ( 'NONE',  ( 5.617739682035653992, 39.81210785744588065, 52.56498351368300348 ) ) ;
#7721=ORIENTED_EDGE ( 'NONE', *, *, #4187, .F. ) ;
#7722=CARTESIAN_POINT ( 'NONE',  ( 16.99999999999997513, 20.00000000000000355, 102.0000000000000142 ) ) ;
#7723=CARTESIAN_POINT ( 'NONE',  ( 15.24242605747179802, 36.49796895611718384, 56.65858500684291243 ) ) ;
#7727=CARTESIAN_POINT ( 'NONE',  ( 11.24990497771462827, 36.62343892044964377, -57.74518096503230424 ) ) ;
#7728=ORIENTED_EDGE ( 'NONE', *, *, #12745, .T. ) ;
#7729=ORIENTED_EDGE ( 'NONE', *, *, #17140, .T. ) ;
#7731=EDGE_CURVE ( 'NONE', #11090, #18872, #20562, .T. ) ;
#7733=FACE_OUTER_BOUND ( 'NONE', #7359, .T. ) ;
#7740=EDGE_CURVE ( 'NONE', #10900, #3760, #4432, .T. ) ;
#7741=ADVANCED_BREP_SHAPE_REPRESENTATION ( '', ( #17721, #18273 ), #10192 ) ;
#7748=DIRECTION ( 'NONE',  ( -1.000000000000000000, 0.000000000000000000, 0.000000000000000000 ) ) ;
#7750=FACE_OUTER_BOUND ( 'NONE', #11665, .T. ) ;
#7760=CARTESIAN_POINT ( 'NONE',  ( 19.99999999999998579, 20.00000000000000711, -60.62177826491069510 ) ) ;
#7761=CARTESIAN_POINT ( 'NONE',  ( -6.869624750922561418, 39.72564401595366945, -53.24680511806212024 ) ) ;
#7763=CARTESIAN_POINT ( 'NONE',  ( 35.00000000000058265, 40.00000000000000711, -55.00000000000076028 ) ) ;
#7768=ORIENTED_EDGE ( 'NONE', *, *, #12181, .F. ) ;
#7770=EDGE_CURVE ( 'NONE', #1187, #2480, #15757, .T. ) ;
#7776=EDGE_CURVE ( 'NONE', #15580, #11720, #18697, .T. ) ;
#7778=VECTOR ( 'NONE', #14237, 1000.000000000000000 ) ;
#7779=ADVANCED_FACE ( 'NONE', ( #10116 ), #17336, .F. ) ;
#7781=CARTESIAN_POINT ( 'NONE',  ( 7.531932117834364782, 39.99999999999999289, -52.77310570466495676 ) ) ;
#7783=CARTESIAN_POINT ( 'NONE',  ( 2.669015549682804078, 39.95797184809391212, -50.69824233904017063 ) ) ;
#7785=ADVANCED_FACE ( 'NONE', ( #8414 ), #22636, .F. ) ;
#7788=CARTESIAN_POINT ( 'NONE',  ( 10.50000000000024514, -2.516660498395250745, -105.0000000000000142 ) ) ;
#7789=DIRECTION ( 'NONE',  ( 0.000000000000000000, 0.000000000000000000, -1.000000000000000000 ) ) ;
#7792=CYLINDRICAL_SURFACE ( 'NONE', #17635, 2.099999999999997868 ) ;
#7793=ORIENTED_EDGE ( 'NONE', *, *, #21182, .T. ) ;
#7794=DIRECTION ( 'NONE',  ( 0.000000000000000000, 0.000000000000000000, 1.000000000000000000 ) ) ;
#7796=DIRECTION ( 'NONE',  ( 0.000000000000000000, 0.000000000000000000, -1.000000000000000000 ) ) ;
#7799=DIRECTION ( 'NONE',  ( -0.8391477167891884248, 0.3845457931435832810, -0.3846500258456567733 ) ) ;
#7801=ORIENTED_EDGE ( 'NONE', *, *, #15860, .F. ) ;
#7804=AXIS2_PLACEMENT_3D ( 'NONE', #13604, #3096, #10066 ) ;
#7809=ORIENTED_EDGE ( 'NONE', *, *, #18522, .T. ) ;
#7810=CARTESIAN_POINT ( 'NONE',  ( 10.79056263833815343, 40.00000000000000711, 53.90082266129228117 ) ) ;
#7811=CARTESIAN_POINT ( 'NONE',  ( 5.961618526222387082, -3.061744126944893729, 51.29856354178728850 ) ) ;
#7814=CARTESIAN_POINT ( 'NONE',  ( -42.50000000000000711, -9.600000000000001421, 45.40000000000001279 ) ) ;
#7816=VERTEX_POINT ( 'NONE', #3267 ) ;
#7817=DIRECTION ( 'NONE',  ( 0.000000000000000000, 0.000000000000000000, -1.000000000000000000 ) ) ;
#7820=CARTESIAN_POINT ( 'NONE',  ( -15.00000000000001421, 20.00000000000000355, 101.0000000000000568 ) ) ;
#7821=CARTESIAN_POINT ( 'NONE',  ( -90.00000000000000000, 40.00000000000000000, -9.108981535246192915E-16 ) ) ;
#7823=DIRECTION ( 'NONE',  ( 1.000000000000000000, 0.000000000000000000, 0.000000000000000000 ) ) ;
#7826=CARTESIAN_POINT ( 'NONE',  ( -1.045703040280250073, 0.02735608008922960077, 49.70561346074470777 ) ) ;
#7827=ADVANCED_FACE ( 'NONE', ( #17565 ), #1592, .T. ) ;
#7828=ORIENTED_EDGE ( 'NONE', *, *, #1550, .F. ) ;
#7829=CARTESIAN_POINT ( 'NONE',  ( 1.427805587809481747, 39.96253296377607001, 50.08434700428703223 ) ) ;
#7830=CARTESIAN_POINT ( 'NONE',  ( -2.517789369293989221, 0.1458720723281411724, -52.33403986263111562 ) ) ;
#7832=VECTOR ( 'NONE', #2403, 1000.000000000000000 ) ;
#7833=CARTESIAN_POINT ( 'NONE',  ( 9.081037608041055975, 37.83854577724110868, 56.73868670301713024 ) ) ;
#7836=AXIS2_PLACEMENT_3D ( 'NONE', #3094, #1718, #22354 ) ;
#7837=CARTESIAN_POINT ( 'NONE',  ( -8.256135806682758371, -0.3920627093389252860, -55.63523492904088386 ) ) ;
#7841=CIRCLE ( 'NONE', #3473, 2.499999999999996891 ) ;
#7842=EDGE_LOOP ( 'NONE', ( #2150, #21603, #14880, #18396 ) ) ;
#7843=ORIENTED_EDGE ( 'NONE', *, *, #777, .F. ) ;
#7844=CARTESIAN_POINT ( 'NONE',  ( 9.689843208404433028, 39.33333333333334991, 54.54983754392749518 ) ) ;
#7845=CIRCLE ( 'NONE', #20655, 2.499999999999995115 ) ;
#7847=EDGE_LOOP ( 'NONE', ( #14655, #5971, #8418, #10855 ) ) ;
#7850=EDGE_LOOP ( 'NONE', ( #17060, #8517, #16089, #4134 ) ) ;
#7854=DIRECTION ( 'NONE',  ( -0.000000000000000000, -0.000000000000000000, -1.000000000000000000 ) ) ;
#7857=CLOSED_SHELL ( 'NONE', ( #8203, #6163, #966, #393, #6822, #15547, #12627, #10306, #7280, #20246, #15451, #14457, #19407, #8857, #17278, #15654, #12090, #12648, #4098, #6248, #9308, #1966, #18774, #22457, #11594, #19145, #8318, #15152, #5898, #13096, #17902, #17469, #2284, #11705, #1107, #4323, #15743, #13804, #11878, #19239, #1031, #19957, #14903, #1943, #1443, #15197, #5627, #15832, #20117, #6517, #12052, #14238, #16820, #14351, #9178, #19778, #62, #5091, #15380, #9307, #20319, #13835, #11915, #16938, #914, #1640, #3735, #21114, #2461, #21479, #11975, #1210, #11139, #1599, #21471, #16125, #1758, #10295, #10150, #7785, #11110, #9916, #2828, #13541, #2172, #21788, #8169, #7496, #15190, #20955, #11173, #6296, #4805, #1690, #19668, #16103, #21918, #7417, #208, #13353, #20112, #18655, #6386, #15286, #10791, #12940, #5031, #757, #18670, #20778, #14037, #8235, #11306, #20950, #17864, #1479, #15007, #22669, #1587, #19480, #3125, #14505, #3804, #879, #4721, #7989, #16919, #13493, #14830, #17435, #679, #2153, #8343, #3330, #6019, #12842, #16219, #134, #4240, #15605, #9965, #8673, #20013, #11292, #22297, #20295, #21871, #20108, #11752, #1532, #20069, #12732, #4141, #21377, #11851, #6423, #11315, #11179, #2251, #4911, #11428, #7689, #4021, #22351, #6917, #2325, #17181, #17097, #987, #20584, #10139, #16134, #18833, #10595, #4361, #2773, #15850, #13170, #14327, #14980, #6569, #26, #6886, #11236, #18196, #11087, #17714, #4813, #20967, #10673, #10582, #2999, #5559, #20297, #223, #21658, #7779, #4722, #21224, #21774, #18103, #18122, #4978, #5282, #6661, #6518, #12396, #4518, #20337, #9621, #776, #9572, #15793, #5541, #4601, #10931, #20489, #16174, #19268, #311, #6213, #1433, #8881, #10384, #20554, #5134, #14057, #15645, #12718, #12125, #71, #769, #7827, #15028, #12517, #8456, #13640, #17423, #5538, #2922, #2495, #1004, #391, #22563, #1572, #12437 ) ) ;
#7862=CARTESIAN_POINT ( 'NONE',  ( -1.265314100866710527E-14, 40.00000000000000000, 48.73397172404484223 ) ) ;
#7869=EDGE_LOOP ( 'NONE', ( #16019, #4656 ) ) ;
#7870=CARTESIAN_POINT ( 'NONE',  ( -19.48215071169293111, 15.15508441933061334, 58.00945324420519000 ) ) ;
#7874=CARTESIAN_POINT ( 'NONE',  ( 7.545596340824617165, -0.4932457138987723644, -52.99914579202174281 ) ) ;
#7888=CARTESIAN_POINT ( 'NONE',  ( 12.27586057105636108, 4.193657236093906171, 55.54740530680977884 ) ) ;
#7889=EDGE_CURVE ( 'NONE', #9501, #790, #14659, .T. ) ;
#7894=DIRECTION ( 'NONE',  ( 0.000000000000000000, 0.000000000000000000, 1.000000000000000000 ) ) ;
#7900=DIRECTION ( 'NONE',  ( 0.000000000000000000, 0.000000000000000000, 1.000000000000000000 ) ) ;
#7901=CARTESIAN_POINT ( 'NONE',  ( 5.004764015427562107, 40.00000000000000000, -51.61237785440702197 ) ) ;
#7905=CARTESIAN_POINT ( 'NONE',  ( 0.5471940025628014848, 39.99822778032481807, -49.15513688211015619 ) ) ;
#7906=CONICAL_SURFACE ( 'NONE', #13731, 8.999999999999973355, 0.7853981633974657095 ) ;
#7910=DIRECTION ( 'NONE',  ( 0.8171172023792294681, -0.3308262969263033870, -0.4720947350246249008 ) ) ;
#7911=CARTESIAN_POINT ( 'NONE',  ( -3.807409458091504995, 39.99999999999999289, 50.99570509775378468 ) ) ;
#7912=CARTESIAN_POINT ( 'NONE',  ( -42.50000000000000711, -11.97499999999999964, -47.50000000000000000 ) ) ;
#7913=CARTESIAN_POINT ( 'NONE',  ( 7.167333399831417102E-15, 39.99999999999997158, 48.73397172404483513 ) ) ;
#7917=DIRECTION ( 'NONE',  ( -0.000000000000000000, -1.000000000000000000, -0.000000000000000000 ) ) ;
#7920=CARTESIAN_POINT ( 'NONE',  ( 35.00000000000000000, -9.000000000000001776, 4.258610482196280173E-15 ) ) ;
#7922=CARTESIAN_POINT ( 'NONE',  ( -10.50000000000012079, 42.51666049839536043, 105.0000000000000142 ) ) ;
#7924=AXIS2_PLACEMENT_3D ( 'NONE', #20209, #4514, #11495 ) ;
#7926=VERTEX_POINT ( 'NONE', #4159 ) ;
#7932=CARTESIAN_POINT ( 'NONE',  ( 11.89435616776537508, 39.99999999999999289, 54.28884887643226165 ) ) ;
#7936=EDGE_CURVE ( 'NONE', #20516, #5386, #3339, .T. ) ;
#7937=LINE ( 'NONE', #6439, #12727 ) ;
#7941=ORIENTED_EDGE ( 'NONE', *, *, #11777, .T. ) ;
#7942=CARTESIAN_POINT ( 'NONE',  ( 35.00000000000058265, 28.00000000000000000, -55.00000000000076028 ) ) ;
#7944=DIRECTION ( 'NONE',  ( -0.000000000000000000, 1.000000000000000000, -0.000000000000000000 ) ) ;
#7945=CARTESIAN_POINT ( 'NONE',  ( 35.00000000000000000, 40.00000000000000000, 4.258610482196280173E-15 ) ) ;
#7947=CARTESIAN_POINT ( 'NONE',  ( -4.406386027442511732, 39.99999999999999289, -51.31001915654736933 ) ) ;
#7948=CARTESIAN_POINT ( 'NONE',  ( 1.255208329926582822, 39.96308463907303832, -50.19868133818717126 ) ) ;
#7949=ORIENTED_EDGE ( 'NONE', *, *, #10273, .T. ) ;
#7950=CARTESIAN_POINT ( 'NONE',  ( 2.576224933359583247, 39.84426458497860324, 51.65025110506229566 ) ) ;
#7951=CARTESIAN_POINT ( 'NONE',  ( -2.589893228699289285, 0.1394114517735031977, -50.61995827140722781 ) ) ;
#7952=AXIS2_PLACEMENT_3D ( 'NONE', #14340, #1881, #21130 ) ;
#7955=CARTESIAN_POINT ( 'NONE',  ( 12.72045107882486370, 38.45933137995365314, 55.71167848415526436 ) ) ;
#7958=EDGE_CURVE ( 'NONE', #9032, #3415, #9558, .T. ) ;
#7959=CARTESIAN_POINT ( 'NONE',  ( 21.29213537401512468, 12.67546417994482688, -58.41859095437539651 ) ) ;
#7965=EDGE_LOOP ( 'NONE', ( #485, #9414, #14427, #9420, #21581 ) ) ;
#7967=DIRECTION ( 'NONE',  ( -0.000000000000000000, -0.000000000000000000, -1.000000000000000000 ) ) ;
#7975=ORIENTED_EDGE ( 'NONE', *, *, #18288, .T. ) ;
#7976=CARTESIAN_POINT ( 'NONE',  ( -2.836563456948004695E-15, -1.236374842841498678, -48.24164917503444627 ) ) ;
#7979=AXIS2_PLACEMENT_3D ( 'NONE', #20500, #3082, #10051 ) ;
#7980=CARTESIAN_POINT ( 'NONE',  ( -8.331955809010631597, 38.18181818181817988, -56.36098470834072316 ) ) ;
#7983=AXIS2_PLACEMENT_3D ( 'NONE', #9297, #18112, #2426 ) ;
#7989=ADVANCED_FACE ( 'NONE', ( #16406 ), #16520, .F. ) ;
#7991=CIRCLE ( 'NONE', #1033, 30.00000000000000000 ) ;
#7993=CARTESIAN_POINT ( 'NONE',  ( -19.03045156298755103, 26.21228714462430176, 57.88457068412354545 ) ) ;
#7995=PLANE ( 'NONE',  #15643 ) ;
#8001=CARTESIAN_POINT ( 'NONE',  ( 1.255529093608926727, 39.96306425836120724, 50.19904361858062458 ) ) ;
#8002=CARTESIAN_POINT ( 'NONE',  ( 5.249999999999981348, 40.00000000000000000, 41.42387596543812123 ) ) ;
#8003=CARTESIAN_POINT ( 'NONE',  ( 10.27431133777207961, -4.928932188134511172, 51.43682631505490832 ) ) ;
#8006=EDGE_CURVE ( 'NONE', #12299, #1894, #4734, .T. ) ;
#8009=CARTESIAN_POINT ( 'NONE',  ( 35.00000000000000000, -9.000000000000001776, 4.258610482196280173E-15 ) ) ;
#8010=CARTESIAN_POINT ( 'NONE',  ( -9.689843208404443686, 39.33333333333332860, 54.54983754392751649 ) ) ;
#8019=DIRECTION ( 'NONE',  ( 0.000000000000000000, -0.7071067811867928210, -0.7071067811863022134 ) ) ;
#8020=CARTESIAN_POINT ( 'NONE',  ( 8.421835294225278545, 39.99999999999998579, -53.12761979129442125 ) ) ;
#8022=VERTEX_POINT ( 'NONE', #14787 ) ;
#8023=CARTESIAN_POINT ( 'NONE',  ( 15.50000000000024336, -2.516660498395250301, -100.0000000000000000 ) ) ;
#8026=CARTESIAN_POINT ( 'NONE',  ( -12.48541242016036357, 28.32175387455460935, -44.64471390988169475 ) ) ;
#8027=EDGE_CURVE ( 'NONE', #15231, #11262, #9873, .T. ) ;
#8033=CYLINDRICAL_SURFACE ( 'NONE', #5707, 2.499999999999996891 ) ;
#8036=CARTESIAN_POINT ( 'NONE',  ( 9.062586715441165452, 2.130694986412128511, 54.31128890270545639 ) ) ;
#8043=ORIENTED_EDGE ( 'NONE', *, *, #39, .T. ) ;
#8047=CARTESIAN_POINT ( 'NONE',  ( 18.52604901273056015, 27.59774142807036057, -60.25307787776290525 ) ) ;
#8048=CARTESIAN_POINT ( 'NONE',  ( 90.00000000000000000, 28.00000000000000000, -9.108981535246192915E-16 ) ) ;
#8051=CARTESIAN_POINT ( 'NONE',  ( 5.833333333333437842, 6.180730040185884455, -40.61164310337073857 ) ) ;
#8053=CARTESIAN_POINT ( 'NONE',  ( -42.50000000000000711, -12.00000000000012434, 47.50000000000000711 ) ) ;
#8061=CARTESIAN_POINT ( 'NONE',  ( 13.00000000000024336, -2.516660498395250745, 100.0000000000000000 ) ) ;
#8062=ORIENTED_EDGE ( 'NONE', *, *, #10016, .T. ) ;
#8063=CARTESIAN_POINT ( 'NONE',  ( -6.913287963588828688, 40.00000000000000711, -52.51234323549941507 ) ) ;
#8066=CARTESIAN_POINT ( 'NONE',  ( 8.619966100995542391, 38.06590016575250246, 54.65505662632602224 ) ) ;
#8067=CARTESIAN_POINT ( 'NONE',  ( -1.801805001521007421, 0.06845237652821531404, -51.82847917242283131 ) ) ;
#8072=FACE_OUTER_BOUND ( 'NONE', #10501, .T. ) ;
#8074=CARTESIAN_POINT ( 'NONE',  ( 22.43750227530513186, 20.33721733310946433, -58.67013217117666102 ) ) ;
#8077=CIRCLE ( 'NONE', #22358, 2.524999999999999467 ) ;
#8078=ORIENTED_EDGE ( 'NONE', *, *, #4129, .F. ) ;
#8083=CARTESIAN_POINT ( 'NONE',  ( 10.84015308351855111, 39.16451817967297444, 54.95776488309492436 ) ) ;
#8089=CARTESIAN_POINT ( 'NONE',  ( -35.00000000000000000, -5.000000000000000000, 57.00000000000003553 ) ) ;
#8091=CARTESIAN_POINT ( 'NONE',  ( 42.50000000000000711, -3.738192700042122674, -47.50000000000000000 ) ) ;
#8093=CARTESIAN_POINT ( 'NONE',  ( -9.103081159019573931, 0.03030367950605317509, -53.87333532811887693 ) ) ;
#8099=CARTESIAN_POINT ( 'NONE',  ( 90.00000000000000000, 40.00000000000000711, 2.524999999999998579 ) ) ;
#8100=EDGE_LOOP ( 'NONE', ( #14475, #1564, #7446, #10597, #15862 ) ) ;
#8103=CARTESIAN_POINT ( 'NONE',  ( -15.99370094303835899, 7.960486082690917620, 59.50964696497263873 ) ) ;
#8106=DIRECTION ( 'NONE',  ( 0.000000000000000000, 0.000000000000000000, 1.000000000000000000 ) ) ;
#8112=CARTESIAN_POINT ( 'NONE',  ( 5.302825731643186380, 39.28770244913255993, 54.25167596405761117 ) ) ;
#8113=CARTESIAN_POINT ( 'NONE',  ( -13.56354382738803999, 2.142135623730931471, -56.03997097393684612 ) ) ;
#8114=CARTESIAN_POINT ( 'NONE',  ( -4.278324951949648458, 39.54020021135842455, -53.33400390259981805 ) ) ;
#8115=CIRCLE ( 'NONE', #17979, 2.500000000000002220 ) ;
#8120=CARTESIAN_POINT ( 'NONE',  ( -15.50000000000011013, 42.51666049839536043, -105.0000000000000142 ) ) ;
#8121=ORIENTED_EDGE ( 'NONE', *, *, #7501, .T. ) ;
#8122=DIRECTION ( 'NONE',  ( 0.000000000000000000, 0.000000000000000000, -1.000000000000000000 ) ) ;
#8126=ORIENTED_EDGE ( 'NONE', *, *, #18779, .T. ) ;
#8127=CARTESIAN_POINT ( 'NONE',  ( -7.486329337576093756, -0.2507164912831579828, 53.02637754495041378 ) ) ;
#8130=DIRECTION ( 'NONE',  ( 0.000000000000000000, 0.000000000000000000, -1.000000000000000000 ) ) ;
#8134=CARTESIAN_POINT ( 'NONE',  ( -4.846083821622991117, 40.00000000000000711, 51.53252581920469311 ) ) ;
#8135=CARTESIAN_POINT ( 'NONE',  ( 11.86180952234342278, 38.99999999999291589, -55.35904751185374550 ) ) ;
#8136=CARTESIAN_POINT ( 'NONE',  ( 42.50000000000000711, -12.00000000000000000, 41.00000000000000711 ) ) ;
#8141=CARTESIAN_POINT ( 'NONE',  ( 9.744263423234823307, 2.495070046653235174, -54.63687069582775280 ) ) ;
#8144=AXIS2_PLACEMENT_3D ( 'NONE', #13800, #20819, #11864 ) ;
#8146=DIRECTION ( 'NONE',  ( 0.000000000000000000, 0.000000000000000000, -1.000000000000000000 ) ) ;
#8147=EDGE_CURVE ( 'NONE', #14794, #21010, #10966, .T. ) ;
#8149=EDGE_CURVE ( 'NONE', #12680, #2120, #17564, .T. ) ;
#8153=CARTESIAN_POINT ( 'NONE',  ( 10.15869103000891549, 39.99999999999999289, 53.70409622859173027 ) ) ;
#8154=DIRECTION ( 'NONE',  ( 0.9012767464701768594, -2.395770963567785064E-16, -0.4332438415859278247 ) ) ;
#8155=CARTESIAN_POINT ( 'NONE',  ( -1.387778780781445676E-14, 20.00000000000000000, 101.0000000000000568 ) ) ;
#8156=CARTESIAN_POINT ( 'NONE',  ( 19.80807096600698358, 16.80592363802972145, 60.57763526510201757 ) ) ;
#8162=CARTESIAN_POINT ( 'NONE',  ( -13.08927703801866649, 12.63446361230555581, -44.94509734929665967 ) ) ;
#8169=ADVANCED_FACE ( 'NONE', ( #18809 ), #3004, .F. ) ;
#8172=CARTESIAN_POINT ( 'NONE',  ( 0.05289805390978788435, -1.234055917683787085, -48.20418456595464107 ) ) ;
#8173=ORIENTED_EDGE ( 'NONE', *, *, #11678, .T. ) ;
#8177=EDGE_CURVE ( 'NONE', #13151, #14094, #14976, .T. ) ;
#8179=CARTESIAN_POINT ( 'NONE',  ( 19.98510692294565771, 21.15566478732735689, -58.14357129517338052 ) ) ;
#8180=CIRCLE ( 'NONE', #1218, 49.99999999999998579 ) ;
#8186=VECTOR ( 'NONE', #18167, 1000.000000000000000 ) ;
#8187=EDGE_LOOP ( 'NONE', ( #563, #4634, #11413, #16126 ) ) ;
#8196=CARTESIAN_POINT ( 'NONE',  ( 9.375626977035830478, 39.53999066946833096, -54.37753981121610281 ) ) ;
#8197=CIRCLE ( 'NONE', #10736, 2.099999999999990763 ) ;
#8198=FACE_OUTER_BOUND ( 'NONE', #3486, .T. ) ;
#8199=CARTESIAN_POINT ( 'NONE',  ( -9.038247590030331514E-14, -2.816400600653316655, -47.26426760038560104 ) ) ;
#8200=CARTESIAN_POINT ( 'NONE',  ( -0.04595184375223184542, 40.00000000000000711, 48.76974637106872024 ) ) ;
#8203=ADVANCED_FACE ( 'NONE', ( #22372 ), #2195, .F. ) ;
#8205=CARTESIAN_POINT ( 'NONE',  ( -13.75658951623323745, 14.00814961052206797, 45.26303799332217892 ) ) ;
#8207=CIRCLE ( 'NONE', #21021, 6.499999999999999112 ) ;
#8212=CARTESIAN_POINT ( 'NONE',  ( -18.85220035179115072, 32.22744690108881116, 57.78902400853742449 ) ) ;
#8213=CARTESIAN_POINT ( 'NONE',  ( -90.00000000000000000, 26.00000000000000355, -9.108981535246192915E-16 ) ) ;
#8215=CARTESIAN_POINT ( 'NONE',  ( -11.77933723464119531, 39.99999999999998579, 54.24924979334856090 ) ) ;
#8217=AXIS2_PLACEMENT_3D ( 'NONE', #13075, #11819, #15022 ) ;
#8219=CARTESIAN_POINT ( 'NONE',  ( -3.397749879293104236, 40.00000000000000711, -50.77335388622131518 ) ) ;
#8224=CARTESIAN_POINT ( 'NONE',  ( -10.71765026552324152, 39.18334136345070107, 54.91251049719502220 ) ) ;
#8227=CARTESIAN_POINT ( 'NONE',  ( 90.00000000000000000, 40.00000000000000711, -2.525000000000000355 ) ) ;
#8228=DIRECTION ( 'NONE',  ( 0.000000000000000000, 0.000000000000000000, -1.000000000000000000 ) ) ;
#8235=ADVANCED_FACE ( 'NONE', ( #21425, #2287 ), #7103, .T. ) ;
#8239=CARTESIAN_POINT ( 'NONE',  ( -2.601474714586578418, 34.77495088821684277, -39.07471001004991962 ) ) ;
#8242=CARTESIAN_POINT ( 'NONE',  ( -17.42297160866542427, 10.14068842408707560, -59.94615209474301309 ) ) ;
#8243=CARTESIAN_POINT ( 'NONE',  ( -1.486423889133612786, 39.99051292429980009, 49.86506860348632841 ) ) ;
#8245=DIRECTION ( 'NONE',  ( -0.000000000000000000, 1.000000000000000000, -0.000000000000000000 ) ) ;
#8250=VECTOR ( 'NONE', #19557, 1000.000000000000000 ) ;
#8251=EDGE_LOOP ( 'NONE', ( #15323, #3397, #17017, #17439 ) ) ;
#8255=CYLINDRICAL_SURFACE ( 'NONE', #14926, 60.00000000000000000 ) ;
#8259=CIRCLE ( 'NONE', #5693, 2.500000000000002220 ) ;
#8260=ORIENTED_EDGE ( 'NONE', *, *, #6689, .T. ) ;
#8262=ORIENTED_EDGE ( 'NONE', *, *, #17392, .F. ) ;
#8264=VECTOR ( 'NONE', #21537, 1000.000000000000000 ) ;
#8265=CARTESIAN_POINT ( 'NONE',  ( 8.306841138038604910, 0.005341471399264901936, 53.48947974206469524 ) ) ;
#8268=CARTESIAN_POINT ( 'NONE',  ( -1.387778780781445518E-14, 20.00000000000000355, 105.0000000000000142 ) ) ;
#8269=ORIENTED_EDGE ( 'NONE', *, *, #11404, .T. ) ;
#8271=CARTESIAN_POINT ( 'NONE',  ( -1.387778780781445676E-14, 20.00000000000000000, 100.0000000000000000 ) ) ;
#8272=ORIENTED_EDGE ( 'NONE', *, *, #8801, .T. ) ;
#8273=CARTESIAN_POINT ( 'NONE',  ( -15.00000000000001421, 20.00000000000000000, -45.82575694955838230 ) ) ;
#8275=DIRECTION ( 'NONE',  ( 0.000000000000000000, -0.000000000000000000, -1.000000000000000000 ) ) ;
#8276=LINE ( 'NONE', #18597, #13344 ) ;
#8277=CARTESIAN_POINT ( 'NONE',  ( 2.633052075911578527, 39.95897179782880926, 50.67294416386110356 ) ) ;
#8279=CARTESIAN_POINT ( 'NONE',  ( -6.490531301833351918, 40.00000000000000711, -52.32367560554533270 ) ) ;
#8283=CIRCLE ( 'NONE', #3901, 6.499999999999999112 ) ;
#8284=CARTESIAN_POINT ( 'NONE',  ( -2.836563456948004695E-15, -1.236374842841498678, -48.24164917503444627 ) ) ;
#8285=VECTOR ( 'NONE', #10647, 1000.000000000000000 ) ;
#8287=CARTESIAN_POINT ( 'NONE',  ( 35.00000000000000000, 40.00000000000000000, 4.258610482196280173E-15 ) ) ;
#8289=LINE ( 'NONE', #22390, #199 ) ;
#8292=CARTESIAN_POINT ( 'NONE',  ( 19.03045156299229745, 26.21228714462666787, -57.88457068413015350 ) ) ;
#8293=ORIENTED_EDGE ( 'NONE', *, *, #22450, .T. ) ;
#8298=ORIENTED_EDGE ( 'NONE', *, *, #12132, .F. ) ;
#8306=CIRCLE ( 'NONE', #5374, 6.499999999999999112 ) ;
#8308=CARTESIAN_POINT ( 'NONE',  ( 4.750176626998272589, 39.43750955791287538, -52.76318975003094636 ) ) ;
#8310=FACE_OUTER_BOUND ( 'NONE', #7847, .T. ) ;
#8311=CARTESIAN_POINT ( 'NONE',  ( 1.387778780781445676E-14, 40.00000000000000000, 48.73397172404482802 ) ) ;
#8313=VECTOR ( 'NONE', #15360, 1000.000000000000000 ) ;
#8317=ORIENTED_EDGE ( 'NONE', *, *, #6047, .F. ) ;
#8318=ADVANCED_FACE ( 'NONE', ( #4029 ), #10532, .F. ) ;
#8321=CARTESIAN_POINT ( 'NONE',  ( -19.96824854984944508, 18.58379861519951959, 58.13906733437337948 ) ) ;
#8324=AXIS2_PLACEMENT_3D ( 'NONE', #20033, #4339, #11318 ) ;
#8326=CARTESIAN_POINT ( 'NONE',  ( 8.230913578179089640, 39.55470086212452685, 53.98103023414088142 ) ) ;
#8328=CIRCLE ( 'NONE', #1018, 15.99999999999993072 ) ;
#8331=DIRECTION ( 'NONE',  ( -0.000000000000000000, 1.000000000000000000, -0.000000000000000000 ) ) ;
#8332=CARTESIAN_POINT ( 'NONE',  ( -4.643077448496365278, 40.00000000000000711, -51.42938343542150648 ) ) ;
#8336=EDGE_CURVE ( 'NONE', #938, #5289, #5494, .T. ) ;
#8340=CARTESIAN_POINT ( 'NONE',  ( -10.27431133777641215, -4.928932188134511172, -51.43682631505697600 ) ) ;
#8343=ADVANCED_FACE ( 'NONE', ( #1845 ), #108, .F. ) ;
#8345=ORIENTED_EDGE ( 'NONE', *, *, #5866, .T. ) ;
#8346=EDGE_CURVE ( 'NONE', #4117, #16727, #1816, .T. ) ;
#8347=EDGE_LOOP ( 'NONE', ( #14357, #1396 ) ) ;
#8348=CARTESIAN_POINT ( 'NONE',  ( -5.974741775054217996, -3.061019228945407455, 51.30674412914550686 ) ) ;
#8350=CARTESIAN_POINT ( 'NONE',  ( -42.50000000000000711, -12.00000000000012434, -47.50000000000000000 ) ) ;
#8356=CONICAL_SURFACE ( 'NONE', #4346, 58.99999999999994316, 0.7853981633974725929 ) ;
#8359=CARTESIAN_POINT ( 'NONE',  ( -17.58064943503768518, 10.42262370234541358, -57.45835854660190023 ) ) ;
#8360=AXIS2_PLACEMENT_3D ( 'NONE', #22259, #11925, #13518 ) ;
#8362=CARTESIAN_POINT ( 'NONE',  ( 25.99999999999998579, 19.99999999999999645, 100.0000000000000000 ) ) ;
#8363=CARTESIAN_POINT ( 'NONE',  ( -9.165377225651191395, 37.79989650906291132, 54.16098472236624417 ) ) ;
#8365=FACE_OUTER_BOUND ( 'NONE', #15202, .T. ) ;
#8366=FACE_BOUND ( 'NONE', #13680, .T. ) ;
#8367=CARTESIAN_POINT ( 'NONE',  ( 11.68090480754619875, 3.765577839755218648, -57.90797000640169045 ) ) ;
#8368=CARTESIAN_POINT ( 'NONE',  ( 9.165151389911684987, 40.00000000000000000, -56.36098470834078711 ) ) ;
#8375=EDGE_LOOP ( 'NONE', ( #8628, #21847, #1497, #11638 ) ) ;
#8379=DIRECTION ( 'NONE',  ( 0.000000000000000000, 0.000000000000000000, -1.000000000000000000 ) ) ;
#8383=CARTESIAN_POINT ( 'NONE',  ( 12.24744603029285273, 40.00000000000000000, 54.43639671998466412 ) ) ;
#8385=DIRECTION ( 'NONE',  ( -0.7071067811865561215, 0.000000000000000000, -0.7071067811865390240 ) ) ;
#8386=DIRECTION ( 'NONE',  ( -1.000000000000000000, 0.000000000000000000, 0.000000000000000000 ) ) ;
#8387=AXIS2_PLACEMENT_3D ( 'NONE', #604, #12503, #19516 ) ;
#8391=DIRECTION ( 'NONE',  ( 0.000000000000000000, -1.000000000000000000, 0.000000000000000000 ) ) ;
#8394=CARTESIAN_POINT ( 'NONE',  ( -0.7351298805842383377, 39.99998559474256865, -49.30628110933329822 ) ) ;
#8397=CARTESIAN_POINT ( 'NONE',  ( -14.95260096911754566, 3.243207204902324392, 56.55590526898573955 ) ) ;
#8399=CARTESIAN_POINT ( 'NONE',  ( -34.99999999999999289, 40.00000000000000000, 58.99999999999995737 ) ) ;
#8401=CARTESIAN_POINT ( 'NONE',  ( 35.00000000000058265, 40.00000000000000711, -52.47500000000076170 ) ) ;
#8402=CARTESIAN_POINT ( 'NONE',  ( 42.50000000000000711, -5.000000000000000000, 49.60000000000000853 ) ) ;
#8403=CARTESIAN_POINT ( 'NONE',  ( 17.96553007763552401, 11.19640018279076976, -57.57421575614285558 ) ) ;
#8414=FACE_OUTER_BOUND ( 'NONE', #596, .T. ) ;
#8415=ORIENTED_EDGE ( 'NONE', *, *, #19133, .T. ) ;
#8418=ORIENTED_EDGE ( 'NONE', *, *, #1897, .F. ) ;
#8419=CARTESIAN_POINT ( 'NONE',  ( 12.82970538955508566, 1.687462484002703267, 55.75926248610235803 ) ) ;
#8423=DIRECTION ( 'NONE',  ( 0.000000000000000000, 0.000000000000000000, 1.000000000000000000 ) ) ;
#8425=CARTESIAN_POINT ( 'NONE',  ( -8.492273200209872641, 39.51732067042856045, 54.09038547598553492 ) ) ;
#8426=FACE_OUTER_BOUND ( 'NONE', #10002, .T. ) ;
#8430=ORIENTED_EDGE ( 'NONE', *, *, #18143, .F. ) ;
#8435=CARTESIAN_POINT ( 'NONE',  ( -12.37316313323532491, 4.263667856436507364, 58.19925355777651532 ) ) ;
#8437=CYLINDRICAL_SURFACE ( 'NONE', #11806, 2.499999999999995115 ) ;
#8438=CARTESIAN_POINT ( 'NONE',  ( 2.243244216241373046, 39.96968658937159091, -50.39827808307496326 ) ) ;
#8440=CARTESIAN_POINT ( 'NONE',  ( 9.689843208404433028, 39.33333333333334991, 54.54983754392749518 ) ) ;
#8441=CIRCLE ( 'NONE', #13905, 2.499999999999998668 ) ;
#8445=CARTESIAN_POINT ( 'NONE',  ( -6.607276061855908544, 39.99999999999999289, -52.37472751582438946 ) ) ;
#8450=CARTESIAN_POINT ( 'NONE',  ( 42.50000000000000711, -9.600000000000001421, 47.50000000000000711 ) ) ;
#8454=CARTESIAN_POINT ( 'NONE',  ( -1.583519045122685265, -4.618580011808625763, -46.65783332780171833 ) ) ;
#8455=DIRECTION ( 'NONE',  ( -0.000000000000000000, -1.000000000000000000, -0.000000000000000000 ) ) ;
#8456=ADVANCED_FACE ( 'NONE', ( #7675 ), #10362, .T. ) ;
#8462=EDGE_LOOP ( 'NONE', ( #16718, #18801 ) ) ;
#8463=CARTESIAN_POINT ( 'NONE',  ( 11.84669267190939124, 10.76938159504117110, 44.31876460048056998 ) ) ;
#8465=CYLINDRICAL_SURFACE ( 'NONE', #1205, 2.500000000000002220 ) ;
#8466=DIRECTION ( 'NONE',  ( 0.000000000000000000, 0.000000000000000000, -1.000000000000000000 ) ) ;
#8467=CARTESIAN_POINT ( 'NONE',  ( -18.13678767553130200, 6.731837175185868105, -57.58481432322442117 ) ) ;
#8468=CARTESIAN_POINT ( 'NONE',  ( -3.803763136379629373, 39.91204990968978450, 51.45951558227579170 ) ) ;
#8469=CARTESIAN_POINT ( 'NONE',  ( -10.58465497539836342, 37.06540556999310354, 54.84139108225201653 ) ) ;
#8471=ORIENTED_EDGE ( 'NONE', *, *, #12725, .T. ) ;
#8472=CARTESIAN_POINT ( 'NONE',  ( 11.37797799463863768, 29.78145794493465104, 44.06891764425670743 ) ) ;
#8474=DIRECTION ( 'NONE',  ( -1.000000000000000000, 0.000000000000000000, 0.000000000000000000 ) ) ;
#8476=ORIENTED_EDGE ( 'NONE', *, *, #10524, .T. ) ;
#8482=ORIENTED_EDGE ( 'NONE', *, *, #7041, .T. ) ;
#8489=DIRECTION ( 'NONE',  ( -0.000000000000000000, -0.000000000000000000, -1.000000000000000000 ) ) ;
#8491=LINE ( 'NONE', #10309, #19354 ) ;
#8492=CARTESIAN_POINT ( 'NONE',  ( -12.24744603029287937, 40.00000000000000000, -54.43639671998464991 ) ) ;
#8494=CARTESIAN_POINT ( 'NONE',  ( 1.583519045122702806, -4.618580011808624874, -46.65783332780173964 ) ) ;
#8496=AXIS2_PLACEMENT_3D ( 'NONE', #3799, #9408, #21212 ) ;
#8497=CARTESIAN_POINT ( 'NONE',  ( -42.50000000000000711, -5.000000000000000000, 47.50000000000000711 ) ) ;
#8498=CARTESIAN_POINT ( 'NONE',  ( 6.217946977017707155, 39.75326280521958466, 52.92450750590739261 ) ) ;
#8499=ORIENTED_EDGE ( 'NONE', *, *, #3068, .F. ) ;
#8500=CARTESIAN_POINT ( 'NONE',  ( -1.485224345418334257, 39.99052334577585555, -49.86416394167165578 ) ) ;
#8504=CARTESIAN_POINT ( 'NONE',  ( -15.34956869069049823, 36.37910824616915306, 56.69201590313574712 ) ) ;
#8508=CARTESIAN_POINT ( 'NONE',  ( -42.50000000000000711, -5.000000000000000000, -47.50000000000000000 ) ) ;
#8509=VERTEX_POINT ( 'NONE', #11102 ) ;
#8517=ORIENTED_EDGE ( 'NONE', *, *, #12635, .F. ) ;
#8519=CARTESIAN_POINT ( 'NONE',  ( 21.21578383525635658, 27.34973130705544619, 58.39578210113617729 ) ) ;
#8520=CARTESIAN_POINT ( 'NONE',  ( -42.50000000000000711, -5.000000000000000000, 47.50000000000000711 ) ) ;
#8521=EDGE_CURVE ( 'NONE', #14798, #7317, #3965, .T. ) ;
#8524=DIRECTION ( 'NONE',  ( -0.000000000000000000, -0.000000000000000000, -1.000000000000000000 ) ) ;
#8526=DIRECTION ( 'NONE',  ( 1.000000000000000000, 0.000000000000000000, 0.000000000000000000 ) ) ;
#8530=DIRECTION ( 'NONE',  ( 0.000000000000000000, 0.000000000000000000, -1.000000000000000000 ) ) ;
#8541=ORIENTED_EDGE ( 'NONE', *, *, #18556, .T. ) ;
#8544=AXIS2_PLACEMENT_3D ( 'NONE', #13773, #17108, #3606 ) ;
#8547=DIRECTION ( 'NONE',  ( -0.000000000000000000, 1.000000000000000000, -0.000000000000000000 ) ) ;
#8548=CARTESIAN_POINT ( 'NONE',  ( 5.466611488789254736, 39.81233002189807024, 52.49274978756180587 ) ) ;
#8549=AXIS2_PLACEMENT_3D ( 'NONE', #5277, #15565, #13502 ) ;
#8550=ORIENTED_EDGE ( 'NONE', *, *, #15860, .T. ) ;
#8552=CARTESIAN_POINT ( 'NONE',  ( -2.175117848631995532, 40.00000000000000711, -50.07592579258850662 ) ) ;
#8554=CARTESIAN_POINT ( 'NONE',  ( 10.34137811700762555, 39.99999999999997868, -53.75702834151196896 ) ) ;
#8557=AXIS2_PLACEMENT_3D ( 'NONE', #7180, #14265, #5145 ) ;
#8560=CARTESIAN_POINT ( 'NONE',  ( -14.31751149541525336, 33.97259629115305302, 58.93694582298957840 ) ) ;
#8565=CYLINDRICAL_SURFACE ( 'NONE', #9337, 2.500000000000002220 ) ;
#8567=CARTESIAN_POINT ( 'NONE',  ( -2.109039589833474171, 34.88603667777789497, 38.90259428073981240 ) ) ;
#8568=VERTEX_POINT ( 'NONE', #15548 ) ;
#8570=FACE_OUTER_BOUND ( 'NONE', #894, .T. ) ;
#8572=CIRCLE ( 'NONE', #15880, 2.499999999999995115 ) ;
#8575=CARTESIAN_POINT ( 'NONE',  ( 14.99999999999998934, 19.22713695939442857, 45.82575694955839651 ) ) ;
#8576=CARTESIAN_POINT ( 'NONE',  ( 8.331955809010596070, 38.18181818181818699, -56.36098470834070895 ) ) ;
#8578=EDGE_CURVE ( 'NONE', #5921, #14950, #20144, .T. ) ;
#8579=CARTESIAN_POINT ( 'NONE',  ( -19.65511384563465569, 23.80142929986424960, -60.53962097676930654 ) ) ;
#8585=FACE_BOUND ( 'NONE', #6610, .T. ) ;
#8586=CARTESIAN_POINT ( 'NONE',  ( -30.00000000000001421, 20.00000000000000711, -100.0000000000000000 ) ) ;
#8595=DIRECTION ( 'NONE',  ( -0.000000000000000000, -0.000000000000000000, -1.000000000000000000 ) ) ;
#8601=ORIENTED_EDGE ( 'NONE', *, *, #5813, .T. ) ;
#8603=CARTESIAN_POINT ( 'NONE',  ( -10.06223851446539541, 39.28158160658948361, 54.67678195792279183 ) ) ;
#8606=CARTESIAN_POINT ( 'NONE',  ( 29.99999999999998579, 20.00000000000000355, -105.0000000000000142 ) ) ;
#8607=CARTESIAN_POINT ( 'NONE',  ( 20.10834676944517696, 10.02088872142240383, -58.12296025200761562 ) ) ;
#8608=AXIS2_PLACEMENT_3D ( 'NONE', #15047, #20349, #4655 ) ;
#8612=VERTEX_POINT ( 'NONE', #13592 ) ;
#8613=CARTESIAN_POINT ( 'NONE',  ( 42.50000000000000711, -3.738192700042122674, 47.50000000000000711 ) ) ;
#8615=ORIENTED_EDGE ( 'NONE', *, *, #9477, .F. ) ;
#8617=CARTESIAN_POINT ( 'NONE',  ( -30.00000000000001421, 20.00000000000000355, 105.0000000000000142 ) ) ;
#8621=FACE_BOUND ( 'NONE', #21554, .T. ) ;
#8624=ORIENTED_EDGE ( 'NONE', *, *, #14974, .F. ) ;
#8625=VECTOR ( 'NONE', #1910, 1000.000000000000000 ) ;
#8628=ORIENTED_EDGE ( 'NONE', *, *, #11532, .T. ) ;
#8631=CARTESIAN_POINT ( 'NONE',  ( 21.43973101033761708, 13.38729130222876762, 58.44776001661261233 ) ) ;
#8633=CARTESIAN_POINT ( 'NONE',  ( 8.265432197626479294, 40.00000000000000000, 53.06731919463958747 ) ) ;
#8636=CARTESIAN_POINT ( 'NONE',  ( 90.00000000000000000, 40.00000000000000711, -9.108981535246192915E-16 ) ) ;
#8638=AXIS2_PLACEMENT_3D ( 'NONE', #7821, #20201, #16759 ) ;
#8639=CARTESIAN_POINT ( 'NONE',  ( -6.000920103808232042, -0.8369757414283609531, 52.11565860623115753 ) ) ;
#8640=VECTOR ( 'NONE', #5912, 1000.000000000000000 ) ;
#8641=AXIS2_PLACEMENT_3D ( 'NONE', #6940, #19984, #2572 ) ;
#8645=CARTESIAN_POINT ( 'NONE',  ( 7.464640338966086475, 38.57205754384674634, -54.30630206323173326 ) ) ;
#8646=CARTESIAN_POINT ( 'NONE',  ( -1.814315892323006274, 39.98032163334644196, 50.09302599523660149 ) ) ;
#8650=CARTESIAN_POINT ( 'NONE',  ( 18.68837533793185912, 7.522086334128933238, 57.74247137455829915 ) ) ;
#8651=FACE_OUTER_BOUND ( 'NONE', #12505, .T. ) ;
#8652=DIRECTION ( 'NONE',  ( 0.000000000000000000, 0.000000000000000000, -1.000000000000000000 ) ) ;
#8654=AXIS2_PLACEMENT_3D ( 'NONE', #14511, #12347, #88 ) ;
#8656=ORIENTED_EDGE ( 'NONE', *, *, #22074, .F. ) ;
#8658=ORIENTED_EDGE ( 'NONE', *, *, #3893, .T. ) ;
#8661=CIRCLE ( 'NONE', #21846, 4.000000000000000000 ) ;
#8662=CARTESIAN_POINT ( 'NONE',  ( -13.00000000000011546, 42.51666049839536043, -100.0000000000000000 ) ) ;
#8663=FACE_OUTER_BOUND ( 'NONE', #14581, .T. ) ;
#8665=CARTESIAN_POINT ( 'NONE',  ( 2.239818980015277017, 39.96978032374031642, 50.39586354373248156 ) ) ;
#8666=B_SPLINE_CURVE_WITH_KNOTS ( 'NONE', 3,
 ( #5655, #11036, #12630, #18024, #2336, #387, #17808, #16304 ),
 .UNSPECIFIED., .F., .F.,
 ( 4, 2, 2, 4 ),
 ( 0.000000000000000000, 0.002330949112885988446, 0.004661898225771976892, 0.009323796451543943375 ),
 .UNSPECIFIED. ) ;
#8669=CARTESIAN_POINT ( 'NONE',  ( -2.783900127212157738, 40.00000000000000000, -50.42898717388165153 ) ) ;
#8673=ADVANCED_FACE ( 'NONE', ( #14044, #17731 ), #19238, .F. ) ;
#8675=CARTESIAN_POINT ( 'NONE',  ( -13.63965147459812322, 34.63504322468456564, 58.68815147418794709 ) ) ;
#8676=VERTEX_POINT ( 'NONE', #5259 ) ;
#8679=DIRECTION ( 'NONE',  ( -1.000000000000000000, 0.000000000000000000, 0.000000000000000000 ) ) ;
#8684=AXIS2_PLACEMENT_3D ( 'NONE', #4951, #19158, #20539 ) ;
#8688=CARTESIAN_POINT ( 'NONE',  ( 35.00000000000000000, -4.928932188134504955, 4.258610482196280173E-15 ) ) ;
#8689=VERTEX_POINT ( 'NONE', #3663 ) ;
#8693=AXIS2_PLACEMENT_3D ( 'NONE', #15985, #9549, #1807 ) ;
#8696=CARTESIAN_POINT ( 'NONE',  ( -19.81381843823601585, 22.85613052104876530, -58.09821304537217657 ) ) ;
#8700=DIRECTION ( 'NONE',  ( -0.000000000000000000, -0.000000000000000000, 1.000000000000000000 ) ) ;
#8702=DIRECTION ( 'NONE',  ( -0.000000000000000000, 1.000000000000000000, -0.000000000000000000 ) ) ;
#8706=DIRECTION ( 'NONE',  ( 3.585095183685401065E-15, 0.000000000000000000, -1.000000000000000000 ) ) ;
#8713=AXIS2_PLACEMENT_3D ( 'NONE', #4092, #21729, #2368 ) ;
#8715=ORIENTED_EDGE ( 'NONE', *, *, #15859, .F. ) ;
#8718=CARTESIAN_POINT ( 'NONE',  ( 5.770190843040702511, -4.767707482267821817, 49.21533144469336918 ) ) ;
#8723=CARTESIAN_POINT ( 'NONE',  ( -11.06593724743309082, 39.99999999999999289, -53.99256019164670306 ) ) ;
#8724=EDGE_LOOP ( 'NONE', ( #5307, #3708, #9296, #7828 ) ) ;
#8725=CARTESIAN_POINT ( 'NONE',  ( 0.7809641287214669214, -4.625293788890100011, -46.06432795380058565 ) ) ;
#8726=CARTESIAN_POINT ( 'NONE',  ( 19.73349596156085184, 30.70641346160533303, -58.02568834892367988 ) ) ;
#8728=CARTESIAN_POINT ( 'NONE',  ( 17.99999999999998579, 20.00000000000000355, 103.0000000000000284 ) ) ;
#8733=DIRECTION ( 'NONE',  ( -0.000000000000000000, -0.000000000000000000, 1.000000000000000000 ) ) ;
#8734=CIRCLE ( 'NONE', #21541, 2.500000000000002220 ) ;
#8737=VERTEX_POINT ( 'NONE', #14160 ) ;
#8738=CARTESIAN_POINT ( 'NONE',  ( 28.49999999999998224, 19.99999999999999645, 105.0000000000000142 ) ) ;
#8742=CARTESIAN_POINT ( 'NONE',  ( 42.50000000000000711, -12.00000000000012434, -44.97499999999988773 ) ) ;
#8744=B_SPLINE_SURFACE_WITH_KNOTS ( 'NONE', 1, 3, ( 
 ( #1568, #11763, #6964, #13923, #8554, #22552 ),
 ( #18760, #20590, #17031, #4900, #20831, #12109 ) ),
 .UNSPECIFIED., .F., .F., .F.,
 ( 2, 2 ),
 ( 4, 2, 4 ),
 ( 0.000000000000000000, 1.000000000000000000 ),
 ( 0.000000000000000000, 0.001214050925806519710, 0.002428101851613039420 ),
 .UNSPECIFIED. ) ;
#8751=AXIS2_PLACEMENT_3D ( 'NONE', #19415, #17673, #16068 ) ;
#8752=ORIENTED_EDGE ( 'NONE', *, *, #10684, .T. ) ;
#8754=CARTESIAN_POINT ( 'NONE',  ( 21.56999872847275057, 13.83083564369840701, 58.47776649573041396 ) ) ;
#8755=CARTESIAN_POINT ( 'NONE',  ( 8.604786169551864816, 40.00000000000000000, 53.19510612370975622 ) ) ;
#8758=CARTESIAN_POINT ( 'NONE',  ( 1.039655021832692539, -3.147609295952956909, -46.52691668518789214 ) ) ;
#8759=VERTEX_POINT ( 'NONE', #13211 ) ;
#8761=DIRECTION ( 'NONE',  ( 0.000000000000000000, 0.000000000000000000, 1.000000000000000000 ) ) ;
#8766=DIRECTION ( 'NONE',  ( 0.000000000000000000, -1.000000000000000000, 0.000000000000000000 ) ) ;
#8767=CARTESIAN_POINT ( 'NONE',  ( -4.591783869092104453, 39.86870517915106404, 51.95897982375534241 ) ) ;
#8771=CARTESIAN_POINT ( 'NONE',  ( 19.38379237383783149, 24.94684328524480321, 57.98195591854139508 ) ) ;
#8777=ORIENTED_EDGE ( 'NONE', *, *, #13219, .T. ) ;
#8786=CARTESIAN_POINT ( 'NONE',  ( 2.665759242407653495, 39.95807813352564608, 50.69599102971979221 ) ) ;
#8787=ORIENTED_EDGE ( 'NONE', *, *, #19065, .F. ) ;
#8789=CARTESIAN_POINT ( 'NONE',  ( -9.272092388914145999, 40.00000000000000000, -53.43088570759663725 ) ) ;
#8794=CARTESIAN_POINT ( 'NONE',  ( -19.71583072461107378, 23.39500837205461536, 60.55395521980175033 ) ) ;
#8798=DIRECTION ( 'NONE',  ( 0.000000000000000000, 0.7071067811865474617, 0.7071067811865474617 ) ) ;
#8801=EDGE_CURVE ( 'NONE', #164, #507, #8077, .T. ) ;
#8802=ORIENTED_EDGE ( 'NONE', *, *, #2128, .T. ) ;
#8803=DIRECTION ( 'NONE',  ( -0.000000000000000000, 1.000000000000000000, -0.000000000000000000 ) ) ;
#8805=CYLINDRICAL_SURFACE ( 'NONE', #16385, 2.499999999999998668 ) ;
#8811=DIRECTION ( 'NONE',  ( 0.000000000000000000, 1.000000000000000000, 0.000000000000000000 ) ) ;
#8812=EDGE_LOOP ( 'NONE', ( #14405, #3338, #10665, #1726, #2203, #3603 ) ) ;
#8815=CARTESIAN_POINT ( 'NONE',  ( -90.00000000000000000, 40.00000000000000000, -9.108981535246192915E-16 ) ) ;
#8816=CARTESIAN_POINT ( 'NONE',  ( -35.00000000000000000, -9.000000000000001776, 1.387778780781445676E-14 ) ) ;
#8817=VERTEX_POINT ( 'NONE', #8089 ) ;
#8822=ORIENTED_EDGE ( 'NONE', *, *, #7381, .F. ) ;
#8825=CARTESIAN_POINT ( 'NONE',  ( 0.6683989176583298164, -3.155640224524286275, 47.80307817979240070 ) ) ;
#8826=DIRECTION ( 'NONE',  ( 0.000000000000000000, -1.000000000000000000, 0.000000000000000000 ) ) ;
#8827=DIRECTION ( 'NONE',  ( -1.000000000000000000, 0.000000000000000000, 0.000000000000000000 ) ) ;
#8833=CARTESIAN_POINT ( 'NONE',  ( 19.51193873661505762, 31.10741194645160235, -57.96703944061300007 ) ) ;
#8834=LINE ( 'NONE', #7229, #3508 ) ;
#8835=DIRECTION ( 'NONE',  ( -0.000000000000000000, -0.000000000000000000, -1.000000000000000000 ) ) ;
#8836=ORIENTED_EDGE ( 'NONE', *, *, #7501, .F. ) ;
#8837=CARTESIAN_POINT ( 'NONE',  ( 12.99999999999993960, 42.51666049839543149, 100.0000000000000000 ) ) ;
#8838=CARTESIAN_POINT ( 'NONE',  ( -2.175253701329903144, 39.97152389588116961, -50.35029005139294611 ) ) ;
#8840=ORIENTED_EDGE ( 'NONE', *, *, #19356, .T. ) ;
#8841=CARTESIAN_POINT ( 'NONE',  ( 10.31465995609116604, 2.846668092511916992, 57.27881138849571840 ) ) ;
#8843=( BOUNDED_SURFACE ( )  B_SPLINE_SURFACE ( 3, 2, ( 
 ( #16264, #21315, #15913 ),
 ( #7680, #9168, #9284 ),
 ( #5611, #2414, #5851 ),
 ( #14421, #21429, #7224 ),
 ( #697, #231, #4034 ),
 ( #7449, #9061, #14654 ) ),
 .UNSPECIFIED., .F., .F., .T. ) 
 B_SPLINE_SURFACE_WITH_KNOTS ( ( 4, 2, 4 ),
 ( 3, 3 ),
 ( -8.673617379884035472E-19, 0.002858401832365830338, 0.005716803664731661544 ),
 ( 0.000000000000000000, 1.000000000000000000 ),
 .UNSPECIFIED. ) 
 GEOMETRIC_REPRESENTATION_ITEM ( )  RATIONAL_B_SPLINE_SURFACE ( (
 ( 1.000000000000000000, 0.6290213284793358950, 1.000000000000000000),
 ( 1.000000000000000000, 0.6455195629496804921, 1.000000000000000000),
 ( 1.000000000000000000, 0.6615687397065170838, 1.000000000000000000),
 ( 1.000000000000000000, 0.6920701670982940534, 1.000000000000000000),
 ( 1.000000000000000000, 0.7065285139749719612, 1.000000000000000000),
 ( 1.000000000000000000, 0.7200096751079134716, 1.000000000000000000) ) ) 
 REPRESENTATION_ITEM ( '' )  SURFACE ( )  );
#8853=DIRECTION ( 'NONE',  ( 0.7071067811865524577, 8.659560562354993255E-17, -0.7071067811865426878 ) ) ;
#8854=CARTESIAN_POINT ( 'NONE',  ( 13.56354382738800268, 2.142135623730931471, 56.03997097393685323 ) ) ;
#8855=CARTESIAN_POINT ( 'NONE',  ( 9.689843208404393948, 39.33333333333333570, -54.54983754392740991 ) ) ;
#8856=CARTESIAN_POINT ( 'NONE',  ( 2.026528946947714349, 40.00000000000001421, 49.98891164559377387 ) ) ;
#8857=ADVANCED_FACE ( 'NONE', ( #4984 ), #7140, .T. ) ;
#8859=FACE_BOUND ( 'NONE', #3213, .T. ) ;
#8860=FACE_OUTER_BOUND ( 'NONE', #18983, .T. ) ;
#8861=ORIENTED_EDGE ( 'NONE', *, *, #9476, .T. ) ;
#8864=VERTEX_POINT ( 'NONE', #13990 ) ;
#8866=ORIENTED_EDGE ( 'NONE', *, *, #14488, .F. ) ;
#8868=EDGE_CURVE ( 'NONE', #21245, #22510, #8441, .T. ) ;
#8869=FACE_OUTER_BOUND ( 'NONE', #16894, .T. ) ;
#8870=CARTESIAN_POINT ( 'NONE',  ( -1.105958002183684119, 39.99272032066614457, 49.57516047002052773 ) ) ;
#8871=CARTESIAN_POINT ( 'NONE',  ( 15.89815672374940725, 32.14246426897741316, 59.47617874060763654 ) ) ;
#8872=CARTESIAN_POINT ( 'NONE',  ( 5.833333333333336590, 40.00000000000000000, 40.61164310337068173 ) ) ;
#8875=ORIENTED_EDGE ( 'NONE', *, *, #7534, .F. ) ;
#8876=ORIENTED_EDGE ( 'NONE', *, *, #16352, .F. ) ;
#8877=ORIENTED_EDGE ( 'NONE', *, *, #15916, .F. ) ;
#8879=CARTESIAN_POINT ( 'NONE',  ( -12.27586057105639661, 4.193657236093902618, 55.54740530680980015 ) ) ;
#8881=ADVANCED_FACE ( 'NONE', ( #10456 ), #12781, .F. ) ;
#8882=B_SPLINE_CURVE_WITH_KNOTS ( 'NONE', 3,
 ( #18727, #16785, #20114, #1090, #853, #3034, #1190, #8083, #973, #22057, #6350, #14705, #7844 ),
 .UNSPECIFIED., .F., .F.,
 ( 4, 2, 1, 1, 1, 2, 2, 4 ),
 ( 0.000000000000000000, 0.2499999999999845124, 0.3749999999999741318, 0.4374999999999714673, 0.4687499999999691358, 0.4843749999999679146, 0.4999999999999667488, 1.000000000000000000 ),
 .UNSPECIFIED. ) ;
#8883=LINE ( 'NONE', #15754, #19348 ) ;
#8884=CARTESIAN_POINT ( 'NONE',  ( 4.573707224651647252, 39.86977587139770662, 51.94771479820464322 ) ) ;
#8888=CARTESIAN_POINT ( 'NONE',  ( 23.49999999999998579, 19.99999999999999645, 105.0000000000000142 ) ) ;
#8896=DIRECTION ( 'NONE',  ( 1.000000000000000000, 0.000000000000000000, 0.000000000000000000 ) ) ;
#8902=CIRCLE ( 'NONE', #10720, 2.000000000000002665 ) ;
#8903=CIRCLE ( 'NONE', #847, 2.099999999999997868 ) ;
#8904=VERTEX_POINT ( 'NONE', #729 ) ;
#8905=CARTESIAN_POINT ( 'NONE',  ( 10.27431133777639793, -4.928932188134518277, -51.43682631505696179 ) ) ;
#8907=CARTESIAN_POINT ( 'NONE',  ( 11.16030968682943225, 40.00000000000000711, -54.02479386262969996 ) ) ;
#8909=CIRCLE ( 'NONE', #1606, 2.099999999999997868 ) ;
#8915=ORIENTED_EDGE ( 'NONE', *, *, #15572, .T. ) ;
#8917=FACE_BOUND ( 'NONE', #5338, .T. ) ;
#8920=CARTESIAN_POINT ( 'NONE',  ( 13.76792553423403831, 13.99810558461767407, -45.26963775109937416 ) ) ;
#8926=DIRECTION ( 'NONE',  ( 0.000000000000000000, 0.000000000000000000, -1.000000000000000000 ) ) ;
#8928=AXIS2_PLACEMENT_3D ( 'NONE', #2230, #21480, #18153 ) ;
#8929=ORIENTED_EDGE ( 'NONE', *, *, #10441, .F. ) ;
#8932=ORIENTED_EDGE ( 'NONE', *, *, #9040, .F. ) ;
#8938=CARTESIAN_POINT ( 'NONE',  ( -8.105728697730361532, 40.00000000000000000, 53.00649037880594250 ) ) ;
#8939=ORIENTED_EDGE ( 'NONE', *, *, #14173, .T. ) ;
#8941=FACE_OUTER_BOUND ( 'NONE', #2491, .T. ) ;
#8945=DIRECTION ( 'NONE',  ( 0.000000000000000000, -1.000000000000000000, 0.000000000000000000 ) ) ;
#8948=CARTESIAN_POINT ( 'NONE',  ( -4.556497549088540211, 39.87079204719141501, -51.93698204320140377 ) ) ;
#8949=AXIS2_PLACEMENT_3D ( 'NONE', #21646, #7432, #16128 ) ;
#8952=CARTESIAN_POINT ( 'NONE',  ( -7.505578006075205089, 1.461761173328240515, 55.63523492904089096 ) ) ;
#8955=ORIENTED_EDGE ( 'NONE', *, *, #4401, .T. ) ;
#8957=EDGE_LOOP ( 'NONE', ( #16141, #3902 ) ) ;
#8961=CIRCLE ( 'NONE', #15165, 2.099999999999997868 ) ;
#8962=CYLINDRICAL_SURFACE ( 'NONE', #15994, 20.00000000000000000 ) ;
#8963=CARTESIAN_POINT ( 'NONE',  ( 3.022692775171828217, 39.94544418562367838, -50.94009349721213198 ) ) ;
#8964=CARTESIAN_POINT ( 'NONE',  ( 8.578904124028513323, 40.00000000000000000, 53.18551242646393717 ) ) ;
#8965=VERTEX_POINT ( 'NONE', #11028 ) ;
#8969=CARTESIAN_POINT ( 'NONE',  ( -1.436159831096171624, -1.268900497114691772, 49.23900052097178559 ) ) ;
#8972=CARTESIAN_POINT ( 'NONE',  ( 17.99999999999998579, 20.00000000000000355, 105.0000000000000142 ) ) ;
#8974=DIRECTION ( 'NONE',  ( -0.000000000000000000, -0.000000000000000000, 1.000000000000000000 ) ) ;
#8981=CARTESIAN_POINT ( 'NONE',  ( 8.732266002733743093, 39.99999999999999289, -53.24192878695249931 ) ) ;
#8982=CARTESIAN_POINT ( 'NONE',  ( 19.97049456717391891, 21.17381189076418124, 60.61481192459388723 ) ) ;
#8986=CARTESIAN_POINT ( 'NONE',  ( 35.00000000000000000, -4.928932188134504955, 57.07106781186552524 ) ) ;
#8989=ORIENTED_EDGE ( 'NONE', *, *, #3031, .F. ) ;
#8997=B_SPLINE_CURVE_WITH_KNOTS ( 'NONE', 3,
 ( #10422, #13622, #10310, #10537, #15700, #1739, #8723, #15, #20984, #10203, #5073, #8492 ),
 .UNSPECIFIED., .F., .F.,
 ( 4, 1, 1, 1, 1, 2, 2, 4 ),
 ( 0.000000000000000000, 0.2500000000000013323, 0.3750000000000022760, 0.4375000000000013878, 0.4687500000000019984, 0.4843750000000033862, 0.5000000000000047740, 1.000000000000000000 ),
 .UNSPECIFIED. ) ;
#8999=DIRECTION ( 'NONE',  ( -0.000000000000000000, 1.000000000000000000, -0.000000000000000000 ) ) ;
#9000=CARTESIAN_POINT ( 'NONE',  ( 0.03025501645077945459, 39.99999465686278199, 48.75751133701592011 ) ) ;
#9002=ORIENTED_EDGE ( 'NONE', *, *, #6708, .T. ) ;
#9006=LINE ( 'NONE', #14259, #15918 ) ;
#9008=CARTESIAN_POINT ( 'NONE',  ( -18.87121696173700514, 26.69448804128720099, 60.34297443853448328 ) ) ;
#9009=CIRCLE ( 'NONE', #17794, 8.999999999999966249 ) ;
#9013=FACE_OUTER_BOUND ( 'NONE', #10497, .T. ) ;
#9014=EDGE_CURVE ( 'NONE', #21600, #16362, #14525, .T. ) ;
#9015=CYLINDRICAL_SURFACE ( 'NONE', #21111, 20.00000000000000000 ) ;
#9020=ORIENTED_EDGE ( 'NONE', *, *, #7122, .F. ) ;
#9021=CARTESIAN_POINT ( 'NONE',  ( 3.001573872050378622, -1.099462678408570149, -50.31569927527887387 ) ) ;
#9023=AXIS2_PLACEMENT_3D ( 'NONE', #2045, #22584, #10398 ) ;
#9028=CARTESIAN_POINT ( 'NONE',  ( -17.38307674301858796, 10.07685590252459029, 59.93367040492846343 ) ) ;
#9029=CARTESIAN_POINT ( 'NONE',  ( -13.25803659942197754, 34.99815359651601909, -58.54720450724500580 ) ) ;
#9032=VERTEX_POINT ( 'NONE', #7820 ) ;
#9039=ORIENTED_EDGE ( 'NONE', *, *, #1610, .T. ) ;
#9040=EDGE_CURVE ( 'NONE', #17179, #8864, #14452, .T. ) ;
#9041=CARTESIAN_POINT ( 'NONE',  ( 42.50000000000000711, -9.600000000000001421, 45.40000000000001279 ) ) ;
#9043=DIRECTION ( 'NONE',  ( -1.000000000000000000, 0.000000000000000000, 0.000000000000000000 ) ) ;
#9044=AXIS2_PLACEMENT_3D ( 'NONE', #16603, #7556, #20052 ) ;
#9045=DIRECTION ( 'NONE',  ( -0.000000000000000000, -1.000000000000000000, -0.000000000000000000 ) ) ;
#9046=EDGE_CURVE ( 'NONE', #3399, #19609, #640, .T. ) ;
#9047=VERTEX_POINT ( 'NONE', #11485 ) ;
#9052=CARTESIAN_POINT ( 'NONE',  ( 0.2369875743634299314, 39.99966999001385659, -48.91756785322892398 ) ) ;
#9054=CARTESIAN_POINT ( 'NONE',  ( -10.60627602730582275, 0.5940385038083396685, 54.69850067894232382 ) ) ;
#9055=CARTESIAN_POINT ( 'NONE',  ( -34.99999999999981526, 24.73819270004212356, 54.99999999999922551 ) ) ;
#9056=FACE_OUTER_BOUND ( 'NONE', #18481, .T. ) ;
#9061=CARTESIAN_POINT ( 'NONE',  ( -8.349099696861340902, 1.803277857259562245, -53.93591755799871379 ) ) ;
#9065=CARTESIAN_POINT ( 'NONE',  ( 14.95260096911750303, 3.243207204902308405, -56.55590526898570403 ) ) ;
#9066=CARTESIAN_POINT ( 'NONE',  ( 42.50000000000000711, -12.00000000000000000, 47.50000000000000711 ) ) ;
#9068=VERTEX_POINT ( 'NONE', #13286 ) ;
#9071=CARTESIAN_POINT ( 'NONE',  ( -0.5323815408128229620, 39.99832331801214735, -49.14386499772781036 ) ) ;
#9073=CIRCLE ( 'NONE', #4336, 30.00000000000000000 ) ;
#9074=CARTESIAN_POINT ( 'NONE',  ( 90.00000000000000000, 39.97500000000000142, 2.500000000000001332 ) ) ;
#9076=AXIS2_PLACEMENT_3D ( 'NONE', #15093, #4367, #15212 ) ;
#9077=VECTOR ( 'NONE', #6257, 1000.000000000000000 ) ;
#9081=ORIENTED_EDGE ( 'NONE', *, *, #5601, .F. ) ;
#9083=ORIENTED_EDGE ( 'NONE', *, *, #848, .T. ) ;
#9085=DIRECTION ( 'NONE',  ( -1.000000000000000000, 0.000000000000000000, 0.000000000000000000 ) ) ;
#9088=AXIS2_PLACEMENT_3D ( 'NONE', #9962, #6648, #3220 ) ;
#9090=CARTESIAN_POINT ( 'NONE',  ( 35.00000000000000711, -5.000000000000000000, -57.00000000000001421 ) ) ;
#9094=CARTESIAN_POINT ( 'NONE',  ( -12.60179598819648739, 38.53795549125497644, -55.66391160832503004 ) ) ;
#9096=AXIS2_PLACEMENT_3D ( 'NONE', #7487, #5771, #16534 ) ;
#9101=ORIENTED_EDGE ( 'NONE', *, *, #12803, .F. ) ;
#9102=CARTESIAN_POINT ( 'NONE',  ( -3.286600300096431288E-14, 40.00000000000000000, -48.73397172404478539 ) ) ;
#9103=CARTESIAN_POINT ( 'NONE',  ( -2.546709079545449672, 39.84786395731773467, 51.61893211308341023 ) ) ;
#9106=CARTESIAN_POINT ( 'NONE',  ( 21.60080777693143972, 26.06115151610029912, 58.48488838346896301 ) ) ;
#9108=CARTESIAN_POINT ( 'NONE',  ( 11.88509939555964046, 36.18356491089507188, -55.39957109942752567 ) ) ;
#9109=CONICAL_SURFACE ( 'NONE', #15302, 2.524999999999999467, 0.7853981633974482790 ) ;
#9111=ORIENTED_EDGE ( 'NONE', *, *, #20140, .T. ) ;
#9112=EDGE_CURVE ( 'NONE', #18984, #12705, #11710, .T. ) ;
#9117=FACE_OUTER_BOUND ( 'NONE', #14616, .T. ) ;
#9118=CARTESIAN_POINT ( 'NONE',  ( -10.84015308335310479, 39.16451817969218041, -54.95776488303458507 ) ) ;
#9119=DIRECTION ( 'NONE',  ( 0.000000000000000000, 0.7071067811865326957, 0.7071067811865622277 ) ) ;
#9121=CARTESIAN_POINT ( 'NONE',  ( 42.50000000000000711, -12.00000000000000000, -45.00000000000000000 ) ) ;
#9122=AXIS2_PLACEMENT_3D ( 'NONE', #21386, #4091, #7637 ) ;
#9123=ORIENTED_EDGE ( 'NONE', *, *, #18406, .T. ) ;
#9124=FACE_OUTER_BOUND ( 'NONE', #12730, .T. ) ;
#9129=EDGE_CURVE ( 'NONE', #10746, #9068, #3353, .T. ) ;
#9137=B_SPLINE_CURVE_WITH_KNOTS ( 'NONE', 3,
 ( #15226, #22246, #15342, #11910, #22361, #6124 ),
 .UNSPECIFIED., .F., .F.,
 ( 4, 2, 4 ),
 ( 3.576224061345498009E-18, 0.003173601132114241274, 0.006347202264228479079 ),
 .UNSPECIFIED. ) ;
#9140=CARTESIAN_POINT ( 'NONE',  ( 11.59091061707581893, 40.00000000000000000, -54.17810196248734655 ) ) ;
#9141=CARTESIAN_POINT ( 'NONE',  ( 44.60000000000000853, -9.600000000000001421, 47.50000000000000711 ) ) ;
#9144=DIRECTION ( 'NONE',  ( -0.000000000000000000, 1.000000000000000000, -0.000000000000000000 ) ) ;
#9151=DIRECTION ( 'NONE',  ( -1.000000000000000000, 0.000000000000000000, 0.000000000000000000 ) ) ;
#9153=EDGE_CURVE ( 'NONE', #21800, #22583, #20643, .T. ) ;
#9159=ORIENTED_EDGE ( 'NONE', *, *, #12120, .T. ) ;
#9161=ORIENTED_EDGE ( 'NONE', *, *, #9153, .T. ) ;
#9168=CARTESIAN_POINT ( 'NONE',  ( -11.68987541777273265, 3.735186999524350959, -55.40064774186661367 ) ) ;
#9173=AXIS2_PLACEMENT_3D ( 'NONE', #11840, #20673, #15384 ) ;
#9178=ADVANCED_FACE ( 'NONE', ( #1397 ), #3579, .F. ) ;
#9179=EDGE_CURVE ( 'NONE', #21079, #11081, #12051, .T. ) ;
#9182=EDGE_LOOP ( 'NONE', ( #10531, #5419, #20690 ) ) ;
#9192=CARTESIAN_POINT ( 'NONE',  ( 3.997614489231452239, 39.99999999999999289, -51.09533703001513771 ) ) ;
#9194=VERTEX_POINT ( 'NONE', #22379 ) ;
#9195=DIRECTION ( 'NONE',  ( 0.000000000000000000, -1.000000000000000000, 0.000000000000000000 ) ) ;
#9200=AXIS2_PLACEMENT_3D ( 'NONE', #15456, #13734, #8379 ) ;
#9201=LINE ( 'NONE', #14226, #3189 ) ;
#9202=ORIENTED_EDGE ( 'NONE', *, *, #14699, .F. ) ;
#9206=CARTESIAN_POINT ( 'NONE',  ( -4.589505318347434581, 39.46976832855466455, 53.62193830992121235 ) ) ;
#9207=DIRECTION ( 'NONE',  ( 0.000000000000000000, -1.000000000000000000, 0.000000000000000000 ) ) ;
#9209=CARTESIAN_POINT ( 'NONE',  ( 9.952189117650862116, 40.00000000000000000, -53.64426396172072486 ) ) ;
#9210=CARTESIAN_POINT ( 'NONE',  ( 20.89003165053258826, 11.75591475223826876, 58.31867307082493568 ) ) ;
#9211=DIRECTION ( 'NONE',  ( -0.000000000000000000, -1.000000000000000000, -0.000000000000000000 ) ) ;
#9212=EDGE_CURVE ( 'NONE', #20378, #5648, #17470, .T. ) ;
#9218=EDGE_CURVE ( 'NONE', #14094, #9683, #12325, .T. ) ;
#9220=ORIENTED_EDGE ( 'NONE', *, *, #18406, .F. ) ;
#9222=CARTESIAN_POINT ( 'NONE',  ( -11.86180952233172725, 39.00000000000000000, -55.35904751184885697 ) ) ;
#9223=CARTESIAN_POINT ( 'NONE',  ( 35.00000000000000000, -5.000000000000000000, 4.258610482196280173E-15 ) ) ;
#9229=DIRECTION ( 'NONE',  ( -0.000000000000000000, -1.000000000000000000, -0.000000000000000000 ) ) ;
#9230=CARTESIAN_POINT ( 'NONE',  ( -90.00000000000000000, 40.00000000000000000, -2.500000000000003109 ) ) ;
#9232=AXIS2_PLACEMENT_3D ( 'NONE', #9459, #5903, #7392 ) ;
#9233=DIRECTION ( 'NONE',  ( 0.000000000000000000, -1.000000000000000000, 0.000000000000000000 ) ) ;
#9235=CARTESIAN_POINT ( 'NONE',  ( -3.171166886497724935, 39.94220484565181550, 51.05051218202238061 ) ) ;
#9236=CARTESIAN_POINT ( 'NONE',  ( 17.99999999999998579, 20.00000000000000711, -105.0000000000000142 ) ) ;
#9237=ORIENTED_EDGE ( 'NONE', *, *, #11097, .T. ) ;
#9238=ORIENTED_EDGE ( 'NONE', *, *, #7625, .T. ) ;
#9243=CARTESIAN_POINT ( 'NONE',  ( -5.007336801250276359, 0.5949183078238818867, -54.03289733825791075 ) ) ;
#9244=CIRCLE ( 'NONE', #5967, 57.07106781186551103 ) ;
#9248=CARTESIAN_POINT ( 'NONE',  ( 12.84899528830093196, 2.142135623730927030, 57.90797000640142045 ) ) ;
#9249=CARTESIAN_POINT ( 'NONE',  ( -16.09174361829569122, 8.097379805989266544, 59.53987500167126257 ) ) ;
#9250=CARTESIAN_POINT ( 'NONE',  ( -12.81940492552891797, 35.37234179763732556, -55.76972854553744696 ) ) ;
#9252=LINE ( 'NONE', #2623, #9722 ) ;
#9253=EDGE_CURVE ( 'NONE', #8612, #21119, #21116, .T. ) ;
#9257=CARTESIAN_POINT ( 'NONE',  ( -1.387778780781445518E-14, 20.00000000000000355, 100.0000000000000000 ) ) ;
#9258=CARTESIAN_POINT ( 'NONE',  ( -1.255529093608962921, 39.96306425836119303, -50.19904361858059616 ) ) ;
#9260=FACE_OUTER_BOUND ( 'NONE', #10088, .T. ) ;
#9264=VERTEX_POINT ( 'NONE', #13745 ) ;
#9268=AXIS2_PLACEMENT_3D ( 'NONE', #9782, #16774, #18720 ) ;
#9269=CARTESIAN_POINT ( 'NONE',  ( 18.15458487487614647, 6.756534690976822688, -57.58998093367154070 ) ) ;
#9271=ORIENTED_EDGE ( 'NONE', *, *, #10561, .T. ) ;
#9274=DIRECTION ( 'NONE',  ( -0.000000000000000000, -1.000000000000000000, -0.000000000000000000 ) ) ;
#9278=CARTESIAN_POINT ( 'NONE',  ( 35.00000000000000000, -9.000000000000001776, 4.258610482196280173E-15 ) ) ;
#9279=AXIS2_PLACEMENT_3D ( 'NONE', #13203, #16552, #4420 ) ;
#9280=DIRECTION ( 'NONE',  ( -0.000000000000000000, -0.000000000000000000, -1.000000000000000000 ) ) ;
#9281=ORIENTED_EDGE ( 'NONE', *, *, #4880, .F. ) ;
#9282=DIRECTION ( 'NONE',  ( -0.7752116086454780008, 0.5577761202038525878, 0.2965345874457610553 ) ) ;
#9283=AXIS2_PLACEMENT_3D ( 'NONE', #7920, #20294, #7796 ) ;
#9284=CARTESIAN_POINT ( 'NONE',  ( -11.00126833625150802, 3.276569432399059512, -57.62199738687990447 ) ) ;
#9290=EDGE_CURVE ( 'NONE', #15500, #22647, #10130, .T. ) ;
#9291=CARTESIAN_POINT ( 'NONE',  ( -26.00000000000001421, 19.99999999999982947, 60.00099999999999767 ) ) ;
#9293=CARTESIAN_POINT ( 'NONE',  ( -1.387778780781445676E-14, 20.00000000000000000, -105.0020000000000095 ) ) ;
#9294=CARTESIAN_POINT ( 'NONE',  ( -5.833333333333328596, 33.81926995981417861, 40.61164310337068173 ) ) ;
#9295=CARTESIAN_POINT ( 'NONE',  ( -4.516278128484037424, 39.87315170859984192, -51.91186101216593585 ) ) ;
#9296=ORIENTED_EDGE ( 'NONE', *, *, #7650, .F. ) ;
#9297=CARTESIAN_POINT ( 'NONE',  ( 34.99999999999980815, 28.00000000000000000, 54.99999999999922551 ) ) ;
#9299=DIRECTION ( 'NONE',  ( 0.000000000000000000, 0.000000000000000000, -1.000000000000000000 ) ) ;
#9304=ORIENTED_EDGE ( 'NONE', *, *, #1067, .T. ) ;
#9305=EDGE_LOOP ( 'NONE', ( #19417, #21675, #21571 ) ) ;
#9307=ADVANCED_FACE ( 'NONE', ( #12822 ), #17990, .F. ) ;
#9308=ADVANCED_FACE ( 'NONE', ( #1955 ), #14077, .F. ) ;
#9309=EDGE_LOOP ( 'NONE', ( #20973, #7136, #14241, #3385 ) ) ;
#9310=DIRECTION ( 'NONE',  ( -0.000000000000000000, 1.000000000000000000, -0.000000000000000000 ) ) ;
#9315=ORIENTED_EDGE ( 'NONE', *, *, #13579, .T. ) ;
#9318=VERTEX_POINT ( 'NONE', #5614 ) ;
#9320=CARTESIAN_POINT ( 'NONE',  ( -17.96165932904281348, 6.521477064918317801, -57.53061250216237710 ) ) ;
#9323=CARTESIAN_POINT ( 'NONE',  ( -15.50000000000011013, 42.51666049839536043, 100.0000000000000000 ) ) ;
#9325=CARTESIAN_POINT ( 'NONE',  ( 9.786525054697406745, 39.51684776735954330, 54.52238233457818239 ) ) ;
#9328=CARTESIAN_POINT ( 'NONE',  ( -5.833333333333339255, 39.00000000000000711, -40.61164310337066041 ) ) ;
#9331=CARTESIAN_POINT ( 'NONE',  ( 12.26943921815721517, 35.80002840870928793, 58.15275698935946735 ) ) ;
#9335=FACE_OUTER_BOUND ( 'NONE', #13954, .T. ) ;
#9337=AXIS2_PLACEMENT_3D ( 'NONE', #3313, #22335, #8122 ) ;
#9338=ORIENTED_EDGE ( 'NONE', *, *, #11285, .T. ) ;
#9343=CARTESIAN_POINT ( 'NONE',  ( 35.00000000000000000, -5.000000000000000000, 4.258610482196280173E-15 ) ) ;
#9346=EDGE_LOOP ( 'NONE', ( #13611, #7975, #9870, #4290, #22205, #9220 ) ) ;
#9348=CARTESIAN_POINT ( 'NONE',  ( -8.479740367040006888, -4.901256658985764680, 50.57596245086825348 ) ) ;
#9349=CIRCLE ( 'NONE', #12255, 2.500000000000002220 ) ;
#9353=LINE ( 'NONE', #2361, #8640 ) ;
#9354=CARTESIAN_POINT ( 'NONE',  ( 42.50000000000000711, -12.00000000000000000, -54.00000000000000000 ) ) ;
#9369=AXIS2_PLACEMENT_3D ( 'NONE', #4567, #18654, #2732 ) ;
#9373=CARTESIAN_POINT ( 'NONE',  ( -1.788720539129516747E-14, -0.8525878274356358810, 48.47769062749615188 ) ) ;
#9374=DIRECTION ( 'NONE',  ( -1.000000000000000000, 0.000000000000000000, 0.000000000000000000 ) ) ;
#9377=CARTESIAN_POINT ( 'NONE',  ( -0.7832251647695825936, 40.00000000000098055, -49.34584158999207659 ) ) ;
#9379=AXIS2_PLACEMENT_3D ( 'NONE', #17314, #13751, #22273 ) ;
#9380=CARTESIAN_POINT ( 'NONE',  ( 35.00000000000058265, 24.73819270004212356, -55.00000000000076028 ) ) ;
#9385=DIRECTION ( 'NONE',  ( -0.000000000000000000, -0.000000000000000000, -1.000000000000000000 ) ) ;
#9389=VERTEX_POINT ( 'NONE', #14424 ) ;
#9391=DIRECTION ( 'NONE',  ( 0.000000000000000000, 0.000000000000000000, 1.000000000000000000 ) ) ;
#9395=CARTESIAN_POINT ( 'NONE',  ( -35.00000000000000000, 40.00000000000000000, 1.387778780781445676E-14 ) ) ;
#9396=EDGE_CURVE ( 'NONE', #9318, #6579, #16742, .T. ) ;
#9397=CARTESIAN_POINT ( 'NONE',  ( 35.00000000000000000, 40.00000000000000000, -58.99999999999993605 ) ) ;
#9399=AXIS2_PLACEMENT_3D ( 'NONE', #1815, #17837, #17719 ) ;
#9405=ORIENTED_EDGE ( 'NONE', *, *, #10524, .F. ) ;
#9407=CARTESIAN_POINT ( 'NONE',  ( -5.233853366103144999, 39.99999999999999289, 51.72875135548209613 ) ) ;
#9408=DIRECTION ( 'NONE',  ( 0.000000000000000000, 0.000000000000000000, 1.000000000000000000 ) ) ;
#9410=CARTESIAN_POINT ( 'NONE',  ( 35.00000000000000000, -9.000000000000001776, 4.258610482196280173E-15 ) ) ;
#9411=CARTESIAN_POINT ( 'NONE',  ( -35.00000000000000000, -9.000000000000001776, 9.000000000000015987 ) ) ;
#9414=ORIENTED_EDGE ( 'NONE', *, *, #14031, .F. ) ;
#9415=CARTESIAN_POINT ( 'NONE',  ( -42.50000000000000711, -5.000000000000000000, 45.40000000000001279 ) ) ;
#9417=ORIENTED_EDGE ( 'NONE', *, *, #19831, .F. ) ;
#9419=AXIS2_PLACEMENT_3D ( 'NONE', #8271, #15241, #22262 ) ;
#9420=ORIENTED_EDGE ( 'NONE', *, *, #11112, .F. ) ;
#9423=AXIS2_PLACEMENT_3D ( 'NONE', #2748, #9274, #566 ) ;
#9425=CARTESIAN_POINT ( 'NONE',  ( 11.08851315719092057, 40.00000000000000000, 54.00022650832064386 ) ) ;
#9426=DIRECTION ( 'NONE',  ( 0.000000000000000000, -1.000000000000000000, 0.000000000000000000 ) ) ;
#9427=DIRECTION ( 'NONE',  ( 0.000000000000000000, 0.000000000000000000, -1.000000000000000000 ) ) ;
#9428=DIRECTION ( 'NONE',  ( 1.000000000000000000, 0.000000000000000000, 0.000000000000000000 ) ) ;
#9430=ORIENTED_EDGE ( 'NONE', *, *, #18211, .F. ) ;
#9434=CARTESIAN_POINT ( 'NONE',  ( 0.3475255461657534850, -0.009191383995502665563, 50.24722912075116454 ) ) ;
#9436=CARTESIAN_POINT ( 'NONE',  ( 16.09174361829564504, 8.097379805989254109, -59.53987500167121993 ) ) ;
#9438=DIRECTION ( 'NONE',  ( -1.000000000000000000, 0.000000000000000000, 0.000000000000000000 ) ) ;
#9440=CARTESIAN_POINT ( 'NONE',  ( 1.801771875243787013, 0.06844342149310433943, 51.82845797839667767 ) ) ;
#9441=AXIS2_PLACEMENT_3D ( 'NONE', #5878, #4160, #9428 ) ;
#9443=CARTESIAN_POINT ( 'NONE',  ( 5.905661774832184463, 39.12131255383282991, 53.51378690820485673 ) ) ;
#9450=DIRECTION ( 'NONE',  ( -0.000000000000000000, -0.000000000000000000, -1.000000000000000000 ) ) ;
#9453=CARTESIAN_POINT ( 'NONE',  ( 12.99999999999993960, 42.51666049839543149, -105.0000000000000142 ) ) ;
#9455=EDGE_LOOP ( 'NONE', ( #13776, #5692, #18644 ) ) ;
#9459=CARTESIAN_POINT ( 'NONE',  ( 42.50000000000000711, -12.00000000000012434, 47.50000000000000711 ) ) ;
#9461=CARTESIAN_POINT ( 'NONE',  ( -11.69583325982488908, 39.02781355213843995, -55.28967510482120673 ) ) ;
#9463=CARTESIAN_POINT ( 'NONE',  ( 34.99999999999980815, 26.00000000000000355, 54.99999999999922551 ) ) ;
#9470=ORIENTED_EDGE ( 'NONE', *, *, #6010, .T. ) ;
#9471=CARTESIAN_POINT ( 'NONE',  ( 12.24744603030438839, 40.00000000000000000, -54.43639671998947449 ) ) ;
#9474=CARTESIAN_POINT ( 'NONE',  ( -35.00000000000000000, -9.000000000000001776, 1.387778780781445676E-14 ) ) ;
#9476=EDGE_CURVE ( 'NONE', #5386, #13427, #2533, .T. ) ;
#9477=EDGE_CURVE ( 'NONE', #14267, #12299, #12704, .T. ) ;
#9479=CARTESIAN_POINT ( 'NONE',  ( 17.99999999999998579, 20.00000000000000711, -102.0000000000000142 ) ) ;
#9481=AXIS2_PLACEMENT_3D ( 'NONE', #3348, #8489, #22484 ) ;
#9486=DIRECTION ( 'NONE',  ( 0.000000000000000000, 0.000000000000000000, 1.000000000000000000 ) ) ;
#9488=AXIS2_PLACEMENT_3D ( 'NONE', #9976, #21926, #16969 ) ;
#9489=DIRECTION ( 'NONE',  ( 0.000000000000000000, 0.7071067811865474617, 0.7071067811865474617 ) ) ;
#9490=CARTESIAN_POINT ( 'NONE',  ( 7.416183817405959028E-14, -1.031411640100015070, 48.34207013941295372 ) ) ;
#9492=CARTESIAN_POINT ( 'NONE',  ( -9.375585286557477360, 39.53990934012379910, -54.37755512015218784 ) ) ;
#9493=DIRECTION ( 'NONE',  ( -0.000000000000000000, 1.000000000000000000, -0.000000000000000000 ) ) ;
#9497=CARTESIAN_POINT ( 'NONE',  ( -34.99999999999980815, 40.00000000000000000, 52.89999999999922409 ) ) ;
#9498=DIRECTION ( 'NONE',  ( -0.000000000000000000, -0.000000000000000000, -1.000000000000000000 ) ) ;
#9501=VERTEX_POINT ( 'NONE', #16384 ) ;
#9502=ORIENTED_EDGE ( 'NONE', *, *, #2249, .F. ) ;
#9503=AXIS2_PLACEMENT_3D ( 'NONE', #16585, #21409, #895 ) ;
#9508=ORIENTED_EDGE ( 'NONE', *, *, #9724, .T. ) ;
#9511=CARTESIAN_POINT ( 'NONE',  ( 7.434579289837093263, 39.99999999999999289, -52.73242323840388934 ) ) ;
#9513=CARTESIAN_POINT ( 'NONE',  ( 3.946564805737537984, 39.90443716270423380, -51.55060807443248194 ) ) ;
#9515=AXIS2_PLACEMENT_3D ( 'NONE', #8450, #1346, #6733 ) ;
#9516=ORIENTED_EDGE ( 'NONE', *, *, #12978, .F. ) ;
#9518=CARTESIAN_POINT ( 'NONE',  ( 10.07716038307521345, 39.27871711258762133, -54.68297691365300039 ) ) ;
#9522=DIRECTION ( 'NONE',  ( 0.000000000000000000, 0.000000000000000000, 1.000000000000000000 ) ) ;
#9524=DIRECTION ( 'NONE',  ( 0.000000000000000000, 0.000000000000000000, 1.000000000000000000 ) ) ;
#9527=AXIS2_PLACEMENT_3D ( 'NONE', #9278, #8826, #16260 ) ;
#9534=CARTESIAN_POINT ( 'NONE',  ( 9.952189117650823036, 40.00000000000000000, 53.64426396172073197 ) ) ;
#9535=CARTESIAN_POINT ( 'NONE',  ( 8.460114887479386780, -4.900635315004578274, 50.56657553898163115 ) ) ;
#9538=CARTESIAN_POINT ( 'NONE',  ( 15.50000000000024336, -2.516660498395250745, 105.0000000000000142 ) ) ;
#9539=CARTESIAN_POINT ( 'NONE',  ( -18.00000000000001421, 20.00000000000000711, 103.0000000000000284 ) ) ;
#9543=EDGE_LOOP ( 'NONE', ( #18859, #12253, #1792, #12098 ) ) ;
#9547=CARTESIAN_POINT ( 'NONE',  ( 11.68090480754629112, 3.765577839755377187, -57.90797000640139913 ) ) ;
#9549=DIRECTION ( 'NONE',  ( -0.000000000000000000, -1.000000000000000000, -0.000000000000000000 ) ) ;
#9550=ORIENTED_EDGE ( 'NONE', *, *, #13041, .T. ) ;
#9551=CARTESIAN_POINT ( 'NONE',  ( 7.073804381388024254, 38.72385617084731280, 54.13593115560357205 ) ) ;
#9552=CARTESIAN_POINT ( 'NONE',  ( -7.882609639814679786E-15, -9.552912840896525389E-26, -50.50395615645409464 ) ) ;
#9555=EDGE_CURVE ( 'NONE', #8509, #9389, #20286, .T. ) ;
#9556=CARTESIAN_POINT ( 'NONE',  ( 17.16827611621489424, 34.47540479398339386, 57.28984973304910255 ) ) ;
#9558=CIRCLE ( 'NONE', #1132, 15.00000000000000000 ) ;
#9562=EDGE_CURVE ( 'NONE', #478, #13151, #9564, .T. ) ;
#9564=B_SPLINE_CURVE_WITH_KNOTS ( 'NONE', 3,
 ( #11452, #9855, #9518, #16843, #18440, #18558, #18329, #9737, #1142, #4589, #16724, #14872, #8135 ),
 .UNSPECIFIED., .F., .F.,
 ( 4, 2, 1, 1, 1, 2, 2, 4 ),
 ( 0.000000000000000000, 0.2499999999999895639, 0.3749999999999843459, 0.4374999999999821809, 0.4687499999999784617, 0.4843749999999783507, 0.4999999999999782396, 1.000000000000000000 ),
 .UNSPECIFIED. ) ;
#9570=CARTESIAN_POINT ( 'NONE',  ( 0.002911692990617354218, 40.00000000000000711, 48.73623850383051348 ) ) ;
#9571=VERTEX_POINT ( 'NONE', #21663 ) ;
#9572=ADVANCED_FACE ( 'NONE', ( #6075 ), #15992, .F. ) ;
#9578=CONICAL_SURFACE ( 'NONE', #22401, 2.524999999999999467, 0.7853981633974482790 ) ;
#9585=CARTESIAN_POINT ( 'NONE',  ( -18.14868794606802282, 11.58103667096326639, 57.62894917896124980 ) ) ;
#9589=CIRCLE ( 'NONE', #8496, 16.99999999999998579 ) ;
#9591=CARTESIAN_POINT ( 'NONE',  ( -4.295527433237782828E-15, -1.236374842841486021, 48.24164917503448180 ) ) ;
#9593=FACE_OUTER_BOUND ( 'NONE', #16380, .T. ) ;
#9597=DIRECTION ( 'NONE',  ( -0.000000000000000000, 1.000000000000000000, -0.000000000000000000 ) ) ;
#9600=DIRECTION ( 'NONE',  ( 0.000000000000000000, 0.7071067811865507924, 0.7071067811865441310 ) ) ;
#9601=LINE ( 'NONE', #16587, #15856 ) ;
#9604=EDGE_LOOP ( 'NONE', ( #2152, #6198 ) ) ;
#9605=LINE ( 'NONE', #21995, #18088 ) ;
#9608=EDGE_CURVE ( 'NONE', #8022, #16638, #5483, .T. ) ;
#9610=AXIS2_PLACEMENT_3D ( 'NONE', #15257, #6341, #844 ) ;
#9612=CARTESIAN_POINT ( 'NONE',  ( 5.188165876950928457, 39.99999999999999289, -51.70385275873069020 ) ) ;
#9613=ORIENTED_EDGE ( 'NONE', *, *, #16512, .T. ) ;
#9615=CARTESIAN_POINT ( 'NONE',  ( 12.24744603029285273, 40.00000000000000000, 54.43639671998466412 ) ) ;
#9616=CARTESIAN_POINT ( 'NONE',  ( -8.256135806682724620, -0.3920627093389371653, 55.63523492904089096 ) ) ;
#9618=CARTESIAN_POINT ( 'NONE',  ( -14.31754202316403735, 5.927758996452408446, -58.94936959136224885 ) ) ;
#9620=CARTESIAN_POINT ( 'NONE',  ( -9.727693426874370886, 39.99999999999998579, 53.57919861644133874 ) ) ;
#9621=ADVANCED_FACE ( 'NONE', ( #9593 ), #20691, .F. ) ;
#9623=DIRECTION ( 'NONE',  ( -0.000000000000000000, 1.000000000000000000, -0.000000000000000000 ) ) ;
#9626=CARTESIAN_POINT ( 'NONE',  ( -12.24744603030441148, 40.00000000000000000, 54.43639671998950291 ) ) ;
#9630=CARTESIAN_POINT ( 'NONE',  ( 9.103081159015365742, 0.03030367950460663429, 53.87333532811653214 ) ) ;
#9632=CARTESIAN_POINT ( 'NONE',  ( -10.63866000424708247, 30.58060543830997702, 43.66469350997160603 ) ) ;
#9634=AXIS2_PLACEMENT_3D ( 'NONE', #11166, #2478, #7629 ) ;
#9635=ORIENTED_EDGE ( 'NONE', *, *, #20140, .F. ) ;
#9638=AXIS2_PLACEMENT_3D ( 'NONE', #5490, #12572, #3674 ) ;
#9640=VECTOR ( 'NONE', #4933, 1000.000000000000114 ) ;
#9642=FACE_BOUND ( 'NONE', #3238, .T. ) ;
#9645=CYLINDRICAL_SURFACE ( 'NONE', #2947, 49.99999999999998579 ) ;
#9649=FACE_OUTER_BOUND ( 'NONE', #10571, .T. ) ;
#9650=EDGE_LOOP ( 'NONE', ( #10276, #8601, #5144, #15479 ) ) ;
#9651=CARTESIAN_POINT ( 'NONE',  ( -14.92530643917655730, 18.45549920837825653, -45.79309713780077828 ) ) ;
#9652=EDGE_CURVE ( 'NONE', #21024, #21115, #11997, .T. ) ;
#9653=CARTESIAN_POINT ( 'NONE',  ( -14.98269809772828864, 3.197274675470663574, -56.58282704237542760 ) ) ;
#9655=CARTESIAN_POINT ( 'NONE',  ( 9.689843208404433028, 39.33333333333334991, 54.54983754392749518 ) ) ;
#9657=CARTESIAN_POINT ( 'NONE',  ( -0.7785680137044753701, 40.00000000000002842, -49.23936450072109494 ) ) ;
#9660=CARTESIAN_POINT ( 'NONE',  ( 90.00000000000000000, 24.73819270004212356, -9.108981535246192915E-16 ) ) ;
#9661=CARTESIAN_POINT ( 'NONE',  ( 10.49999999999994138, 42.51666049839543149, 105.0000000000000142 ) ) ;
#9662=CARTESIAN_POINT ( 'NONE',  ( -1.145641935386710886, 0.005153623471255848118, -49.65547338460926596 ) ) ;
#9664=DIRECTION ( 'NONE',  ( -0.000000000000000000, -0.000000000000000000, -1.000000000000000000 ) ) ;
#9666=CARTESIAN_POINT ( 'NONE',  ( 13.25803659942245538, 34.99815359651562119, 58.54720450724165204 ) ) ;
#9669=CARTESIAN_POINT ( 'NONE',  ( 17.41694144196580396, 10.15895996405146029, -59.94253659024143843 ) ) ;
#9671=EDGE_CURVE ( 'NONE', #7701, #8965, #4319, .T. ) ;
#9673=ORIENTED_EDGE ( 'NONE', *, *, #10603, .T. ) ;
#9674=CIRCLE ( 'NONE', #3081, 18.00000000000000000 ) ;
#9677=LINE ( 'NONE', #18622, #12883 ) ;
#9679=CONICAL_SURFACE ( 'NONE', #4919, 58.99999999999994316, 0.7853981633974725929 ) ;
#9683=VERTEX_POINT ( 'NONE', #22431 ) ;
#9686=ORIENTED_EDGE ( 'NONE', *, *, #1484, .T. ) ;
#9687=DIRECTION ( 'NONE',  ( 0.000000000000000000, 0.000000000000000000, -1.000000000000000000 ) ) ;
#9688=CYLINDRICAL_SURFACE ( 'NONE', #21151, 2.099999999999997868 ) ;
#9689=DIRECTION ( 'NONE',  ( -0.000000000000000000, 1.000000000000000000, -0.000000000000000000 ) ) ;
#9690=AXIS2_PLACEMENT_3D ( 'NONE', #19924, #20043, #2633 ) ;
#9691=AXIS2_PLACEMENT_3D ( 'NONE', #1232, #22442, #14972 ) ;
#9692=CARTESIAN_POINT ( 'NONE',  ( -8.188149873056859818, 7.413691783916316780, 42.20917188641860918 ) ) ;
#9697=AXIS2_PLACEMENT_3D ( 'NONE', #5893, #18264, #4178 ) ;
#9698=ORIENTED_EDGE ( 'NONE', *, *, #7664, .F. ) ;
#9699=CARTESIAN_POINT ( 'NONE',  ( -22.38366207802769736, 18.39979965017058916, 58.65857802150431155 ) ) ;
#9703=B_SPLINE_CURVE_WITH_KNOTS ( 'NONE', 3,
 ( #8093, #20351, #2594, #15049, #983, #7976 ),
 .UNSPECIFIED., .F., .F.,
 ( 4, 2, 4 ),
 ( 1.749076889608653681E-18, 0.005389490931282762097, 0.01077898186256552246 ),
 .UNSPECIFIED. ) ;
#9707=FACE_OUTER_BOUND ( 'NONE', #18282, .T. ) ;
#9708=CARTESIAN_POINT ( 'NONE',  ( 6.696867368503558448E-15, 40.00000000000000000, 48.73397172404481381 ) ) ;
#9709=CARTESIAN_POINT ( 'NONE',  ( -9.103081159019573931, 0.03030367950605317509, -53.87333532811887693 ) ) ;
#9710=CARTESIAN_POINT ( 'NONE',  ( -3.171145143956212387, 39.94219471343448191, -51.05053423814366909 ) ) ;
#9711=EDGE_CURVE ( 'NONE', #19741, #13092, #11875, .T. ) ;
#9713=CARTESIAN_POINT ( 'NONE',  ( -9.958219108218488103, 37.43657071496331668, 57.18097912447552034 ) ) ;
#9714=CARTESIAN_POINT ( 'NONE',  ( 15.97698236194076316, 7.938033795521543645, 59.50430813415452036 ) ) ;
#9716=DIRECTION ( 'NONE',  ( -0.000000000000000000, 1.000000000000000000, -0.000000000000000000 ) ) ;
#9717=ORIENTED_EDGE ( 'NONE', *, *, #2607, .F. ) ;
#9719=ORIENTED_EDGE ( 'NONE', *, *, #3252, .T. ) ;
#9720=DIRECTION ( 'NONE',  ( -0.000000000000000000, -1.000000000000000000, -0.000000000000000000 ) ) ;
#9722=VECTOR ( 'NONE', #547, 1000.000000000000000 ) ;
#9724=EDGE_CURVE ( 'NONE', #16, #21800, #13443, .T. ) ;
#9726=CYLINDRICAL_SURFACE ( 'NONE', #12222, 15.00000000000000000 ) ;
#9727=CARTESIAN_POINT ( 'NONE',  ( 6.122947728378624888, 39.99999999999999289, -52.15215614435199143 ) ) ;
#9731=CARTESIAN_POINT ( 'NONE',  ( 0.9019812149625040520, 39.99518069238214224, -49.42305015773394672 ) ) ;
#9736=CARTESIAN_POINT ( 'NONE',  ( -2.478395369818712446, 39.99999999999999289, 50.25195616245800778 ) ) ;
#9737=CARTESIAN_POINT ( 'NONE',  ( 10.74988822578072956, 39.17840323699249439, -54.92437902621830403 ) ) ;
#9738=CYLINDRICAL_SURFACE ( 'NONE', #15541, 2.499999999999998668 ) ;
#9739=CIRCLE ( 'NONE', #10823, 49.99999999999998579 ) ;
#9740=CARTESIAN_POINT ( 'NONE',  ( 42.50000000000000711, -12.00000000000000000, -47.50000000000000000 ) ) ;
#9748=ORIENTED_EDGE ( 'NONE', *, *, #16176, .F. ) ;
#9749=CARTESIAN_POINT ( 'NONE',  ( 35.00000000000000000, 2.142135623730931471, 4.258610482196280173E-15 ) ) ;
#9751=AXIS2_PLACEMENT_3D ( 'NONE', #1119, #21746, #20147 ) ;
#9754=EDGE_LOOP ( 'NONE', ( #6128, #15914, #19210, #388 ) ) ;
#9758=ORIENTED_EDGE ( 'NONE', *, *, #10991, .F. ) ;
#9759=CARTESIAN_POINT ( 'NONE',  ( 16.16773315356744334, 31.81208924699234331, -59.56501305110271716 ) ) ;
#9760=DIRECTION ( 'NONE',  ( 0.000000000000000000, 0.000000000000000000, -1.000000000000000000 ) ) ;
#9763=CARTESIAN_POINT ( 'NONE',  ( 4.985660570713311479, 5.844760174181406143, -40.05045397208984070 ) ) ;
#9764=ORIENTED_EDGE ( 'NONE', *, *, #10743, .T. ) ;
#9769=CARTESIAN_POINT ( 'NONE',  ( -9.855264211176375966, 8.670295722316108566, -43.22210574525156801 ) ) ;
#9771=CARTESIAN_POINT ( 'NONE',  ( -21.01101238435552077, 12.07760467057786080, -58.34718853222887702 ) ) ;
#9775=CARTESIAN_POINT ( 'NONE',  ( 0.7806882667108998586, 39.98538465716379164, -49.65403242876607237 ) ) ;
#9780=ORIENTED_EDGE ( 'NONE', *, *, #17960, .F. ) ;
#9781=CARTESIAN_POINT ( 'NONE',  ( 12.81940492552829980, 35.37234179763579789, 55.76972854553738301 ) ) ;
#9782=CARTESIAN_POINT ( 'NONE',  ( 42.50000000000000711, -12.00000000000000000, -47.50000000000000000 ) ) ;
#9783=CARTESIAN_POINT ( 'NONE',  ( 19.80158170751278135, 22.94611027470399023, -60.57464962002911335 ) ) ;
#9788=ORIENTED_EDGE ( 'NONE', *, *, #16695, .T. ) ;
#9789=EDGE_LOOP ( 'NONE', ( #17663, #13406, #8272, #11359 ) ) ;
#9792=DIRECTION ( 'NONE',  ( -0.000000000000000000, -1.000000000000000000, -0.000000000000000000 ) ) ;
#9802=CARTESIAN_POINT ( 'NONE',  ( 13.56354382738800268, 2.142135623730931471, 56.03997097393685323 ) ) ;
#9806=DIRECTION ( 'NONE',  ( 0.000000000000000000, 0.000000000000000000, 1.000000000000000000 ) ) ;
#9808=CARTESIAN_POINT ( 'NONE',  ( -0.1620518412016254406, 39.99984822781879501, 48.85971577061582138 ) ) ;
#9812=ORIENTED_EDGE ( 'NONE', *, *, #13379, .F. ) ;
#9817=CIRCLE ( 'NONE', #4708, 2.524999999999999467 ) ;
#9818=ORIENTED_EDGE ( 'NONE', *, *, #14065, .F. ) ;
#9819=CARTESIAN_POINT ( 'NONE',  ( -19.66835476178583164, 23.72826198822068022, 58.05955247658096141 ) ) ;
#9820=DIRECTION ( 'NONE',  ( 0.000000000000000000, 0.000000000000000000, -1.000000000000000000 ) ) ;
#9829=CARTESIAN_POINT ( 'NONE',  ( -8.234869854316453797, 38.24532177630956653, -54.56732844084849887 ) ) ;
#9830=CYLINDRICAL_SURFACE ( 'NONE', #15562, 2.499999999999995115 ) ;
#9834=DIRECTION ( 'NONE',  ( -0.000000000000000000, -1.000000000000000000, -0.000000000000000000 ) ) ;
#9836=CARTESIAN_POINT ( 'NONE',  ( -32.90000000000058833, 28.00000000000000000, -55.00000000000076028 ) ) ;
#9838=CONICAL_SURFACE ( 'NONE', #10553, 18.00000000000000000, 0.7853981633974466137 ) ;
#9841=CARTESIAN_POINT ( 'NONE',  ( 34.99999999999980815, 26.00000000000000355, 54.99999999999922551 ) ) ;
#9846=CARTESIAN_POINT ( 'NONE',  ( -0.7280394207210799662, -4.626139448366399343, 46.02403719818684635 ) ) ;
#9851=CARTESIAN_POINT ( 'NONE',  ( 10.34137811700566090, 39.99999999999998579, 53.75702834151141474 ) ) ;
#9852=DIRECTION ( 'NONE',  ( -0.4124789556921616973, 0.7071067811865355823, -0.5743353646704342230 ) ) ;
#9855=CARTESIAN_POINT ( 'NONE',  ( 9.886810796748164876, 39.30595911735670001, -54.61697552245239962 ) ) ;
#9860=CARTESIAN_POINT ( 'NONE',  ( 5.833333333333336590, 40.00000000000000000, 40.61164310337068173 ) ) ;
#9862=CARTESIAN_POINT ( 'NONE',  ( 42.50000000000000711, -12.00000000000000000, -47.50000000000000000 ) ) ;
#9866=ORIENTED_EDGE ( 'NONE', *, *, #9218, .T. ) ;
#9867=EDGE_CURVE ( 'NONE', #15736, #18333, #19673, .T. ) ;
#9870=ORIENTED_EDGE ( 'NONE', *, *, #10957, .F. ) ;
#9871=CARTESIAN_POINT ( 'NONE',  ( 16.44544766657915957, 31.39195386311723723, 59.65016313815161197 ) ) ;
#9873=LINE ( 'NONE', #16750, #21255 ) ;
#9874=CARTESIAN_POINT ( 'NONE',  ( 19.23800698326013148, 14.47374112874265073, 60.43633296823762890 ) ) ;
#9877=DIRECTION ( 'NONE',  ( -0.7071067811865524577, 0.000000000000000000, -0.7071067811865426878 ) ) ;
#9879=EDGE_CURVE ( 'NONE', #14723, #19899, #3972, .T. ) ;
#9880=DIRECTION ( 'NONE',  ( 1.049727191138617217E-16, 0.5150380749100562650, -0.8571673007021111124 ) ) ;
#9881=CARTESIAN_POINT ( 'NONE',  ( -87.90000000000000568, 28.00000000000000000, -9.108981535246192915E-16 ) ) ;
#9883=AXIS2_PLACEMENT_3D ( 'NONE', #449, #17757, #12371 ) ;
#9886=DIRECTION ( 'NONE',  ( -0.000000000000000000, -0.000000000000000000, 1.000000000000000000 ) ) ;
#9888=VERTEX_POINT ( 'NONE', #10600 ) ;
#9890=CARTESIAN_POINT ( 'NONE',  ( -3.315462071040359060, 0.2472509019876770464, -51.08206760068764396 ) ) ;
#9891=ORIENTED_EDGE ( 'NONE', *, *, #4382, .F. ) ;
#9892=CYLINDRICAL_SURFACE ( 'NONE', #5409, 2.499999999999996891 ) ;
#9893=AXIS2_PLACEMENT_3D ( 'NONE', #11022, #7590, #14788 ) ;
#9894=DIRECTION ( 'NONE',  ( -0.000000000000000000, -1.000000000000000000, -0.000000000000000000 ) ) ;
#9895=EDGE_CURVE ( 'NONE', #7376, #20269, #6889, .T. ) ;
#9896=DIRECTION ( 'NONE',  ( 0.000000000000000000, 0.000000000000000000, 1.000000000000000000 ) ) ;
#9897=CARTESIAN_POINT ( 'NONE',  ( 17.29817675750046391, 30.08054145047140082, -57.37022932959450117 ) ) ;
#9898=ORIENTED_EDGE ( 'NONE', *, *, #3809, .F. ) ;
#9901=ORIENTED_EDGE ( 'NONE', *, *, #7936, .T. ) ;
#9902=ORIENTED_EDGE ( 'NONE', *, *, #3987, .T. ) ;
#9908=ORIENTED_EDGE ( 'NONE', *, *, #933, .F. ) ;
#9909=CARTESIAN_POINT ( 'NONE',  ( 90.00000000000000000, 40.00000000000000711, -9.108981535246192915E-16 ) ) ;
#9911=CARTESIAN_POINT ( 'NONE',  ( 5.617773668148541510, 39.81214093377761287, -52.56495119878665889 ) ) ;
#9912=DIRECTION ( 'NONE',  ( -0.7071067811865426878, 8.659560562354874926E-17, 0.7071067811865524577 ) ) ;
#9914=B_SPLINE_CURVE_WITH_KNOTS ( 'NONE', 3,
 ( #8311, #8200, #15164, #9808, #21969, #6259, #16798, #22186, #866, #22309, #13559, #20571, #21851, #6146, #13788, #17234, #20805, #20918, #19312, #17580, #5219, #1665, #3281, #1438, #17349, #6704, #8870, #22653, #15394, #19198, #8646, #22412, #3504, #18854, #6941, #15623, #3160, #13667, #15839, #18974, #11972, #1888, #13902, #153, #21136, #3388, #7147, #1786, #8767, #10129, #10245, #20684, #10465, #1548, #8425, #15507, #5440 ),
 .UNSPECIFIED., .F., .F.,
 ( 4, 2, 1, 1, 1, 2, 2, 2, 1, 1, 1, 2, 2, 2, 1, 1, 1, 2, 2, 2, 1, 1, 1, 1, 2, 2, 2, 1, 1, 1, 1, 1, 1, 2, 2, 2, 2, 4 ),
 ( 0.0001220703125000000000, 0.01574516296385760489, 0.02355670928953641080, 0.02746248245237637234, 0.02941536903379579279, 0.03039181232450494444, 0.03136825561521409261, 0.04699134826655587682, 0.05480289459222675852, 0.05870866775506264346, 0.06066155433648100226, 0.06163799762719056330, 0.06261444091790013822, 0.09386062622063492955, 0.1094837188720028942, 0.1172952651976868488, 0.1212010383605294644, 0.1231539249419507515, 0.1251068115233720524, 0.1875991821288392758, 0.2188453674315729014, 0.2344684600829397003, 0.2422800064086224336, 0.2461857795714643971, 0.2481386661528859616, 0.2500915527343075540, 0.3750762939453137768, 0.4375686645508168882, 0.4688148498535689712, 0.4844379425049449295, 0.4922494888306329641, 0.4961552619934765374, 0.4981081485748984350, 0.4990845918656087732, 0.5000610351563191669, 0.6250457763672394584, 0.7500305175781598610, 1.000000000000000000 ),
 .UNSPECIFIED. ) ;
#9915=CARTESIAN_POINT ( 'NONE',  ( -11.49399598612409079, 36.39311532300400387, -57.83624353974209953 ) ) ;
#9916=ADVANCED_FACE ( 'NONE', ( #12543 ), #14024, .T. ) ;
#9917=CIRCLE ( 'NONE', #32, 2.099999999999997868 ) ;
#9919=CARTESIAN_POINT ( 'NONE',  ( 15.49999999999993783, 42.51666049839543149, 100.0000000000000000 ) ) ;
#9923=ORIENTED_EDGE ( 'NONE', *, *, #20893, .F. ) ;
#9924=CARTESIAN_POINT ( 'NONE',  ( -21.83670385715168649, 14.52494903932916337, 58.53909266577255011 ) ) ;
#9926=CARTESIAN_POINT ( 'NONE',  ( -18.99836266309359800, 13.69920652258249838, -60.37582729383724711 ) ) ;
#9927=DIRECTION ( 'NONE',  ( 0.000000000000000000, 0.000000000000000000, -1.000000000000000000 ) ) ;
#9930=DIRECTION ( 'NONE',  ( -0.000000000000000000, -0.000000000000000000, -1.000000000000000000 ) ) ;
#9932=DIRECTION ( 'NONE',  ( -0.000000000000000000, -1.000000000000000000, -0.000000000000000000 ) ) ;
#9933=AXIS2_PLACEMENT_3D ( 'NONE', #15940, #16062, #19626 ) ;
#9934=EDGE_LOOP ( 'NONE', ( #22143, #2233, #6558 ) ) ;
#9937=ORIENTED_EDGE ( 'NONE', *, *, #18578, .F. ) ;
#9938=CARTESIAN_POINT ( 'NONE',  ( 5.249999999999976907, 40.00000000000000000, -41.42387596543809991 ) ) ;
#9940=DIRECTION ( 'NONE',  ( 0.000000000000000000, -0.000000000000000000, 1.000000000000000000 ) ) ;
#9941=ORIENTED_EDGE ( 'NONE', *, *, #11043, .T. ) ;
#9945=AXIS2_PLACEMENT_3D ( 'NONE', #2648, #8245, #6079 ) ;
#9950=CYLINDRICAL_SURFACE ( 'NONE', #2667, 6.499999999999999112 ) ;
#9951=CARTESIAN_POINT ( 'NONE',  ( -0.7906725175884161683, 39.99999999999998579, 49.24721161524873736 ) ) ;
#9952=CARTESIAN_POINT ( 'NONE',  ( -21.60080777693147169, 26.06115151610113401, -58.48488838346894880 ) ) ;
#9953=CARTESIAN_POINT ( 'NONE',  ( -3.022694720415397995, 39.94544410387499056, 50.94009479445880828 ) ) ;
#9954=DIRECTION ( 'NONE',  ( -0.000000000000000000, -1.000000000000000000, -0.000000000000000000 ) ) ;
#9955=ORIENTED_EDGE ( 'NONE', *, *, #21210, .F. ) ;
#9956=CARTESIAN_POINT ( 'NONE',  ( 12.70473862104218732, 28.00863069209355061, 44.75655646380169372 ) ) ;
#9957=DIRECTION ( 'NONE',  ( -1.000000000000000000, 0.000000000000000000, 0.000000000000000000 ) ) ;
#9960=VECTOR ( 'NONE', #15326, 1000.000000000000000 ) ;
#9961=ORIENTED_EDGE ( 'NONE', *, *, #18915, .F. ) ;
#9962=CARTESIAN_POINT ( 'NONE',  ( -35.00000000000000000, 0.000000000000000000, 1.387778780781445676E-14 ) ) ;
#9965=ADVANCED_FACE ( 'NONE', ( #15986 ), #14258, .F. ) ;
#9969=FACE_OUTER_BOUND ( 'NONE', #2937, .T. ) ;
#9973=DIRECTION ( 'NONE',  ( -0.000000000000000000, 1.000000000000000000, -0.000000000000000000 ) ) ;
#9976=CARTESIAN_POINT ( 'NONE',  ( -34.99999999999980815, 39.97500000000000142, 54.99999999999922551 ) ) ;
#9979=CARTESIAN_POINT ( 'NONE',  ( -6.426802710256914075, 6.431242889908570071, -41.03786381671499583 ) ) ;
#9981=CARTESIAN_POINT ( 'NONE',  ( 1.485717122675836999, -1.299971956346730906, -49.29290837556843030 ) ) ;
#9983=CARTESIAN_POINT ( 'NONE',  ( 6.490531240979301231, 40.00000000000000711, 52.32367557809152459 ) ) ;
#9984=ORIENTED_EDGE ( 'NONE', *, *, #8177, .T. ) ;
#9990=CARTESIAN_POINT ( 'NONE',  ( -42.50000000000000711, -12.00000000000012434, 50.02500000000011937 ) ) ;
#9994=CARTESIAN_POINT ( 'NONE',  ( 22.04638094649235569, 24.21359277922482534, -58.58544938243624500 ) ) ;
#9996=EDGE_CURVE ( 'NONE', #7279, #10478, #5794, .T. ) ;
#10002=EDGE_LOOP ( 'NONE', ( #6873, #11731, #19612, #310 ) ) ;
#10004=DIRECTION ( 'NONE',  ( 0.000000000000000000, 0.000000000000000000, -1.000000000000000000 ) ) ;
#10005=CIRCLE ( 'NONE', #16602, 2.499999999999996891 ) ;
#10007=ORIENTED_EDGE ( 'NONE', *, *, #17772, .F. ) ;
#10009=CARTESIAN_POINT ( 'NONE',  ( -10.27431133777640149, -4.928932188134504955, 51.43682631505699732 ) ) ;
#10016=EDGE_CURVE ( 'NONE', #4461, #15060, #22649, .T. ) ;
#10021=CARTESIAN_POINT ( 'NONE',  ( -14.04383866228955924, 14.71638174774083119, 45.39674436955353087 ) ) ;
#10023=VECTOR ( 'NONE', #7555, 1000.000000000000000 ) ;
#10024=ORIENTED_EDGE ( 'NONE', *, *, #1245, .T. ) ;
#10026=EDGE_CURVE ( 'NONE', #10462, #19879, #15762, .T. ) ;
#10027=VERTEX_POINT ( 'NONE', #21046 ) ;
#10028=CARTESIAN_POINT ( 'NONE',  ( -19.45266119884174216, 15.02268094489439854, 60.49039575452388107 ) ) ;
#10035=CARTESIAN_POINT ( 'NONE',  ( -5.030996294859122919, 39.99999999999999289, -51.62610382703882550 ) ) ;
#10038=CIRCLE ( 'NONE', #160, 60.00000000000000000 ) ;
#10040=CARTESIAN_POINT ( 'NONE',  ( -11.53082054607096829, 39.05546563713489405, 55.22070542825204598 ) ) ;
#10044=CARTESIAN_POINT ( 'NONE',  ( -9.377138775076113930, -4.928932188134509396, -51.00555535510811467 ) ) ;
#10046=ORIENTED_EDGE ( 'NONE', *, *, #17266, .F. ) ;
#10048=VERTEX_POINT ( 'NONE', #16560 ) ;
#10049=VECTOR ( 'NONE', #20990, 1000.000000000000000 ) ;
#10051=DIRECTION ( 'NONE',  ( 1.000000000000000000, 0.000000000000000000, 0.000000000000000000 ) ) ;
#10053=CARTESIAN_POINT ( 'NONE',  ( 7.033428926742908871, 6.687309450572921143, 41.47353357286038289 ) ) ;
#10054=EDGE_CURVE ( 'NONE', #8568, #14085, #18509, .T. ) ;
#10055=CARTESIAN_POINT ( 'NONE',  ( -42.50000000000000711, -12.00000000000000000, 47.50000000000000711 ) ) ;
#10058=CARTESIAN_POINT ( 'NONE',  ( -21.32169069720652033, 26.98977702688068092, -58.42023943869688196 ) ) ;
#10061=CARTESIAN_POINT ( 'NONE',  ( -9.998533603140343118, 40.00000000000000000, 54.54288842742653287 ) ) ;
#10063=CARTESIAN_POINT ( 'NONE',  ( 8.759110511859017123, 32.19698383752734827, 42.56552456877081170 ) ) ;
#10065=CARTESIAN_POINT ( 'NONE',  ( 11.68987541777365458, 3.735186999670053964, -55.40064774139467119 ) ) ;
#10066=DIRECTION ( 'NONE',  ( -1.000000000000000000, 0.000000000000000000, 0.000000000000000000 ) ) ;
#10068=VERTEX_POINT ( 'NONE', #18048 ) ;
#10069=LINE ( 'NONE', #17066, #2121 ) ;
#10077=ORIENTED_EDGE ( 'NONE', *, *, #12013, .T. ) ;
#10078=ORIENTED_EDGE ( 'NONE', *, *, #17016, .T. ) ;
#10079=DIRECTION ( 'NONE',  ( -0.000000000000000000, 1.000000000000000000, -0.000000000000000000 ) ) ;
#10082=DIRECTION ( 'NONE',  ( 0.000000000000000000, -1.000000000000000000, 0.000000000000000000 ) ) ;
#10086=CARTESIAN_POINT ( 'NONE',  ( -17.00000000000002842, 20.00000000000000355, -102.0000000000000142 ) ) ;
#10087=DIRECTION ( 'NONE',  ( 0.000000000000000000, 0.000000000000000000, -1.000000000000000000 ) ) ;
#10088=EDGE_LOOP ( 'NONE', ( #1111, #5226, #19794, #857 ) ) ;
#10091=CARTESIAN_POINT ( 'NONE',  ( 7.325260514639500961E-15, -4.648749848371387827, 45.43309249825157536 ) ) ;
#10094=CARTESIAN_POINT ( 'NONE',  ( 14.98515767422208000, 20.77155976913489610, -45.81928800960650960 ) ) ;
#10095=EDGE_LOOP ( 'NONE', ( #9123, #18658, #7528, #12423, #22493, #18080, #2098 ) ) ;
#10099=CARTESIAN_POINT ( 'NONE',  ( -17.25453130113931621, 34.47978402352275396, 57.33123263757909882 ) ) ;
#10102=AXIS2_PLACEMENT_3D ( 'NONE', #5163, #330, #17629 ) ;
#10106=CARTESIAN_POINT ( 'NONE',  ( 34.99999999999980815, 26.00000000000000355, 52.89999999999922409 ) ) ;
#10109=CARTESIAN_POINT ( 'NONE',  ( 17.11943327291938388, 30.37830191768389199, -59.85657255524078124 ) ) ;
#10110=ORIENTED_EDGE ( 'NONE', *, *, #20136, .T. ) ;
#10114=CARTESIAN_POINT ( 'NONE',  ( -42.50000000000000711, -12.00000000000012434, -50.02500000000011227 ) ) ;
#10116=FACE_OUTER_BOUND ( 'NONE', #2025, .T. ) ;
#10118=VERTEX_POINT ( 'NONE', #641 ) ;
#10119=DIRECTION ( 'NONE',  ( 0.000000000000000000, 0.000000000000000000, 1.000000000000000000 ) ) ;
#10120=CARTESIAN_POINT ( 'NONE',  ( -3.001573872048556968, -1.099462678412693073, -50.31569927527718988 ) ) ;
#10122=AXIS2_PLACEMENT_3D ( 'NONE', #7945, #14906, #6111 ) ;
#10123=VERTEX_POINT ( 'NONE', #9354 ) ;
#10125=CARTESIAN_POINT ( 'NONE',  ( -10.50000000000012079, 42.51666049839536043, 60.00099999999999767 ) ) ;
#10129=CARTESIAN_POINT ( 'NONE',  ( -4.592957628191689068, 39.86863559330478779, 51.95971113232090488 ) ) ;
#10130=CIRCLE ( 'NONE', #13045, 6.499999999999999112 ) ;
#10132=CARTESIAN_POINT ( 'NONE',  ( 8.215393105055619927, 1.749144060402857637, -56.08634520686065628 ) ) ;
#10138=DIRECTION ( 'NONE',  ( -0.000000000000000000, 1.000000000000000000, -0.000000000000000000 ) ) ;
#10139=ADVANCED_FACE ( 'NONE', ( #7633 ), #9688, .F. ) ;
#10141=CARTESIAN_POINT ( 'NONE',  ( 2.180219338269464124, 39.97139182024317705, -50.35380048836591982 ) ) ;
#10147=CARTESIAN_POINT ( 'NONE',  ( -1.679961165565412751, 40.00000000000000000, -49.78369075542040179 ) ) ;
#10148=EDGE_CURVE ( 'NONE', #18353, #15997, #16451, .T. ) ;
#10150=ADVANCED_FACE ( 'NONE', ( #11403 ), #14491, .F. ) ;
#10154=CIRCLE ( 'NONE', #282, 2.524999999999999467 ) ;
#10158=LINE ( 'NONE', #11552, #10763 ) ;
#10163=VERTEX_POINT ( 'NONE', #20126 ) ;
#10165=CARTESIAN_POINT ( 'NONE',  ( -4.859370622531205441, -0.8506459022589687446, 51.48211018323377886 ) ) ;
#10168=EDGE_LOOP ( 'NONE', ( #3462, #124 ) ) ;
#10175=CARTESIAN_POINT ( 'NONE',  ( -19.96400288702121273, 18.50890182901837022, -60.61328093326559951 ) ) ;
#10176=AXIS2_PLACEMENT_3D ( 'NONE', #7445, #10995, #572 ) ;
#10177=CARTESIAN_POINT ( 'NONE',  ( -11.84669267190941078, 29.23061840495883956, -44.31876460048054156 ) ) ;
#10178=CARTESIAN_POINT ( 'NONE',  ( -15.06903587914754716, 33.17837898604023650, 59.20328215072075295 ) ) ;
#10179=VERTEX_POINT ( 'NONE', #2483 ) ;
#10182=DIRECTION ( 'NONE',  ( 0.000000000000000000, 1.000000000000000000, 0.000000000000000000 ) ) ;
#10184=EDGE_LOOP ( 'NONE', ( #13513, #1647, #17636, #16402 ) ) ;
#10185=EDGE_CURVE ( 'NONE', #938, #12299, #14713, .T. ) ;
#10186=AXIS2_PLACEMENT_3D ( 'NONE', #19554, #4088, #296 ) ;
#10187=CARTESIAN_POINT ( 'NONE',  ( -35.00000000000000000, 40.00000000000000000, -58.99999999999992895 ) ) ;
#10192=( GEOMETRIC_REPRESENTATION_CONTEXT ( 3 ) GLOBAL_UNCERTAINTY_ASSIGNED_CONTEXT ( ( #11499 ) ) GLOBAL_UNIT_ASSIGNED_CONTEXT ( ( #15604, #22632, #22292 ) ) REPRESENTATION_CONTEXT ( 'NONE', 'WORKASPACE' ) );
#10193=VERTEX_POINT ( 'NONE', #17119 ) ;
#10196=CYLINDRICAL_SURFACE ( 'NONE', #1524, 2.499999999999998668 ) ;
#10197=CARTESIAN_POINT ( 'NONE',  ( 4.026578693517047114, -4.679980696195654488, 48.24134193083390443 ) ) ;
#10203=CARTESIAN_POINT ( 'NONE',  ( -11.51554440985547956, 40.00000000000000711, -54.14601575511822773 ) ) ;
#10204=VECTOR ( 'NONE', #15014, 1000.000000000000000 ) ;
#10208=EDGE_CURVE ( 'NONE', #9032, #3941, #6594, .T. ) ;
#10209=FACE_BOUND ( 'NONE', #10722, .T. ) ;
#10211=ORIENTED_EDGE ( 'NONE', *, *, #14707, .T. ) ;
#10212=FACE_OUTER_BOUND ( 'NONE', #13412, .T. ) ;
#10215=CARTESIAN_POINT ( 'NONE',  ( -22.25047517524403062, 22.91581175091617695, 58.62998360803281628 ) ) ;
#10220=LINE ( 'NONE', #7019, #11463 ) ;
#10225=ORIENTED_EDGE ( 'NONE', *, *, #17511, .F. ) ;
#10228=ORIENTED_EDGE ( 'NONE', *, *, #14810, .T. ) ;
#10231=CARTESIAN_POINT ( 'NONE',  ( 9.064501325224163963, 40.00000000000000711, -53.36141974371220442 ) ) ;
#10234=CARTESIAN_POINT ( 'NONE',  ( -1.061447036142183720, 5.028531101166970885, 38.77662560222201904 ) ) ;
#10236=CARTESIAN_POINT ( 'NONE',  ( -9.103081159019536628, 0.03030367950604325594, 53.87333532811888404 ) ) ;
#10237=EDGE_CURVE ( 'NONE', #7020, #6550, #20058, .T. ) ;
#10239=AXIS2_PLACEMENT_3D ( 'NONE', #3414, #14264, #12439 ) ;
#10240=CARTESIAN_POINT ( 'NONE',  ( 42.50000000000000711, -12.00000000000000000, -49.60000000000000142 ) ) ;
#10243=CARTESIAN_POINT ( 'NONE',  ( 35.00000000000000000, -4.928932188134504955, 4.258610482196280173E-15 ) ) ;
#10245=CARTESIAN_POINT ( 'NONE',  ( -5.178708363027197947, 39.83382011705033676, 52.32443608441192850 ) ) ;
#10249=EDGE_CURVE ( 'NONE', #3928, #12420, #3158, .T. ) ;
#10252=ORIENTED_EDGE ( 'NONE', *, *, #2324, .F. ) ;
#10254=ORIENTED_EDGE ( 'NONE', *, *, #19838, .F. ) ;
#10255=CARTESIAN_POINT ( 'NONE',  ( -11.68090480754633376, 3.765577839755392286, 57.90797000640143466 ) ) ;
#10260=CARTESIAN_POINT ( 'NONE',  ( 35.00000000000000000, 39.00000000000000711, 4.258610482196280173E-15 ) ) ;
#10261=EDGE_CURVE ( 'NONE', #11720, #15580, #13453, .T. ) ;
#10266=FACE_OUTER_BOUND ( 'NONE', #12981, .T. ) ;
#10269=CARTESIAN_POINT ( 'NONE',  ( -13.28791054760751322, 34.95496542652811200, 58.55506233662532622 ) ) ;
#10270=ORIENTED_EDGE ( 'NONE', *, *, #5695, .T. ) ;
#10272=DIRECTION ( 'NONE',  ( -0.5840452403773163104, -0.8117211080122302969, 0.000000000000000000 ) ) ;
#10273=EDGE_CURVE ( 'NONE', #3905, #675, #18969, .T. ) ;
#10276=ORIENTED_EDGE ( 'NONE', *, *, #10683, .F. ) ;
#10278=ORIENTED_EDGE ( 'NONE', *, *, #11112, .T. ) ;
#10286=CARTESIAN_POINT ( 'NONE',  ( -19.94270148199918680, 21.57319560958785232, -58.13234078200304822 ) ) ;
#10288=EDGE_LOOP ( 'NONE', ( #16784, #13826, #4331, #9613 ) ) ;
#10290=FACE_BOUND ( 'NONE', #8462, .T. ) ;
#10295=ADVANCED_FACE ( 'NONE', ( #22184 ), #20075, .F. ) ;
#10306=ADVANCED_FACE ( 'NONE', ( #8198 ), #8356, .T. ) ;
#10307=DIRECTION ( 'NONE',  ( 1.000000000000000000, 0.000000000000000000, 0.000000000000000000 ) ) ;
#10308=ORIENTED_EDGE ( 'NONE', *, *, #13457, .T. ) ;
#10309=CARTESIAN_POINT ( 'NONE',  ( 34.99999999999980815, 26.00000000000000355, 57.09999999999921982 ) ) ;
#10310=CARTESIAN_POINT ( 'NONE',  ( -10.45842016914155259, 40.00000000000001421, -53.79442460303518203 ) ) ;
#10312=DIRECTION ( 'NONE',  ( 0.4124789556921606426, 0.7071067811865359154, -0.5743353646704345561 ) ) ;
#10313=DIRECTION ( 'NONE',  ( 0.000000000000000000, -1.000000000000000000, 0.000000000000000000 ) ) ;
#10314=CARTESIAN_POINT ( 'NONE',  ( -35.00000000000000000, -5.000000000000000888, 18.00000000000001421 ) ) ;
#10315=CARTESIAN_POINT ( 'NONE',  ( 0.7351295361033751696, 39.99998559611954363, 49.30628084492604302 ) ) ;
#10316=CARTESIAN_POINT ( 'NONE',  ( 8.759110511859015347, 32.19698383752734827, -42.56552456877079038 ) ) ;
#10318=EDGE_LOOP ( 'NONE', ( #16959, #15403, #18650 ) ) ;
#10322=CARTESIAN_POINT ( 'NONE',  ( -42.50000000000000711, -12.00000000000000000, 41.00000000000000711 ) ) ;
#10325=VERTEX_POINT ( 'NONE', #17006 ) ;
#10330=DIRECTION ( 'NONE',  ( 0.000000000000000000, -0.000000000000000000, -1.000000000000000000 ) ) ;
#10331=VECTOR ( 'NONE', #17466, 1000.000000000000000 ) ;
#10333=VERTEX_POINT ( 'NONE', #9411 ) ;
#10335=CARTESIAN_POINT ( 'NONE',  ( 21.01101238435548879, 12.07760467057785370, 58.34718853222888413 ) ) ;
#10339=DIRECTION ( 'NONE',  ( -0.000000000000000000, 1.000000000000000000, -0.000000000000000000 ) ) ;
#10344=ORIENTED_EDGE ( 'NONE', *, *, #3992, .T. ) ;
#10349=CARTESIAN_POINT ( 'NONE',  ( 16.49514046905077436, 8.656442121910195908, 59.66722042020315797 ) ) ;
#10353=EDGE_CURVE ( 'NONE', #18007, #13854, #7268, .T. ) ;
#10355=ORIENTED_EDGE ( 'NONE', *, *, #20821, .F. ) ;
#10356=EDGE_CURVE ( 'NONE', #2703, #1700, #4197, .T. ) ;
#10358=ORIENTED_EDGE ( 'NONE', *, *, #9179, .F. ) ;
#10359=ORIENTED_EDGE ( 'NONE', *, *, #16714, .T. ) ;
#10360=FACE_OUTER_BOUND ( 'NONE', #17131, .T. ) ;
#10362=B_SPLINE_SURFACE_WITH_KNOTS ( 'NONE', 1, 3, ( 
 ( #6190, #9851, #16720, #21773, #2410, #9615 ),
 ( #5846, #14649, #21893, #16493, #6070, #13036 ) ),
 .UNSPECIFIED., .F., .F., .F.,
 ( 2, 2 ),
 ( 4, 2, 4 ),
 ( 0.000000000000000000, 1.000000000000000000 ),
 ( 0.000000000000000000, 0.001214050925800256708, 0.002428101851600513415 ),
 .UNSPECIFIED. ) ;
#10363=AXIS2_PLACEMENT_3D ( 'NONE', #2849, #9834, #13137 ) ;
#10364=AXIS2_PLACEMENT_3D ( 'NONE', #16618, #926, #16391 ) ;
#10366=CARTESIAN_POINT ( 'NONE',  ( -90.00000000000000000, 26.00000000000000355, -2.099999999999991651 ) ) ;
#10367=CARTESIAN_POINT ( 'NONE',  ( 2.175252786020501983, 39.97152392022739775, 50.35028940454238011 ) ) ;
#10371=DIRECTION ( 'NONE',  ( -0.000000000000000000, -1.000000000000000000, -0.000000000000000000 ) ) ;
#10373=DIRECTION ( 'NONE',  ( -0.000000000000000000, -0.000000000000000000, 1.000000000000000000 ) ) ;
#10375=CARTESIAN_POINT ( 'NONE',  ( -19.92971843794357056, 21.94076660514457089, 60.60536071356336407 ) ) ;
#10379=CARTESIAN_POINT ( 'NONE',  ( -8.331955809010665348, 38.18181818181817277, 56.36098470834075158 ) ) ;
#10380=CARTESIAN_POINT ( 'NONE',  ( -35.00000000000000000, 2.142135623730931471, 1.387778780781445676E-14 ) ) ;
#10384=ADVANCED_FACE ( 'NONE', ( #239 ), #15110, .F. ) ;
#10385=ORIENTED_EDGE ( 'NONE', *, *, #11936, .T. ) ;
#10386=ORIENTED_EDGE ( 'NONE', *, *, #5057, .F. ) ;
#10387=CARTESIAN_POINT ( 'NONE',  ( 2.066061548970023143, -1.174227811084479489, -49.70141618117591520 ) ) ;
#10389=VERTEX_POINT ( 'NONE', #9294 ) ;
#10394=CARTESIAN_POINT ( 'NONE',  ( -22.38103533145807944, 18.35979201191610244, -58.65801380639353368 ) ) ;
#10395=CIRCLE ( 'NONE', #12239, 57.00000000000002132 ) ;
#10397=ORIENTED_EDGE ( 'NONE', *, *, #1668, .T. ) ;
#10398=DIRECTION ( 'NONE',  ( 0.000000000000000000, 0.000000000000000000, 1.000000000000000000 ) ) ;
#10400=DIRECTION ( 'NONE',  ( 0.000000000000000000, 0.000000000000000000, 1.000000000000000000 ) ) ;
#10401=EDGE_CURVE ( 'NONE', #922, #16909, #12596, .T. ) ;
#10402=EDGE_CURVE ( 'NONE', #1538, #1187, #14409, .T. ) ;
#10407=FACE_OUTER_BOUND ( 'NONE', #1906, .T. ) ;
#10414=CARTESIAN_POINT ( 'NONE',  ( 42.50000000000000711, -12.00000000000000000, 47.50000000000000711 ) ) ;
#10416=AXIS2_PLACEMENT_3D ( 'NONE', #10759, #12591, #19275 ) ;
#10418=EDGE_CURVE ( 'NONE', #11348, #21191, #18079, .T. ) ;
#10419=CARTESIAN_POINT ( 'NONE',  ( 11.86180952233169705, 39.00000000000000000, 55.35904751184887118 ) ) ;
#10422=CARTESIAN_POINT ( 'NONE',  ( -9.952189117650851458, 40.00000000000000000, -53.64426396172072486 ) ) ;
#10423=ORIENTED_EDGE ( 'NONE', *, *, #3335, .F. ) ;
#10424=CARTESIAN_POINT ( 'NONE',  ( 5.816608766684120191, -4.770324936805535820, -49.23968220743348922 ) ) ;
#10425=CARTESIAN_POINT ( 'NONE',  ( 13.56354382738798847, 2.142135623730931471, -56.03997097393683191 ) ) ;
#10427=DIRECTION ( 'NONE',  ( 0.000000000000000000, 0.000000000000000000, 1.000000000000000000 ) ) ;
#10429=CARTESIAN_POINT ( 'NONE',  ( 14.99999999999998579, 20.00000000000000355, -45.82575694955836809 ) ) ;
#10431=DIRECTION ( 'NONE',  ( 1.000000000000000000, 0.000000000000000000, 0.000000000000000000 ) ) ;
#10434=CARTESIAN_POINT ( 'NONE',  ( -17.14099744770040701, 5.493236686326245177, 57.28126710884286155 ) ) ;
#10435=VERTEX_POINT ( 'NONE', #6082 ) ;
#10437=DIRECTION ( 'NONE',  ( -0.000000000000000000, -0.000000000000000000, -1.000000000000000000 ) ) ;
#10441=EDGE_CURVE ( 'NONE', #10027, #8509, #19199, .T. ) ;
#10445=ORIENTED_EDGE ( 'NONE', *, *, #10185, .T. ) ;
#10448=DIRECTION ( 'NONE',  ( 1.776356839400250070E-15, 0.000000000000000000, 1.000000000000000000 ) ) ;
#10450=CARTESIAN_POINT ( 'NONE',  ( 9.100109602677072473, 40.00000000000000000, 53.37249912551077102 ) ) ;
#10452=LINE ( 'NONE', #1428, #2508 ) ;
#10453=CARTESIAN_POINT ( 'NONE',  ( -2.859979007343815383, 5.272989970146413796, 39.14811524457574166 ) ) ;
#10454=ORIENTED_EDGE ( 'NONE', *, *, #14532, .F. ) ;
#10455=AXIS2_PLACEMENT_3D ( 'NONE', #18527, #487, #10670 ) ;
#10456=FACE_OUTER_BOUND ( 'NONE', #21467, .T. ) ;
#10458=CARTESIAN_POINT ( 'NONE',  ( 6.889846921705527817E-15, -1.896945173645837590, 47.89158637319812328 ) ) ;
#10460=ORIENTED_EDGE ( 'NONE', *, *, #9212, .F. ) ;
#10461=CARTESIAN_POINT ( 'NONE',  ( 2.859979007343827817, 34.72701002985358087, 39.14811524457574876 ) ) ;
#10462=VERTEX_POINT ( 'NONE', #18448 ) ;
#10465=CARTESIAN_POINT ( 'NONE',  ( -6.745305152897880241, 39.70676899211738942, 53.21562672405194405 ) ) ;
#10466=CONICAL_SURFACE ( 'NONE', #6461, 49.99999999999998579, 0.7853981633974691512 ) ;
#10467=PLANE ( 'NONE',  #6037 ) ;
#10475=ORIENTED_EDGE ( 'NONE', *, *, #13576, .F. ) ;
#10478=VERTEX_POINT ( 'NONE', #9626 ) ;
#10479=CARTESIAN_POINT ( 'NONE',  ( -15.00671337312635067, 3.288799316214447988, 56.57538198732753898 ) ) ;
#10482=CARTESIAN_POINT ( 'NONE',  ( -35.00000000000000000, 39.00000000000000711, -49.99999999999997158 ) ) ;
#10483=CARTESIAN_POINT ( 'NONE',  ( 0.08083351145619603606, 39.99996233019618330, 48.79679892491352433 ) ) ;
#10485=DIRECTION ( 'NONE',  ( 0.000000000000000000, 0.000000000000000000, -1.000000000000000000 ) ) ;
#10486=CYLINDRICAL_SURFACE ( 'NONE', #19258, 2.500000000000002220 ) ;
#10487=DIRECTION ( 'NONE',  ( 0.000000000000000000, 0.000000000000000000, 1.000000000000000000 ) ) ;
#10492=ORIENTED_EDGE ( 'NONE', *, *, #22039, .T. ) ;
#10494=CARTESIAN_POINT ( 'NONE',  ( -7.938322399564284204, 38.36220367130332676, 56.16250688144528169 ) ) ;
#10495=DIRECTION ( 'NONE',  ( -0.000000000000000000, 1.000000000000000000, -0.000000000000000000 ) ) ;
#10497=EDGE_LOOP ( 'NONE', ( #18057, #4027, #4048 ) ) ;
#10501=EDGE_LOOP ( 'NONE', ( #2649, #15089, #22393 ) ) ;
#10502=CARTESIAN_POINT ( 'NONE',  ( -0.05567163769003378310, -4.650449146058907246, -45.38800358221576658 ) ) ;
#10508=CARTESIAN_POINT ( 'NONE',  ( 15.99999999999991651, 20.00000000000000000, 102.0000000000000142 ) ) ;
#10510=CARTESIAN_POINT ( 'NONE',  ( -12.50843255120859965, 35.62740313860118135, -55.64392373821144133 ) ) ;
#10514=EDGE_LOOP ( 'NONE', ( #14035, #4916 ) ) ;
#10515=CARTESIAN_POINT ( 'NONE',  ( 42.50000000000000711, -11.97499999999999964, -45.00000000000000000 ) ) ;
#10517=FACE_BOUND ( 'NONE', #22548, .T. ) ;
#10518=CARTESIAN_POINT ( 'NONE',  ( 35.00000000000000711, 40.00000000000000000, -51.00000000000001421 ) ) ;
#10519=PLANE ( 'NONE',  #1596 ) ;
#10520=CIRCLE ( 'NONE', #20781, 49.99999999999998579 ) ;
#10524=EDGE_CURVE ( 'NONE', #19371, #14798, #18566, .T. ) ;
#10530=VECTOR ( 'NONE', #16522, 1000.000000000000000 ) ;
#10531=ORIENTED_EDGE ( 'NONE', *, *, #16678, .F. ) ;
#10532=CYLINDRICAL_SURFACE ( 'NONE', #14242, 15.00000000000000000 ) ;
#10534=DIRECTION ( 'NONE',  ( -0.000000000000000000, 1.000000000000000000, -0.000000000000000000 ) ) ;
#10537=CARTESIAN_POINT ( 'NONE',  ( -10.79056263833820850, 39.99999999999999289, -53.90082266129228827 ) ) ;
#10540=CARTESIAN_POINT ( 'NONE',  ( 22.08212374814979384, 16.07286297122273311, -58.59297470305927646 ) ) ;
#10542=CARTESIAN_POINT ( 'NONE',  ( -6.217947036537184502, 39.75326280012639302, -52.92450753908158845 ) ) ;
#10543=AXIS2_PLACEMENT_3D ( 'NONE', #19218, #22429, #15525 ) ;
#10546=CARTESIAN_POINT ( 'NONE',  ( -22.08212374814983292, 16.07286297122275798, 58.59297470305928357 ) ) ;
#10549=CARTESIAN_POINT ( 'NONE',  ( 11.05758567242883572, 3.294696707135831737, 55.18338768059803812 ) ) ;
#10550=AXIS2_PLACEMENT_3D ( 'NONE', #18430, #20050, #21651 ) ;
#10553=AXIS2_PLACEMENT_3D ( 'NONE', #21095, #2180, #17984 ) ;
#10554=EDGE_CURVE ( 'NONE', #5122, #164, #16849, .T. ) ;
#10559=CIRCLE ( 'NONE', #22311, 60.00000000000000000 ) ;
#10561=EDGE_CURVE ( 'NONE', #5921, #4421, #1269, .T. ) ;
#10565=CARTESIAN_POINT ( 'NONE',  ( 35.00000000000000000, 39.00000000000000711, -49.99999999999997868 ) ) ;
#10566=DIRECTION ( 'NONE',  ( -0.000000000000000000, -1.000000000000000000, -0.000000000000000000 ) ) ;
#10569=CARTESIAN_POINT ( 'NONE',  ( -1.387778780781445518E-14, 20.00000000000000355, -100.0000000000000000 ) ) ;
#10571=EDGE_LOOP ( 'NONE', ( #16445, #1299, #14801, #12795, #1449 ) ) ;
#10574=CARTESIAN_POINT ( 'NONE',  ( -13.67681338760606735, 37.77871559274755953, -56.08437820317177369 ) ) ;
#10575=ORIENTED_EDGE ( 'NONE', *, *, #14311, .T. ) ;
#10578=FACE_OUTER_BOUND ( 'NONE', #9182, .T. ) ;
#10580=CYLINDRICAL_SURFACE ( 'NONE', #13374, 10.00000000000000178 ) ;
#10582=ADVANCED_FACE ( 'NONE', ( #8366, #4819, #10290, #3439, #13602, #15336, #10517, #19023 ), #15558, .T. ) ;
#10583=CARTESIAN_POINT ( 'NONE',  ( 18.96886095803687056, 26.35434275172393015, 60.36758075326454787 ) ) ;
#10584=DIRECTION ( 'NONE',  ( -0.000000000000000000, -0.000000000000000000, 1.000000000000000000 ) ) ;
#10594=CARTESIAN_POINT ( 'NONE',  ( 0.3971958550642871177, 39.99908967365433199, 49.04071034064279644 ) ) ;
#10595=ADVANCED_FACE ( 'NONE', ( #15784 ), #11503, .F. ) ;
#10597=ORIENTED_EDGE ( 'NONE', *, *, #14276, .T. ) ;
#10598=CARTESIAN_POINT ( 'NONE',  ( -90.00000000000000000, 26.00000000000000355, -9.108981535246192915E-16 ) ) ;
#10599=DIRECTION ( 'NONE',  ( -0.000000000000000000, 1.000000000000000000, -0.000000000000000000 ) ) ;
#10600=CARTESIAN_POINT ( 'NONE',  ( -9.103081159019573931, 0.03030367950605317509, -53.87333532811887693 ) ) ;
#10603=EDGE_CURVE ( 'NONE', #14814, #11530, #14404, .T. ) ;
#10604=CARTESIAN_POINT ( 'NONE',  ( -11.50056215611671107, 36.46966885432792083, 57.85578624339548526 ) ) ;
#10608=ORIENTED_EDGE ( 'NONE', *, *, #9895, .F. ) ;
#10613=DIRECTION ( 'NONE',  ( 0.000000000000000000, 0.000000000000000000, 1.000000000000000000 ) ) ;
#10616=CARTESIAN_POINT ( 'NONE',  ( 9.103081159015154356, 0.03030367950454006254, 53.87333532811640424 ) ) ;
#10622=CYLINDRICAL_SURFACE ( 'NONE', #5127, 2.499999999999998668 ) ;
#10624=DIRECTION ( 'NONE',  ( 0.000000000000000000, 0.000000000000000000, 1.000000000000000000 ) ) ;
#10625=CARTESIAN_POINT ( 'NONE',  ( 13.07600923154788219, 12.64060470162861272, -44.93756990742566160 ) ) ;
#10626=ORIENTED_EDGE ( 'NONE', *, *, #12117, .F. ) ;
#10628=CARTESIAN_POINT ( 'NONE',  ( -34.99999999999980815, 40.00000000000000000, 57.49999999999921840 ) ) ;
#10630=EDGE_CURVE ( 'NONE', #21858, #1751, #20616, .T. ) ;
#10633=AXIS2_PLACEMENT_3D ( 'NONE', #2837, #18870, #13230 ) ;
#10636=DIRECTION ( 'NONE',  ( 0.000000000000000000, 0.000000000000000000, -1.000000000000000000 ) ) ;
#10641=ORIENTED_EDGE ( 'NONE', *, *, #21221, .T. ) ;
#10643=CARTESIAN_POINT ( 'NONE',  ( 19.90072640592957853, 9.610007367499614261, -58.06946678856479593 ) ) ;
#10645=CARTESIAN_POINT ( 'NONE',  ( -12.24744603029287937, 40.00000000000000000, -54.43639671998464991 ) ) ;
#10647=DIRECTION ( 'NONE',  ( -0.000000000000000000, 1.000000000000000000, -0.000000000000000000 ) ) ;
#10648=CARTESIAN_POINT ( 'NONE',  ( -10.62139969368297443, 0.6004703193305642728, 54.70636795414677778 ) ) ;
#10649=CARTESIAN_POINT ( 'NONE',  ( -4.573707352612297328, 39.86977586383432737, -51.94771487799405918 ) ) ;
#10651=CIRCLE ( 'NONE', #16530, 10.00000000000000178 ) ;
#10661=LINE ( 'NONE', #7250, #15039 ) ;
#10663=CARTESIAN_POINT ( 'NONE',  ( 4.198144980488468292, 39.89210059029527855, -51.71386871416487452 ) ) ;
#10664=CARTESIAN_POINT ( 'NONE',  ( 6.607276003051461011, 39.99999999999998579, 52.37472748948959378 ) ) ;
#10665=ORIENTED_EDGE ( 'NONE', *, *, #17326, .F. ) ;
#10666=DIRECTION ( 'NONE',  ( 0.000000000000000000, -1.000000000000000000, 0.000000000000000000 ) ) ;
#10667=CARTESIAN_POINT ( 'NONE',  ( -3.174475770749913828, -4.645331003331745201, -47.72510079650425752 ) ) ;
#10670=DIRECTION ( 'NONE',  ( 0.000000000000000000, -0.000000000000000000, 1.000000000000000000 ) ) ;
#10673=ADVANCED_FACE ( 'NONE', ( #12356, #19579, #4008, #7200, #8917, #4112, #3890, #550 ), #15893, .F. ) ;
#10674=CARTESIAN_POINT ( 'NONE',  ( 6.094635461695178336, 0.8905127700715224082, 54.73853566233531609 ) ) ;
#10676=CARTESIAN_POINT ( 'NONE',  ( 3.244689583147984280, 39.74755540027143752, -52.34195286441637052 ) ) ;
#10677=CARTESIAN_POINT ( 'NONE',  ( -1.255208329926627453, 39.96308463907305253, 50.19868133818723521 ) ) ;
#10680=CARTESIAN_POINT ( 'NONE',  ( 8.835435312963896948, 40.00000000000000000, -53.27933556908502766 ) ) ;
#10681=CARTESIAN_POINT ( 'NONE',  ( 20.00424115936584712, 19.83711385861052889, 60.62278039730742307 ) ) ;
#10683=EDGE_CURVE ( 'NONE', #862, #6172, #16257, .T. ) ;
#10684=EDGE_CURVE ( 'NONE', #10193, #15500, #19368, .T. ) ;
#10686=VECTOR ( 'NONE', #7620, 1000.000000000000000 ) ;
#10691=EDGE_CURVE ( 'NONE', #13427, #11968, #2313, .T. ) ;
#10696=DIRECTION ( 'NONE',  ( 0.8171172023792293571, 0.3308262969263032760, -0.4720947350246252339 ) ) ;
#10698=CARTESIAN_POINT ( 'NONE',  ( -35.00000000000058265, 40.00000000000000711, -52.47500000000076170 ) ) ;
#10700=CARTESIAN_POINT ( 'NONE',  ( 0.2316811374357567177, 39.99968400796328893, 48.91347626078281507 ) ) ;
#10701=B_SPLINE_CURVE_WITH_KNOTS ( 'NONE', 3,
 ( #14143, #5466, #3751, #7521, #14260, #2364 ),
 .UNSPECIFIED., .F., .F.,
 ( 4, 2, 4 ),
 ( 0.000000000000000000, 0.002641318319677474300, 0.005282636639354948600 ),
 .UNSPECIFIED. ) ;
#10704=EDGE_CURVE ( 'NONE', #8676, #21259, #6394, .T. ) ;
#10705=VERTEX_POINT ( 'NONE', #12457 ) ;
#10708=DIRECTION ( 'NONE',  ( 0.000000000000000000, 1.000000000000000000, 0.000000000000000000 ) ) ;
#10709=DIRECTION ( 'NONE',  ( 0.000000000000000000, 0.000000000000000000, -1.000000000000000000 ) ) ;
#10710=VECTOR ( 'NONE', #20777, 1000.000000000000000 ) ;
#10713=CARTESIAN_POINT ( 'NONE',  ( -1.387778780781445676E-14, 20.00000000000000000, -105.0020000000000095 ) ) ;
#10715=EDGE_CURVE ( 'NONE', #5289, #14267, #14284, .T. ) ;
#10717=VECTOR ( 'NONE', #15038, 1000.000000000000000 ) ;
#10720=AXIS2_PLACEMENT_3D ( 'NONE', #8368, #6990, #22356 ) ;
#10722=EDGE_LOOP ( 'NONE', ( #18896, #9923 ) ) ;
#10723=CARTESIAN_POINT ( 'NONE',  ( 3.309563215936520475, -3.140776953251411374, -49.61090469809367676 ) ) ;
#10728=AXIS2_PLACEMENT_3D ( 'NONE', #12998, #20017, #11300 ) ;
#10729=DIRECTION ( 'NONE',  ( -0.5840452403773163104, 0.8117211080122304079, 0.000000000000000000 ) ) ;
#10730=DIRECTION ( 'NONE',  ( -0.000000000000000000, -0.000000000000000000, -1.000000000000000000 ) ) ;
#10736=AXIS2_PLACEMENT_3D ( 'NONE', #18311, #21877, #2629 ) ;
#10737=DIRECTION ( 'NONE',  ( 0.000000000000000000, 0.000000000000000000, -1.000000000000000000 ) ) ;
#10738=DIRECTION ( 'NONE',  ( 0.000000000000000000, -1.000000000000000000, 0.000000000000000000 ) ) ;
#10742=CARTESIAN_POINT ( 'NONE',  ( -12.99999999999980282, -2.516660498395516310, -105.0000000000000142 ) ) ;
#10743=EDGE_CURVE ( 'NONE', #3040, #1608, #10395, .T. ) ;
#10744=CARTESIAN_POINT ( 'NONE',  ( 16.35275686153459063, 4.590993025984193565, -57.03319805596824921 ) ) ;
#10746=VERTEX_POINT ( 'NONE', #9328 ) ;
#10749=VERTEX_POINT ( 'NONE', #12415 ) ;
#10750=CARTESIAN_POINT ( 'NONE',  ( -90.00000000000000000, 40.00000000000000000, -9.108981535246192915E-16 ) ) ;
#10753=VERTEX_POINT ( 'NONE', #2224 ) ;
#10759=CARTESIAN_POINT ( 'NONE',  ( -35.00000000000000000, 38.99999999999999289, 1.387778780781445676E-14 ) ) ;
#10762=DIRECTION ( 'NONE',  ( -1.000000000000000000, 0.000000000000000000, 0.000000000000000000 ) ) ;
#10763=VECTOR ( 'NONE', #6510, 1000.000000000000000 ) ;
#10765=CARTESIAN_POINT ( 'NONE',  ( -1.103251808850783888, 39.99275656215084496, -49.57314659356683251 ) ) ;
#10772=VECTOR ( 'NONE', #14804, 1000.000000000000000 ) ;
#10773=ORIENTED_EDGE ( 'NONE', *, *, #5478, .F. ) ;
#10777=B_SPLINE_CURVE_WITH_KNOTS ( 'NONE', 3,
 ( #19888, #4199, #18171, #9471 ),
 .UNSPECIFIED., .F., .F.,
 ( 4, 4 ),
 ( 0.000000000000000000, 1.000000000000000000 ),
 .UNSPECIFIED. ) ;
#10780=FACE_OUTER_BOUND ( 'NONE', #1005, .T. ) ;
#10784=CARTESIAN_POINT ( 'NONE',  ( 1.571409433144389078, 40.00000000000000711, -49.72695173164139959 ) ) ;
#10785=CARTESIAN_POINT ( 'NONE',  ( 9.519381200825437261, 39.99999999999999289, 53.51361895441421979 ) ) ;
#10787=DIRECTION ( 'NONE',  ( -0.000000000000000000, -1.000000000000000000, -0.000000000000000000 ) ) ;
#10789=ORIENTED_EDGE ( 'NONE', *, *, #15067, .F. ) ;
#10791=ADVANCED_FACE ( 'NONE', ( #7493 ), #12754, .T. ) ;
#10798=VECTOR ( 'NONE', #11946, 1000.000000000000000 ) ;
#10800=CARTESIAN_POINT ( 'NONE',  ( 42.50000000000000711, -11.97499999999999964, -50.00000000000000000 ) ) ;
#10805=CARTESIAN_POINT ( 'NONE',  ( 18.56336306567978411, 12.50537704746338541, 60.26262883998656150 ) ) ;
#10806=CARTESIAN_POINT ( 'NONE',  ( -12.99999999999980282, -2.516660498395516310, 60.00099999999999767 ) ) ;
#10810=ORIENTED_EDGE ( 'NONE', *, *, #5568, .T. ) ;
#10811=EDGE_CURVE ( 'NONE', #11727, #16638, #6753, .T. ) ;
#10814=AXIS2_PLACEMENT_3D ( 'NONE', #16450, #759, #14712 ) ;
#10818=CIRCLE ( 'NONE', #15193, 2.099999999999997868 ) ;
#10823=AXIS2_PLACEMENT_3D ( 'NONE', #20158, #11333, #14746 ) ;
#10826=DIRECTION ( 'NONE',  ( 0.000000000000000000, 1.000000000000000000, 0.000000000000000000 ) ) ;
#10828=DIRECTION ( 'NONE',  ( 0.000000000000000000, 0.000000000000000000, -1.000000000000000000 ) ) ;
#10829=LINE ( 'NONE', #12884, #13509 ) ;
#10831=VECTOR ( 'NONE', #2502, 1000.000000000000000 ) ;
#10834=CIRCLE ( 'NONE', #221, 2.000000000000001776 ) ;
#10836=CARTESIAN_POINT ( 'NONE',  ( 11.86180952234342278, 38.99999999999291589, -55.35904751185374550 ) ) ;
#10839=ORIENTED_EDGE ( 'NONE', *, *, #6806, .F. ) ;
#10840=EDGE_CURVE ( 'NONE', #6249, #14950, #8666, .T. ) ;
#10841=ORIENTED_EDGE ( 'NONE', *, *, #13589, .T. ) ;
#10842=CARTESIAN_POINT ( 'NONE',  ( -34.99999999999980815, 28.00000000000000000, 54.99999999999922551 ) ) ;
#10843=FACE_OUTER_BOUND ( 'NONE', #6371, .T. ) ;
#10846=CONICAL_SURFACE ( 'NONE', #5744, 57.00000000000002132, 0.7853981633974437271 ) ;
#10850=CARTESIAN_POINT ( 'NONE',  ( -11.68090480754633553, 3.765577839755389622, 57.90797000640144176 ) ) ;
#10852=CARTESIAN_POINT ( 'NONE',  ( -14.30947201679070346, 34.00909065834211731, -56.34794761833929044 ) ) ;
#10855=ORIENTED_EDGE ( 'NONE', *, *, #10401, .F. ) ;
#10856=CARTESIAN_POINT ( 'NONE',  ( -23.50000000000001066, 19.99999999999982947, 105.0000000000000142 ) ) ;
#10857=EDGE_CURVE ( 'NONE', #4421, #4117, #14367, .T. ) ;
#10858=CARTESIAN_POINT ( 'NONE',  ( -42.50000000000000711, -5.000000000000000000, -45.40000000000000568 ) ) ;
#10859=CARTESIAN_POINT ( 'NONE',  ( 14.94062893683334003, 18.45609313704557763, -45.79998742252195143 ) ) ;
#10869=ORIENTED_EDGE ( 'NONE', *, *, #10208, .T. ) ;
#10873=CARTESIAN_POINT ( 'NONE',  ( -9.857944917841395593, 0.2919354798322454925, 54.29891737064847490 ) ) ;
#10878=CARTESIAN_POINT ( 'NONE',  ( -5.863456460679469018, 40.00000000000000000, 52.03112161586459194 ) ) ;
#10883=EDGE_CURVE ( 'NONE', #17279, #4759, #22069, .T. ) ;
#10884=CARTESIAN_POINT ( 'NONE',  ( 6.696867368503558448E-15, 40.00000000000000000, 48.73397172404481381 ) ) ;
#10887=ORIENTED_EDGE ( 'NONE', *, *, #21284, .T. ) ;
#10890=CARTESIAN_POINT ( 'NONE',  ( -6.675595700168979185, 39.71118686595398373, -53.17234509353112770 ) ) ;
#10891=EDGE_LOOP ( 'NONE', ( #1831, #12485, #15068 ) ) ;
#10892=VECTOR ( 'NONE', #709, 1000.000000000000000 ) ;
#10897=B_SPLINE_CURVE_WITH_KNOTS ( 'NONE', 3,
 ( #19416, #42, #10234, #6932, #7138, #12298, #10453, #12186, #17452, #17569, #6813, #17341 ),
 .UNSPECIFIED., .F., .F.,
 ( 4, 2, 2, 2, 2, 4 ),
 ( 0.006347202264228479079, 0.007930096811551054850, 0.008721544085212341868, 0.009512991358873628886, 0.01109588590619620986, 0.01267878045351878910 ),
 .UNSPECIFIED. ) ;
#10899=VECTOR ( 'NONE', #22544, 1000.000000000000000 ) ;
#10900=VERTEX_POINT ( 'NONE', #19985 ) ;
#10903=EDGE_LOOP ( 'NONE', ( #19092, #22276, #20592 ) ) ;
#10906=CARTESIAN_POINT ( 'NONE',  ( 35.00000000000000000, 40.00000000000000000, 4.258610482196280173E-15 ) ) ;
#10920=CARTESIAN_POINT ( 'NONE',  ( 3.630528349514350772, 39.68566064946332972, -51.94954034995315340 ) ) ;
#10921=CARTESIAN_POINT ( 'NONE',  ( 42.50000000000000711, -5.000000000000000000, 47.50000000000000711 ) ) ;
#10922=CIRCLE ( 'NONE', #10176, 9.000000000000003553 ) ;
#10923=DIRECTION ( 'NONE',  ( 0.000000000000000000, 0.000000000000000000, -1.000000000000000000 ) ) ;
#10926=CARTESIAN_POINT ( 'NONE',  ( 17.83677152930479082, 10.91058841726731998, 60.06362461869429126 ) ) ;
#10928=CARTESIAN_POINT ( 'NONE',  ( 13.71171267332174715, 34.59605702017176299, -56.12298047978914894 ) ) ;
#10931=ADVANCED_FACE ( 'NONE', ( #16768 ), #3307, .F. ) ;
#10933=ORIENTED_EDGE ( 'NONE', *, *, #16176, .T. ) ;
#10934=ORIENTED_EDGE ( 'NONE', *, *, #903, .T. ) ;
#10936=ORIENTED_EDGE ( 'NONE', *, *, #11175, .T. ) ;
#10939=CARTESIAN_POINT ( 'NONE',  ( -10.44987231380843618, 39.22455541072930174, -54.81340832922769124 ) ) ;
#10948=FACE_OUTER_BOUND ( 'NONE', #6523, .T. ) ;
#10951=DIRECTION ( 'NONE',  ( 0.000000000000000000, 0.000000000000000000, 1.000000000000000000 ) ) ;
#10954=LINE ( 'NONE', #17831, #20492 ) ;
#10955=CARTESIAN_POINT ( 'NONE',  ( -5.133465198558034182, 39.34078186380426700, 53.02544092942117970 ) ) ;
#10957=EDGE_CURVE ( 'NONE', #16727, #9194, #170, .T. ) ;
#10960=VECTOR ( 'NONE', #15869, 1000.000000000000000 ) ;
#10963=DIRECTION ( 'NONE',  ( -0.000000000000000000, -1.000000000000000000, -0.000000000000000000 ) ) ;
#10964=CARTESIAN_POINT ( 'NONE',  ( 42.50000000000000711, -5.000000000000000000, -45.40000000000000568 ) ) ;
#10966=CIRCLE ( 'NONE', #11337, 9.000000000000003553 ) ;
#10970=CARTESIAN_POINT ( 'NONE',  ( -19.95262135541531379, 18.40707545474674589, 60.61067493606138612 ) ) ;
#10971=CARTESIAN_POINT ( 'NONE',  ( -18.05287651232776369, 33.35671069585768578, -57.55759232970981287 ) ) ;
#10973=CARTESIAN_POINT ( 'NONE',  ( 35.00000000000058265, 39.97500000000000142, -52.50000000000076739 ) ) ;
#10974=EDGE_CURVE ( 'NONE', #6468, #10753, #15478, .T. ) ;
#10978=DIRECTION ( 'NONE',  ( -0.000000000000000000, -1.000000000000000000, -0.000000000000000000 ) ) ;
#10981=DIRECTION ( 'NONE',  ( 0.000000000000000000, 1.000000000000000000, 0.000000000000000000 ) ) ;
#10986=DIRECTION ( 'NONE',  ( 1.000000000000000000, 0.000000000000000000, 0.000000000000000000 ) ) ;
#10987=EDGE_CURVE ( 'NONE', #6067, #11258, #1639, .T. ) ;
#10989=ORIENTED_EDGE ( 'NONE', *, *, #646, .F. ) ;
#10990=DIRECTION ( 'NONE',  ( 1.000000000000000000, 0.000000000000000000, 0.000000000000000000 ) ) ;
#10991=EDGE_CURVE ( 'NONE', #21584, #3760, #19167, .T. ) ;
#10995=DIRECTION ( 'NONE',  ( 0.000000000000000000, -1.000000000000000000, 0.000000000000000000 ) ) ;
#10996=VERTEX_POINT ( 'NONE', #14084 ) ;
#11003=B_SPLINE_CURVE_WITH_KNOTS ( 'NONE', 3,
 ( #16725, #15330, #18559, #22006, #20610, #2873, #6413, #4924, #10177, #8026, #14987, #13380, #20399, #4709, #18679, #2983, #91, #5484, #13840, #21184, #7084, #325 ),
 .UNSPECIFIED., .F., .F.,
 ( 4, 2, 2, 2, 2, 2, 2, 2, 2, 2, 4 ),
 ( 0.007712149587921354570, 0.01231940472852628525, 0.01347121851367751207, 0.01462303229882873888, 0.01692665986913119078, 0.01807847365428241759, 0.01923028743943364788, 0.02153391500973611539, 0.02268572879488734567, 0.02383754258003857943, 0.02614117015034102959 ),
 .UNSPECIFIED. ) ;
#11005=AXIS2_PLACEMENT_3D ( 'NONE', #4497, #9427, #1162 ) ;
#11006=CARTESIAN_POINT ( 'NONE',  ( -15.49999999999980282, -2.516660498395516310, 60.00099999999999767 ) ) ;
#11008=ORIENTED_EDGE ( 'NONE', *, *, #13168, .F. ) ;
#11010=CARTESIAN_POINT ( 'NONE',  ( -12.84005703541686749, 1.693876179762715983, 55.76322220626266812 ) ) ;
#11011=CARTESIAN_POINT ( 'NONE',  ( -3.944371625881058385, 39.90454848232354834, -51.54919429721285695 ) ) ;
#11012=ORIENTED_EDGE ( 'NONE', *, *, #14399, .F. ) ;
#11014=DIRECTION ( 'NONE',  ( 0.000000000000000000, 0.000000000000000000, 1.000000000000000000 ) ) ;
#11016=EDGE_CURVE ( 'NONE', #10179, #19351, #2662, .T. ) ;
#11020=DIRECTION ( 'NONE',  ( -0.000000000000000000, -0.000000000000000000, 1.000000000000000000 ) ) ;
#11022=CARTESIAN_POINT ( 'NONE',  ( 35.00000000000000000, -4.999999999999997335, 4.258610482196280173E-15 ) ) ;
#11025=CARTESIAN_POINT ( 'NONE',  ( -13.00000000000011546, 42.51666049839536043, 100.0000000000000000 ) ) ;
#11028=CARTESIAN_POINT ( 'NONE',  ( 17.00000000000000000, 20.00000000000000711, -102.0000000000000142 ) ) ;
#11030=AXIS2_PLACEMENT_3D ( 'NONE', #22399, #22294, #10448 ) ;
#11031=CARTESIAN_POINT ( 'NONE',  ( -42.50000000000000711, -5.000000000000000000, -49.60000000000000142 ) ) ;
#11034=ORIENTED_EDGE ( 'NONE', *, *, #10630, .T. ) ;
#11035=CARTESIAN_POINT ( 'NONE',  ( 3.244689583147291945, 39.74755540027157252, 52.34195286440930772 ) ) ;
#11036=CARTESIAN_POINT ( 'NONE',  ( 0.6211727382237610673, 4.802676810931882923E-16, 50.97074642427956093 ) ) ;
#11037=ORIENTED_EDGE ( 'NONE', *, *, #22659, .T. ) ;
#11039=CARTESIAN_POINT ( 'NONE',  ( 9.870870746772787641, 37.43479630315659534, 54.49920060628448937 ) ) ;
#11040=DIRECTION ( 'NONE',  ( 0.000000000000000000, 0.000000000000000000, 1.000000000000000000 ) ) ;
#11043=EDGE_CURVE ( 'NONE', #19599, #10325, #4542, .T. ) ;
#11047=ORIENTED_EDGE ( 'NONE', *, *, #504, .T. ) ;
#11052=ORIENTED_EDGE ( 'NONE', *, *, #9218, .F. ) ;
#11054=CARTESIAN_POINT ( 'NONE',  ( -4.084299015953898326, -4.682619376883251583, 48.27507093819014017 ) ) ;
#11063=DIRECTION ( 'NONE',  ( 0.000000000000000000, -1.000000000000000000, 0.000000000000000000 ) ) ;
#11065=CARTESIAN_POINT ( 'NONE',  ( -0.6290164960542528050, 40.00000000000000000, 49.48738346576863023 ) ) ;
#11069=ORIENTED_EDGE ( 'NONE', *, *, #14871, .T. ) ;
#11073=CARTESIAN_POINT ( 'NONE',  ( 6.002321937223278780, -0.8366808808176150469, -52.11647083208271169 ) ) ;
#11076=CARTESIAN_POINT ( 'NONE',  ( 5.233625953339160397E-15, -0.1272971988267498356, 49.60954963577236043 ) ) ;
#11077=LINE ( 'NONE', #19464, #18608 ) ;
#11078=CARTESIAN_POINT ( 'NONE',  ( -1.268121568161834523, 39.97056933375375110, -50.22305475357490678 ) ) ;
#11081=VERTEX_POINT ( 'NONE', #11462 ) ;
#11082=CARTESIAN_POINT ( 'NONE',  ( -42.50000000000000711, -5.000000000000000000, 47.50000000000000711 ) ) ;
#11083=DIRECTION ( 'NONE',  ( -0.000000000000000000, 1.000000000000000000, -0.000000000000000000 ) ) ;
#11084=DIRECTION ( 'NONE',  ( 0.000000000000000000, -1.000000000000000000, 0.000000000000000000 ) ) ;
#11085=FACE_OUTER_BOUND ( 'NONE', #19326, .T. ) ;
#11087=ADVANCED_FACE ( 'NONE', ( #18450 ), #13047, .F. ) ;
#11089=CIRCLE ( 'NONE', #4152, 6.499999999999999112 ) ;
#11090=VERTEX_POINT ( 'NONE', #18568 ) ;
#11093=CIRCLE ( 'NONE', #9638, 10.00000000000000178 ) ;
#11094=TOROIDAL_SURFACE ( 'NONE', #3058, 50.00000000000000000, 10.00000000000000000 ) ;
#11095=ORIENTED_EDGE ( 'NONE', *, *, #933, .T. ) ;
#11097=EDGE_CURVE ( 'NONE', #10123, #15736, #17690, .T. ) ;
#11098=TOROIDAL_SURFACE ( 'NONE', #9634, 22.00000000000000000, 2.000000000000000000 ) ;
#11099=CARTESIAN_POINT ( 'NONE',  ( 7.725164357189188813, 40.00000000000000000, -52.85294098179745248 ) ) ;
#11101=CARTESIAN_POINT ( 'NONE',  ( 4.586071060776173880, 39.86904401650008367, -51.95542086194134157 ) ) ;
#11102=CARTESIAN_POINT ( 'NONE',  ( 23.49999999999998579, 19.99999999999999645, -100.0000000000000000 ) ) ;
#11106=CARTESIAN_POINT ( 'NONE',  ( 35.00000000000058265, 28.00000000000000000, -57.50000000000076028 ) ) ;
#11107=AXIS2_PLACEMENT_3D ( 'NONE', #9862, #16851, #6083 ) ;
#11108=CARTESIAN_POINT ( 'NONE',  ( -9.750125222798885716, 39.99999999999999289, 53.58569999979536647 ) ) ;
#11110=ADVANCED_FACE ( 'NONE', ( #2652 ), #2709, .F. ) ;
#11112=EDGE_CURVE ( 'NONE', #21024, #5921, #18790, .T. ) ;
#11113=AXIS2_PLACEMENT_3D ( 'NONE', #560, #8926, #2399 ) ;
#11114=CARTESIAN_POINT ( 'NONE',  ( -7.549837901776227156, 39.99999999999999289, 52.78128042259339736 ) ) ;
#11119=CARTESIAN_POINT ( 'NONE',  ( -2.239819223192103692, 39.96978031709322465, -50.39586371513333063 ) ) ;
#11121=DIRECTION ( 'NONE',  ( -0.000000000000000000, 1.000000000000000000, -0.000000000000000000 ) ) ;
#11123=AXIS2_PLACEMENT_3D ( 'NONE', #7458, #2423, #16390 ) ;
#11126=EDGE_CURVE ( 'NONE', #19011, #18643, #4891, .T. ) ;
#11127=ORIENTED_EDGE ( 'NONE', *, *, #9996, .T. ) ;
#11130=CARTESIAN_POINT ( 'NONE',  ( 7.899727005596350438, 39.58366633022075121, -53.79762619906099275 ) ) ;
#11131=LINE ( 'NONE', #20084, #16006 ) ;
#11133=DIRECTION ( 'NONE',  ( -1.000000000000000000, 0.000000000000000000, 0.000000000000000000 ) ) ;
#11139=ADVANCED_FACE ( 'NONE', ( #22587 ), #7448, .F. ) ;
#11143=CYLINDRICAL_SURFACE ( 'NONE', #3875, 6.499999999999999112 ) ;
#11148=CARTESIAN_POINT ( 'NONE',  ( 4.278324951947499954, 39.54020021135884377, 53.33400390260334945 ) ) ;
#11151=DIRECTION ( 'NONE',  ( 0.000000000000000000, 0.000000000000000000, 1.000000000000000000 ) ) ;
#11152=FACE_OUTER_BOUND ( 'NONE', #2638, .T. ) ;
#11154=CARTESIAN_POINT ( 'NONE',  ( 35.00000000000058265, 40.00000000000000711, -55.00000000000076028 ) ) ;
#11156=AXIS2_PLACEMENT_3D ( 'NONE', #9841, #11768, #22102 ) ;
#11159=ORIENTED_EDGE ( 'NONE', *, *, #4435, .T. ) ;
#11161=DIRECTION ( 'NONE',  ( 0.000000000000000000, 0.000000000000000000, 1.000000000000000000 ) ) ;
#11166=CARTESIAN_POINT ( 'NONE',  ( -1.387778780781445676E-14, 20.00000000000000000, -98.00000000000000000 ) ) ;
#11168=VECTOR ( 'NONE', #6638, 1000.000000000000000 ) ;
#11173=ADVANCED_FACE ( 'NONE', ( #12031 ), #6718, .T. ) ;
#11175=EDGE_CURVE ( 'NONE', #19744, #22334, #500, .T. ) ;
#11177=CARTESIAN_POINT ( 'NONE',  ( 5.833333333333437842, 6.180730040185884455, -40.61164310337073857 ) ) ;
#11179=ADVANCED_FACE ( 'NONE', ( #20860 ), #18910, .F. ) ;
#11181=VECTOR ( 'NONE', #18688, 1000.000000000000000 ) ;
#11188=CARTESIAN_POINT ( 'NONE',  ( -0.6212853642548137323, -1.852178711329401354E-16, -50.97083105892616572 ) ) ;
#11190=CARTESIAN_POINT ( 'NONE',  ( 4.240553750831081103, 39.54840718952534218, 53.29860200223214406 ) ) ;
#11195=CYLINDRICAL_SURFACE ( 'NONE', #14944, 2.499999999999998668 ) ;
#11197=CIRCLE ( 'NONE', #20731, 15.00000000000000000 ) ;
#11198=EDGE_LOOP ( 'NONE', ( #14615, #18036, #6422, #11518 ) ) ;
#11199=DIRECTION ( 'NONE',  ( 0.000000000000000000, 0.000000000000000000, 1.000000000000000000 ) ) ;
#11200=DIRECTION ( 'NONE',  ( 0.000000000000000000, 0.000000000000000000, -1.000000000000000000 ) ) ;
#11203=CYLINDRICAL_SURFACE ( 'NONE', #14015, 2.099999999999997868 ) ;
#11210=CIRCLE ( 'NONE', #4661, 2.525000000000110489 ) ;
#11211=EDGE_CURVE ( 'NONE', #3042, #121, #15844, .T. ) ;
#11215=CARTESIAN_POINT ( 'NONE',  ( 0.4444706617113970970, 39.99884075969093544, -49.07683524994765634 ) ) ;
#11218=VERTEX_POINT ( 'NONE', #1600 ) ;
#11221=ORIENTED_EDGE ( 'NONE', *, *, #10691, .T. ) ;
#11222=CARTESIAN_POINT ( 'NONE',  ( -13.56354382738803466, 2.142135623730933247, -56.03997097393685323 ) ) ;
#11223=CARTESIAN_POINT ( 'NONE',  ( 13.31210290807009322, 38.06413856043591437, -55.94798518138998844 ) ) ;
#11227=AXIS2_PLACEMENT_3D ( 'NONE', #7942, #21930, #15017 ) ;
#11230=CIRCLE ( 'NONE', #19317, 2.524999999999999467 ) ;
#11236=ADVANCED_FACE ( 'NONE', ( #1078 ), #17178, .F. ) ;
#11239=ORIENTED_EDGE ( 'NONE', *, *, #15883, .T. ) ;
#11246=CARTESIAN_POINT ( 'NONE',  ( 19.71583072461104535, 23.39500837205462602, -60.55395521980172902 ) ) ;
#11247=CARTESIAN_POINT ( 'NONE',  ( 8.523345606421392162, -2.856915207551451452, 52.89411661606261106 ) ) ;
#11248=DIRECTION ( 'NONE',  ( 0.000000000000000000, -0.7071067811867928210, -0.7071067811863022134 ) ) ;
#11249=CARTESIAN_POINT ( 'NONE',  ( -17.00000000000000000, 20.00000000000000711, 102.0000000000000142 ) ) ;
#11256=CARTESIAN_POINT ( 'NONE',  ( -16.26546936781298314, 4.421830200407484313, -57.01255691153426852 ) ) ;
#11257=CARTESIAN_POINT ( 'NONE',  ( 19.52068517772377376, 15.62943592677015126, -60.50640500721814163 ) ) ;
#11258=VERTEX_POINT ( 'NONE', #1372 ) ;
#11260=FACE_OUTER_BOUND ( 'NONE', #16131, .T. ) ;
#11262=VERTEX_POINT ( 'NONE', #8586 ) ;
#11263=CARTESIAN_POINT ( 'NONE',  ( 6.433485051969655366, 38.94088993357593154, 55.16018527340020938 ) ) ;
#11264=CARTESIAN_POINT ( 'NONE',  ( -1.485717122675851432, -1.299971956346734459, 49.29290837556845872 ) ) ;
#11267=EDGE_CURVE ( 'NONE', #3791, #478, #8902, .T. ) ;
#11270=DIRECTION ( 'NONE',  ( -0.000000000000000000, -1.000000000000000000, -0.000000000000000000 ) ) ;
#11272=FACE_OUTER_BOUND ( 'NONE', #6159, .T. ) ;
#11277=CIRCLE ( 'NONE', #16024, 18.00000000000000355 ) ;
#11282=CARTESIAN_POINT ( 'NONE',  ( 35.00000000000000000, 40.00000000000000000, 4.258610482196280173E-15 ) ) ;
#11283=CONICAL_SURFACE ( 'NONE', #17495, 2.099999999999997868, 1.029744258676653867 ) ;
#11285=EDGE_CURVE ( 'NONE', #11348, #2120, #5164, .T. ) ;
#11288=CARTESIAN_POINT ( 'NONE',  ( 0.005803611680460589971, 39.99999985006627412, 48.73848948830625716 ) ) ;
#11289=ORIENTED_EDGE ( 'NONE', *, *, #3684, .F. ) ;
#11292=ADVANCED_FACE ( 'NONE', ( #2274 ), #18058, .F. ) ;
#11294=DIRECTION ( 'NONE',  ( -0.000000000000000000, -1.000000000000000000, -0.000000000000000000 ) ) ;
#11300=DIRECTION ( 'NONE',  ( -1.000000000000000000, 0.000000000000000000, 0.000000000000000000 ) ) ;
#11301=DIRECTION ( 'NONE',  ( 0.000000000000000000, 0.000000000000000000, -1.000000000000000000 ) ) ;
#11304=EDGE_CURVE ( 'NONE', #22506, #675, #11093, .T. ) ;
#11306=ADVANCED_FACE ( 'NONE', ( #9260 ), #14003, .F. ) ;
#11308=CARTESIAN_POINT ( 'NONE',  ( -18.99835506941826679, 13.52193747355387821, 57.87905887291319829 ) ) ;
#11311=AXIS2_PLACEMENT_3D ( 'NONE', #2486, #3862, #10828 ) ;
#11312=CIRCLE ( 'NONE', #17159, 2.499999999999995115 ) ;
#11314=CARTESIAN_POINT ( 'NONE',  ( -1.045703040280289819, 0.02735608008923263654, -49.70561346074465803 ) ) ;
#11315=ADVANCED_FACE ( 'NONE', ( #17741, #16243 ), #10519, .F. ) ;
#11316=CARTESIAN_POINT ( 'NONE',  ( 11.68090480754630178, 3.765577839755386069, 57.90797000640142045 ) ) ;
#11318=DIRECTION ( 'NONE',  ( -1.000000000000000000, 0.000000000000000000, 0.000000000000000000 ) ) ;
#11321=VERTEX_POINT ( 'NONE', #3560 ) ;
#11323=B_SPLINE_CURVE_WITH_KNOTS ( 'NONE', 3,
 ( #11591, #6435, #18586, #16518, #22024, #1055, #20082, #13277, #9759, #6316, #2775, #18244, #6212, #8047, #4732, #13398, #1159, #19962, #11246, #5981, #18125, #15006 ),
 .UNSPECIFIED., .F., .F.,
 ( 4, 2, 2, 2, 2, 2, 2, 2, 2, 2, 4 ),
 ( 0.000000000000000000, 0.005822207826702249442, 0.007277759783377814838, 0.008733311740053378500, 0.01164441565340452144, 0.01309996761008009811, 0.01455551956675567304, 0.01746662348010682639, 0.01892217543678240479, 0.02037772739345798320, 0.02328883130680912614 ),
 .UNSPECIFIED. ) ;
#11324=DIRECTION ( 'NONE',  ( 0.000000000000000000, 0.000000000000000000, -1.000000000000000000 ) ) ;
#11333=DIRECTION ( 'NONE',  ( 0.000000000000000000, 1.000000000000000000, 0.000000000000000000 ) ) ;
#11334=ORIENTED_EDGE ( 'NONE', *, *, #17148, .T. ) ;
#11336=DIRECTION ( 'NONE',  ( -0.000000000000000000, 1.000000000000000000, -0.000000000000000000 ) ) ;
#11337=AXIS2_PLACEMENT_3D ( 'NONE', #15458, #10082, #15696 ) ;
#11338=CARTESIAN_POINT ( 'NONE',  ( 6.176815998947249753, 40.00000000000000000, -52.17714723720779801 ) ) ;
#11340=CARTESIAN_POINT ( 'NONE',  ( 0.9695974223849092022, 39.99443194917778754, -49.47365400635877108 ) ) ;
#11343=CARTESIAN_POINT ( 'NONE',  ( 5.833333333333329485, 39.00000000000000711, -40.61164310337066041 ) ) ;
#11345=CARTESIAN_POINT ( 'NONE',  ( 23.49999999999998579, 19.99999999999999645, 60.00099999999999767 ) ) ;
#11346=CARTESIAN_POINT ( 'NONE',  ( -1.571417673354765121, 40.00000000000000711, 49.72695664780195557 ) ) ;
#11348=VERTEX_POINT ( 'NONE', #14174 ) ;
#11351=CARTESIAN_POINT ( 'NONE',  ( -0.03961255302991764649, 39.99999109211487536, -48.76478634770423071 ) ) ;
#11355=CARTESIAN_POINT ( 'NONE',  ( -13.25963002225074128, 27.02330685613479133, 45.02656532858658522 ) ) ;
#11357=EDGE_CURVE ( 'NONE', #19508, #17407, #20957, .T. ) ;
#11359=ORIENTED_EDGE ( 'NONE', *, *, #11690, .F. ) ;
#11361=CARTESIAN_POINT ( 'NONE',  ( 11.51554440985536054, 39.99999999999998579, 54.14601575511818510 ) ) ;
#11362=CARTESIAN_POINT ( 'NONE',  ( 7.682546357462705089, -2.941798577944364723, 52.37062424969784757 ) ) ;
#11364=DIRECTION ( 'NONE',  ( 0.000000000000000000, 0.000000000000000000, -1.000000000000000000 ) ) ;
#11365=CARTESIAN_POINT ( 'NONE',  ( -42.50000000000000711, -12.00000000000000000, -41.00000000000000000 ) ) ;
#11373=CARTESIAN_POINT ( 'NONE',  ( 3.179547380502777187, 39.99999999999999289, 50.65098720036137081 ) ) ;
#11374=ORIENTED_EDGE ( 'NONE', *, *, #18233, .F. ) ;
#11375=FACE_OUTER_BOUND ( 'NONE', #13366, .T. ) ;
#11376=CARTESIAN_POINT ( 'NONE',  ( -0.3446551741050853934, -0.009348518860262763908, 50.24945914274604064 ) ) ;
#11378=LINE ( 'NONE', #12971, #2057 ) ;
#11379=EDGE_CURVE ( 'NONE', #19741, #4643, #6362, .T. ) ;
#11381=CARTESIAN_POINT ( 'NONE',  ( 14.77818138858686048, 33.48299671874048045, 59.09975138256965010 ) ) ;
#11384=EDGE_CURVE ( 'NONE', #22334, #17065, #5269, .T. ) ;
#11386=CARTESIAN_POINT ( 'NONE',  ( 17.17026400045398304, 34.49621688465821023, -57.29349885535136622 ) ) ;
#11387=B_SPLINE_CURVE_WITH_KNOTS ( 'NONE', 3,
 ( #12469, #19482, #3786, #19380, #17755, #9052, #16031, #341, #6188, #16375, #2408, #4364, #14648, #11215, #2750, #21655, #11866, #7905, #911, #5845, #20281, #9731, #11340, #5952, #1454, #13152, #692, #12922, #18325, #19934, #18215, #16719, #4242, #10141, #14866, #17136, #8438, #4892, #7783, #1024, #2528, #9513, #21548, #20165, #13034, #12813, #11448, #11101, #6294, #19826, #13253, #16492, #18435, #800, #14757, #4127, #21772 ),
 .UNSPECIFIED., .F., .F.,
 ( 4, 2, 1, 1, 1, 2, 2, 2, 1, 1, 1, 2, 2, 2, 1, 1, 1, 2, 2, 2, 1, 1, 1, 1, 2, 2, 2, 1, 1, 1, 1, 1, 1, 2, 2, 2, 2, 4 ),
 ( 0.0001220703125000000000, 0.01574516296389847497, 0.02355670928959713653, 0.02746248245244646904, 0.02941536903387057672, 0.03039181232458206330, 0.03136825561529354989, 0.04699134826667931281, 0.05480289459237219080, 0.05870866775521863673, 0.06066155433664183888, 0.06163799762735343302, 0.06261444091806502021, 0.09386062622083597706, 0.1094837188722208726, 0.1172952651979133482, 0.1212010383607589475, 0.1231539249421811366, 0.1251068115236033118, 0.1875991821290926842, 0.2188453674318368292, 0.2344684600832089294, 0.2422800064088944383, 0.2461857795717378450, 0.2481386661531595761, 0.2500915527345812794, 0.3750762939455960510, 0.4375686645511029371, 0.4688148498538569631, 0.4844379425052339205, 0.4922494888309228989, 0.4961552619937668052, 0.4981081485751883142, 0.4990845918658983749, 0.5000610351566083800, 0.6250457763674563960, 0.7500305175783041900, 1.000000000000000000 ),
 .UNSPECIFIED. ) ;
#11392=CARTESIAN_POINT ( 'NONE',  ( 15.49999999999993960, 42.51666049839543149, -105.0000000000000142 ) ) ;
#11403=FACE_OUTER_BOUND ( 'NONE', #7607, .T. ) ;
#11404=EDGE_CURVE ( 'NONE', #16804, #5777, #8197, .T. ) ;
#11409=CARTESIAN_POINT ( 'NONE',  ( -1.575030625093513326, 39.98856684152734431, 49.93404140185739948 ) ) ;
#11413=ORIENTED_EDGE ( 'NONE', *, *, #6617, .T. ) ;
#11414=EDGE_CURVE ( 'NONE', #11797, #3437, #9601, .T. ) ;
#11416=CARTESIAN_POINT ( 'NONE',  ( -20.01613897799924047, 20.29830884309395600, 58.15166638929883192 ) ) ;
#11422=AXIS2_PLACEMENT_3D ( 'NONE', #13042, #2985, #21780 ) ;
#11423=DIRECTION ( 'NONE',  ( 0.000000000000000000, 1.000000000000000000, 0.000000000000000000 ) ) ;
#11426=DIRECTION ( 'NONE',  ( -0.000000000000000000, -1.000000000000000000, -0.000000000000000000 ) ) ;
#11427=CARTESIAN_POINT ( 'NONE',  ( -3.244689583143077094, 39.74755540027242517, -52.34195286441636341 ) ) ;
#11428=ADVANCED_FACE ( 'NONE', ( #8426 ), #11203, .F. ) ;
#11431=LINE ( 'NONE', #9497, #6359 ) ;
#11432=DIRECTION ( 'NONE',  ( 0.000000000000000000, 0.000000000000000000, 1.000000000000000000 ) ) ;
#11436=ORIENTED_EDGE ( 'NONE', *, *, #646, .T. ) ;
#11437=ORIENTED_EDGE ( 'NONE', *, *, #3180, .T. ) ;
#11439=CARTESIAN_POINT ( 'NONE',  ( 42.50000000000000711, -12.00000000000000000, -47.50000000000000000 ) ) ;
#11441=CIRCLE ( 'NONE', #14352, 2.000000000000000888 ) ;
#11444=AXIS2_PLACEMENT_3D ( 'NONE', #13305, #20329, #1294 ) ;
#11445=CARTESIAN_POINT ( 'NONE',  ( -42.50000000000000711, -9.600000000000001421, 50.00000000000000711 ) ) ;
#11448=CARTESIAN_POINT ( 'NONE',  ( 4.577493544539172454, 39.86955222714477998, -51.95007588729110637 ) ) ;
#11451=LINE ( 'NONE', #16610, #5413 ) ;
#11452=CARTESIAN_POINT ( 'NONE',  ( 9.689843208404422370, 39.33333333333334281, -54.54983754392748097 ) ) ;
#11453=CARTESIAN_POINT ( 'NONE',  ( -8.845639221078089420, 39.99999999999999289, 53.28397946285252829 ) ) ;
#11462=CARTESIAN_POINT ( 'NONE',  ( 29.99999999999998579, 20.00000000000000355, -100.0000000000000000 ) ) ;
#11463=VECTOR ( 'NONE', #6916, 1000.000000000000114 ) ;
#11465=EDGE_LOOP ( 'NONE', ( #16757, #17531, #15690, #1629, #6862, #4873 ) ) ;
#11467=CARTESIAN_POINT ( 'NONE',  ( -26.00000000000001421, 19.99999999999982947, -105.0000000000000142 ) ) ;
#11472=AXIS2_PLACEMENT_3D ( 'NONE', #8816, #5591, #2049 ) ;
#11476=CARTESIAN_POINT ( 'NONE',  ( 19.91015268464080279, 21.95549706463424400, 60.60051340835966016 ) ) ;
#11477=DIRECTION ( 'NONE',  ( -0.000000000000000000, -1.000000000000000000, -0.000000000000000000 ) ) ;
#11480=CARTESIAN_POINT ( 'NONE',  ( -4.108808078302945255, 5.537732191391603997, -39.55687577697710822 ) ) ;
#11485=CARTESIAN_POINT ( 'NONE',  ( -42.50000000000000711, -12.00000000000000000, 54.00000000000000711 ) ) ;
#11486=CARTESIAN_POINT ( 'NONE',  ( -22.16820537380702660, 16.50892643625844158, -58.61209530626887698 ) ) ;
#11488=CARTESIAN_POINT ( 'NONE',  ( 7.298342794717536198E-15, -4.765964690023824168, 45.28512947536575695 ) ) ;
#11489=VECTOR ( 'NONE', #4095, 1000.000000000000000 ) ;
#11490=CARTESIAN_POINT ( 'NONE',  ( 12.89955995983991421, 4.696256998628590473, -58.40693116658149364 ) ) ;
#11492=DIRECTION ( 'NONE',  ( -0.000000000000000000, 1.000000000000000000, -0.000000000000000000 ) ) ;
#11495=DIRECTION ( 'NONE',  ( 0.000000000000000000, 0.000000000000000000, 1.000000000000000000 ) ) ;
#11497=CARTESIAN_POINT ( 'NONE',  ( -3.095776913249378250E-14, -0.8525976281474469953, -48.47768327036356339 ) ) ;
#11499=UNCERTAINTY_MEASURE_WITH_UNIT (LENGTH_MEASURE( 1.000000000000000082E-05 ), #15604, 'distance_accuracy_value', 'NONE');
#11503=CONICAL_SURFACE ( 'NONE', #7836, 2.524999999999999467, 0.7853981633974482790 ) ;
#11504=CARTESIAN_POINT ( 'NONE',  ( 21.32594275109616433, 27.02633437841368291, -58.42208514511779072 ) ) ;
#11508=VECTOR ( 'NONE', #17992, 1000.000000000000000 ) ;
#11514=PRODUCT_DEFINITION_SHAPE ( 'NONE', 'NONE',  #17241 ) ;
#11518=ORIENTED_EDGE ( 'NONE', *, *, #18288, .F. ) ;
#11522=ORIENTED_EDGE ( 'NONE', *, *, #11211, .T. ) ;
#11527=CARTESIAN_POINT ( 'NONE',  ( -14.98515767422211198, 19.22844023086510745, 45.81928800960655934 ) ) ;
#11530=VERTEX_POINT ( 'NONE', #20267 ) ;
#11532=EDGE_CURVE ( 'NONE', #4643, #19741, #13664, .T. ) ;
#11534=CARTESIAN_POINT ( 'NONE',  ( -19.43475998741692834, 8.756352882855134467, 57.94642939675672721 ) ) ;
#11537=CARTESIAN_POINT ( 'NONE',  ( -11.19713514086471129, 39.99999999999999289, 54.03748032825711078 ) ) ;
#11538=CIRCLE ( 'NONE', #7522, 1.999999999999999778 ) ;
#11539=PLANE ( 'NONE',  #10455 ) ;
#11543=CARTESIAN_POINT ( 'NONE',  ( 3.235223465813951371, -4.647308930658565096, 47.76313845446021134 ) ) ;
#11547=CARTESIAN_POINT ( 'NONE',  ( 16.37028666999325210, 4.520534895872216907, 57.04777702420265939 ) ) ;
#11548=CIRCLE ( 'NONE', #6427, 30.00000000000000000 ) ;
#11549=DIRECTION ( 'NONE',  ( -0.000000000000000000, -0.000000000000000000, 1.000000000000000000 ) ) ;
#11552=CARTESIAN_POINT ( 'NONE',  ( -35.00000000000058265, 40.00000000000000000, -57.50000000000076028 ) ) ;
#11562=CARTESIAN_POINT ( 'NONE',  ( 0.7906703573358260240, 40.00000000000000000, -49.24721022140938231 ) ) ;
#11570=DIRECTION ( 'NONE',  ( 0.000000000000000000, 0.000000000000000000, 1.000000000000000000 ) ) ;
#11572=LINE ( 'NONE', #13258, #11168 ) ;
#11574=CARTESIAN_POINT ( 'NONE',  ( 42.50000000000000711, -9.600000000000001421, -45.40000000000000568 ) ) ;
#11578=CARTESIAN_POINT ( 'NONE',  ( 10.31465995609163322, 2.846668092512274484, -57.27881138850304410 ) ) ;
#11585=ORIENTED_EDGE ( 'NONE', *, *, #9396, .F. ) ;
#11587=ORIENTED_EDGE ( 'NONE', *, *, #9014, .F. ) ;
#11591=CARTESIAN_POINT ( 'NONE',  ( 8.331955809010596070, 38.18181818181818699, -56.36098470834070895 ) ) ;
#11594=ADVANCED_FACE ( 'NONE', ( #8651 ), #20807, .F. ) ;
#11595=CARTESIAN_POINT ( 'NONE',  ( 15.59166974688843688, 7.467814210042471146, 59.37578565761233307 ) ) ;
#11598=CARTESIAN_POINT ( 'NONE',  ( -35.00000000000000000, 2.142135623730931471, 1.387778780781445676E-14 ) ) ;
#11601=CARTESIAN_POINT ( 'NONE',  ( -6.696867368503558448E-15, 39.00000000000000711, -48.73397172404479960 ) ) ;
#11602=CARTESIAN_POINT ( 'NONE',  ( 6.447719747032748441E-15, -4.883049072963745019, 45.13706194851797449 ) ) ;
#11605=CARTESIAN_POINT ( 'NONE',  ( -5.249999999999978684, 40.00000000000000000, 41.42387596543811412 ) ) ;
#11610=CARTESIAN_POINT ( 'NONE',  ( -6.976621346229579856, 1.175841510106858667, -53.23008234738043853 ) ) ;
#11614=AXIS2_PLACEMENT_3D ( 'NONE', #8636, #10339, #15615 ) ;
#11615=CARTESIAN_POINT ( 'NONE',  ( 17.19628968518533085, 9.778502620742363760, -59.87797704339183724 ) ) ;
#11619=ORIENTED_EDGE ( 'NONE', *, *, #7958, .T. ) ;
#11622=ORIENTED_EDGE ( 'NONE', *, *, #5084, .F. ) ;
#11624=CARTESIAN_POINT ( 'NONE',  ( -8.460114887485421065, -4.900635314995738234, -50.56657553899492541 ) ) ;
#11625=ORIENTED_EDGE ( 'NONE', *, *, #19194, .T. ) ;
#11630=CARTESIAN_POINT ( 'NONE',  ( 5.340789179572837497, 39.27722415257166233, -54.28402915905239468 ) ) ;
#11631=DIRECTION ( 'NONE',  ( -0.000000000000000000, -1.000000000000000000, -0.000000000000000000 ) ) ;
#11632=CARTESIAN_POINT ( 'NONE',  ( -6.777919286276303216E-15, -4.184616259352855749, -46.01897913074525803 ) ) ;
#11635=EDGE_CURVE ( 'NONE', #20449, #4414, #19083, .T. ) ;
#11636=CARTESIAN_POINT ( 'NONE',  ( 10.99584631063768647, 3.272668205460784741, -57.61971594758620796 ) ) ;
#11638=ORIENTED_EDGE ( 'NONE', *, *, #3834, .F. ) ;
#11646=CARTESIAN_POINT ( 'NONE',  ( -14.30107462755440473, 5.991811841696772944, 58.93430465799253426 ) ) ;
#11665=EDGE_LOOP ( 'NONE', ( #3425, #17888, #18014, #8476, #18241, #3697, #7357 ) ) ;
#11666=FACE_OUTER_BOUND ( 'NONE', #15042, .T. ) ;
#11669=DIRECTION ( 'NONE',  ( -0.000000000000000000, 1.000000000000000000, -0.000000000000000000 ) ) ;
#11672=AXIS2_PLACEMENT_3D ( 'NONE', #15124, #16755, #13180 ) ;
#11674=FACE_OUTER_BOUND ( 'NONE', #17228, .T. ) ;
#11678=EDGE_CURVE ( 'NONE', #21198, #12113, #14002, .T. ) ;
#11680=CYLINDRICAL_SURFACE ( 'NONE', #21892, 2.500000000000002220 ) ;
#11682=DIRECTION ( 'NONE',  ( -1.000000000000000000, 0.000000000000000000, 0.000000000000000000 ) ) ;
#11685=ORIENTED_EDGE ( 'NONE', *, *, #9046, .F. ) ;
#11688=DIRECTION ( 'NONE',  ( 0.000000000000000000, -1.000000000000000000, 0.000000000000000000 ) ) ;
#11690=EDGE_CURVE ( 'NONE', #16507, #507, #5780, .T. ) ;
#11691=CARTESIAN_POINT ( 'NONE',  ( -0.06748528862095062864, 39.99997318105867805, -48.78643676837788945 ) ) ;
#11692=VERTEX_POINT ( 'NONE', #14350 ) ;
#11697=CIRCLE ( 'NONE', #9515, 2.099999999999997868 ) ;
#11700=ORIENTED_EDGE ( 'NONE', *, *, #469, .F. ) ;
#11701=DIRECTION ( 'NONE',  ( -0.000000000000000000, -1.000000000000000000, -0.000000000000000000 ) ) ;
#11704=CARTESIAN_POINT ( 'NONE',  ( -35.00000000000058265, 40.00000000000000000, -55.00000000000076028 ) ) ;
#11705=ADVANCED_FACE ( 'NONE', ( #3840 ), #19873, .F. ) ;
#11707=CARTESIAN_POINT ( 'NONE',  ( -12.99999999999980282, -2.516660498395516310, -105.0000000000000142 ) ) ;
#11710=LINE ( 'NONE', #2907, #1736 ) ;
#11712=DIRECTION ( 'NONE',  ( -0.000000000000000000, 1.000000000000000000, 0.000000000000000000 ) ) ;
#11714=CARTESIAN_POINT ( 'NONE',  ( 5.234365386614148186, 40.00000000000000711, 51.72901478475910153 ) ) ;
#11716=CARTESIAN_POINT ( 'NONE',  ( -8.413264671629002933, 39.99999999999999289, -53.12447868246846383 ) ) ;
#11718=CYLINDRICAL_SURFACE ( 'NONE', #9379, 10.00000000000000178 ) ;
#11719=CARTESIAN_POINT ( 'NONE',  ( -5.863435294608654486E-12, 3.518151346420735669E-15, -50.27768525408826150 ) ) ;
#11720=VERTEX_POINT ( 'NONE', #2115 ) ;
#11721=CARTESIAN_POINT ( 'NONE',  ( -35.00000000000058265, 26.00000000000000355, -52.90000000000076597 ) ) ;
#11724=LINE ( 'NONE', #18370, #19159 ) ;
#11726=CARTESIAN_POINT ( 'NONE',  ( 20.65262896361246803, 28.82759387226735370, -58.26038807538034803 ) ) ;
#11727=VERTEX_POINT ( 'NONE', #4179 ) ;
#11729=VERTEX_POINT ( 'NONE', #620 ) ;
#11730=ORIENTED_EDGE ( 'NONE', *, *, #8336, .F. ) ;
#11731=ORIENTED_EDGE ( 'NONE', *, *, #14414, .F. ) ;
#11740=EDGE_LOOP ( 'NONE', ( #593, #976, #19303, #19809 ) ) ;
#11741=CARTESIAN_POINT ( 'NONE',  ( 6.869660410832048036, 39.72568940399584392, -53.24677441048955728 ) ) ;
#11743=CARTESIAN_POINT ( 'NONE',  ( 35.00000000000000000, 40.00000000000000000, 4.258610482196280173E-15 ) ) ;
#11745=CARTESIAN_POINT ( 'NONE',  ( -19.91015268464082411, 21.95549706463424755, -60.60051340835962463 ) ) ;
#11750=CIRCLE ( 'NONE', #4810, 49.99999999999998579 ) ;
#11751=ORIENTED_EDGE ( 'NONE', *, *, #13130, .F. ) ;
#11752=ADVANCED_FACE ( 'NONE', ( #6005 ), #6328, .F. ) ;
#11753=ORIENTED_EDGE ( 'NONE', *, *, #1305, .T. ) ;
#11754=CARTESIAN_POINT ( 'NONE',  ( -20.01704759191785499, 20.30656121192005870, 60.62580324355963057 ) ) ;
#11757=CARTESIAN_POINT ( 'NONE',  ( -12.15643230334918279, 39.99999999999999289, 54.39836425128645914 ) ) ;
#11758=EDGE_CURVE ( 'NONE', #5648, #3905, #9244, .T. ) ;
#11761=CARTESIAN_POINT ( 'NONE',  ( -6.043799261040989634, 39.99999999999999289, -52.11526435034569715 ) ) ;
#11763=CARTESIAN_POINT ( 'NONE',  ( 11.87329829276352200, 39.99999999999998579, -54.28004929203127205 ) ) ;
#11765=VERTEX_POINT ( 'NONE', #18150 ) ;
#11768=DIRECTION ( 'NONE',  ( -0.000000000000000000, 1.000000000000000000, -0.000000000000000000 ) ) ;
#11769=CARTESIAN_POINT ( 'NONE',  ( -8.479740367039939386, -4.901256658985757575, -50.57596245086818243 ) ) ;
#11771=VERTEX_POINT ( 'NONE', #499 ) ;
#11773=CARTESIAN_POINT ( 'NONE',  ( -9.327259741686505734, -2.742977062671840827, 53.40697683846378396 ) ) ;
#11777=EDGE_CURVE ( 'NONE', #2375, #1150, #2577, .T. ) ;
#11779=CARTESIAN_POINT ( 'NONE',  ( 1.079570778443343260, 34.99943186904513936, -38.73482392062543767 ) ) ;
#11781=CARTESIAN_POINT ( 'NONE',  ( -18.56336306567920502, 12.50537704746205847, -60.26262883998990816 ) ) ;
#11786=CARTESIAN_POINT ( 'NONE',  ( 13.75658951623322679, 25.99185038947792847, 45.26303799332217181 ) ) ;
#11788=CARTESIAN_POINT ( 'NONE',  ( 10.62139969368193881, 0.6004703193305798159, -54.70636795414631592 ) ) ;
#11792=AXIS2_PLACEMENT_3D ( 'NONE', #19661, #12424, #3740 ) ;
#11797=VERTEX_POINT ( 'NONE', #21706 ) ;
#11800=EDGE_CURVE ( 'NONE', #18495, #3688, #16083, .T. ) ;
#11805=DIRECTION ( 'NONE',  ( -0.000000000000000000, 1.000000000000000000, -0.000000000000000000 ) ) ;
#11806=AXIS2_PLACEMENT_3D ( 'NONE', #15406, #4784, #1113 ) ;
#11808=CYLINDRICAL_SURFACE ( 'NONE', #22303, 2.500000000000002220 ) ;
#11814=AXIS2_PLACEMENT_3D ( 'NONE', #16279, #5868, #4149 ) ;
#11819=DIRECTION ( 'NONE',  ( -0.000000000000000000, 1.000000000000000000, -0.000000000000000000 ) ) ;
#11821=DIRECTION ( 'NONE',  ( 0.000000000000000000, 0.000000000000000000, 1.000000000000000000 ) ) ;
#11822=CARTESIAN_POINT ( 'NONE',  ( -13.31210290807011276, 38.06413856043590727, 55.94798518139002397 ) ) ;
#11827=B_SPLINE_SURFACE_WITH_KNOTS ( 'NONE', 1, 3, ( 
 ( #15520, #13914, #6719, #15640, #20931, #19666 ),
 ( #7628, #14485, #4195, #7396, #14604, #18042 ) ),
 .UNSPECIFIED., .F., .F., .F.,
 ( 2, 2 ),
 ( 4, 2, 4 ),
 ( 0.000000000000000000, 1.000000000000000000 ),
 ( 0.000000000000000000, 0.001214050925800259527, 0.002428101851600519053 ),
 .UNSPECIFIED. ) ;
#11828=CARTESIAN_POINT ( 'NONE',  ( 21.60519577075306685, 26.10363331747821647, -58.48615516158968575 ) ) ;
#11829=EDGE_CURVE ( 'NONE', #11530, #14814, #6691, .T. ) ;
#11840=CARTESIAN_POINT ( 'NONE',  ( -42.50000000000000711, -12.00000000000000000, 47.50000000000000711 ) ) ;
#11843=CARTESIAN_POINT ( 'NONE',  ( 15.99999999999997335, 20.00000000000000355, -102.0000000000000142 ) ) ;
#11844=CARTESIAN_POINT ( 'NONE',  ( -5.961618526223441350, -3.061744126952760325, -51.29856354178470212 ) ) ;
#11845=ORIENTED_EDGE ( 'NONE', *, *, #10811, .F. ) ;
#11847=DIRECTION ( 'NONE',  ( 0.000000000000000000, 1.000000000000000000, 0.000000000000000000 ) ) ;
#11850=CARTESIAN_POINT ( 'NONE',  ( -1.387778780781445518E-14, 20.00000000000000355, 102.0000000000000142 ) ) ;
#11851=ADVANCED_FACE ( 'NONE', ( #8072 ), #20972, .F. ) ;
#11857=CARTESIAN_POINT ( 'NONE',  ( 11.68090480754629112, 3.765577839755377187, -57.90797000640139913 ) ) ;
#11858=CONICAL_SURFACE ( 'NONE', #4203, 18.00000000000000000, 0.7853981633974466137 ) ;
#11864=DIRECTION ( 'NONE',  ( 0.000000000000000000, 0.000000000000000000, 1.000000000000000000 ) ) ;
#11866=CARTESIAN_POINT ( 'NONE',  ( 0.5386985600499774041, 39.99828252980264409, -49.14867219490655259 ) ) ;
#11867=CARTESIAN_POINT ( 'NONE',  ( -16.07406985629802421, 8.092854060485290546, -59.53272467997609141 ) ) ;
#11868=CARTESIAN_POINT ( 'NONE',  ( -11.13570271988771232, 40.00000000000000000, 54.01634158485468618 ) ) ;
#11871=EDGE_LOOP ( 'NONE', ( #13585, #18156, #15200, #340 ) ) ;
#11874=CARTESIAN_POINT ( 'NONE',  ( -8.448970479837855763, 40.00000000000000000, -53.13698760634334661 ) ) ;
#11875=LINE ( 'NONE', #20485, #14540 ) ;
#11876=FACE_OUTER_BOUND ( 'NONE', #2122, .T. ) ;
#11878=ADVANCED_FACE ( 'NONE', ( #18830 ), #20105, .F. ) ;
#11880=EDGE_LOOP ( 'NONE', ( #8293, #21204 ) ) ;
#11882=CARTESIAN_POINT ( 'NONE',  ( -12.99999999999980282, -2.516660498395516310, 100.0000000000000000 ) ) ;
#11885=ORIENTED_EDGE ( 'NONE', *, *, #9046, .T. ) ;
#11889=CARTESIAN_POINT ( 'NONE',  ( -5.786532357731522858, -4.768624102719487112, 49.22393831245486950 ) ) ;
#11893=CARTESIAN_POINT ( 'NONE',  ( 14.99999999999998579, 20.00000000000000000, 45.82575694955838230 ) ) ;
#11895=DIRECTION ( 'NONE',  ( 0.000000000000000000, 0.000000000000000000, 1.000000000000000000 ) ) ;
#11897=CARTESIAN_POINT ( 'NONE',  ( -19.67606655124792780, 9.154757266468241284, -58.01240525280853433 ) ) ;
#11898=CARTESIAN_POINT ( 'NONE',  ( -7.471700997414055578, 39.63178059879609805, 53.58785626114602252 ) ) ;
#11903=DIRECTION ( 'NONE',  ( -0.000000000000000000, -0.000000000000000000, -1.000000000000000000 ) ) ;
#11905=DIRECTION ( 'NONE',  ( 0.000000000000000000, 0.000000000000000000, 1.000000000000000000 ) ) ;
#11907=ORIENTED_EDGE ( 'NONE', *, *, #431, .T. ) ;
#11910=CARTESIAN_POINT ( 'NONE',  ( 2.109039589833486161, 5.113963322222096153, 38.90259428073981240 ) ) ;
#11912=AXIS2_PLACEMENT_3D ( 'NONE', #15066, #11423, #999 ) ;
#11915=ADVANCED_FACE ( 'NONE', ( #18611 ), #18486, .F. ) ;
#11916=AXIS2_PLACEMENT_3D ( 'NONE', #5218, #8766, #2107 ) ;
#11919=EDGE_LOOP ( 'NONE', ( #20091, #15086, #17160, #12729 ) ) ;
#11925=DIRECTION ( 'NONE',  ( -0.000000000000000000, -0.000000000000000000, -1.000000000000000000 ) ) ;
#11928=CARTESIAN_POINT ( 'NONE',  ( -11.15511648636534048, 39.11609166919075875, 55.07420106209026756 ) ) ;
#11929=ORIENTED_EDGE ( 'NONE', *, *, #789, .T. ) ;
#11931=CARTESIAN_POINT ( 'NONE',  ( -42.50000000000000711, -9.600000000000001421, -45.40000000000000568 ) ) ;
#11935=CARTESIAN_POINT ( 'NONE',  ( 14.69988787053502222, 23.08500126984897349, -45.69379240540676079 ) ) ;
#11936=EDGE_CURVE ( 'NONE', #19954, #9032, #11724, .T. ) ;
#11938=CARTESIAN_POINT ( 'NONE',  ( 5.004946378181853284, 0.5943096879531043486, -54.03132084814315306 ) ) ;
#11940=VECTOR ( 'NONE', #10599, 1000.000000000000000 ) ;
#11941=CARTESIAN_POINT ( 'NONE',  ( -22.32664865868314763, 17.89874346835047092, 58.64628984943162493 ) ) ;
#11944=ORIENTED_EDGE ( 'NONE', *, *, #14871, .F. ) ;
#11946=DIRECTION ( 'NONE',  ( -0.000000000000000000, 1.000000000000000000, -0.000000000000000000 ) ) ;
#11950=CARTESIAN_POINT ( 'NONE',  ( 15.00671337312779663, 3.288799316213545154, -56.57538198732802215 ) ) ;
#11957=CARTESIAN_POINT ( 'NONE',  ( 21.80163436544120970, 14.71892543950345100, 58.53048140122282916 ) ) ;
#11959=ORIENTED_EDGE ( 'NONE', *, *, #7534, .T. ) ;
#11960=FACE_BOUND ( 'NONE', #19168, .T. ) ;
#11962=ORIENTED_EDGE ( 'NONE', *, *, #5855, .T. ) ;
#11963=CARTESIAN_POINT ( 'NONE',  ( 6.696867368503558448E-15, 40.00000000000000000, 48.73397172404481381 ) ) ;
#11965=CARTESIAN_POINT ( 'NONE',  ( 35.00000000000000000, 39.00000000000000711, 4.258610482196280173E-15 ) ) ;
#11968=VERTEX_POINT ( 'NONE', #13194 ) ;
#11969=DIRECTION ( 'NONE',  ( 0.000000000000000000, 0.000000000000000000, 1.000000000000000000 ) ) ;
#11970=CARTESIAN_POINT ( 'NONE',  ( -15.99999999999994493, 20.00000000000000355, 102.0000000000000142 ) ) ;
#11972=CARTESIAN_POINT ( 'NONE',  ( -3.658199643160841230, 39.91812894417287083, 51.36232514819826633 ) ) ;
#11973=AXIS2_PLACEMENT_3D ( 'NONE', #5399, #7109, #578 ) ;
#11975=ADVANCED_FACE ( 'NONE', ( #20216 ), #4520, .F. ) ;
#11976=CIRCLE ( 'NONE', #22224, 6.499999999999999112 ) ;
#11978=VERTEX_POINT ( 'NONE', #1083 ) ;
#11979=EDGE_LOOP ( 'NONE', ( #10810, #5762, #16428, #11069, #11625, #17874, #2456, #4712, #1117, #13702, #19540, #7793, #11127, #11983 ) ) ;
#11981=VECTOR ( 'NONE', #19555, 1000.000000000000000 ) ;
#11983=ORIENTED_EDGE ( 'NONE', *, *, #4663, .T. ) ;
#11985=CARTESIAN_POINT ( 'NONE',  ( -35.00000000000000000, 25.00000000000000000, 1.387778780781445676E-14 ) ) ;
#11987=AXIS2_PLACEMENT_3D ( 'NONE', #605, #16412, #21583 ) ;
#11991=CARTESIAN_POINT ( 'NONE',  ( -10.75185716664304358, 40.00000000000000000, 53.88525272612042727 ) ) ;
#11994=CARTESIAN_POINT ( 'NONE',  ( -34.99999999999999289, 2.142135623730931471, 60.00000000000001421 ) ) ;
#11995=CARTESIAN_POINT ( 'NONE',  ( -5.890136611214193074, 40.00000000000000711, -52.04311946512136444 ) ) ;
#11997=B_SPLINE_CURVE_WITH_KNOTS ( 'NONE', 3,
 ( #8003, #6387, #19805, #663, #13012, #4566, #11543, #18533, #2504, #21748 ),
 .UNSPECIFIED., .F., .F.,
 ( 4, 2, 2, 2, 4 ),
 ( 0.000000000000000000, 0.002975785561746833834, 0.005951571123493670269, 0.008927356685240507572, 0.01190314224698734054 ),
 .UNSPECIFIED. ) ;
#11998=CYLINDRICAL_SURFACE ( 'NONE', #14079, 6.499999999999999112 ) ;
#12000=CARTESIAN_POINT ( 'NONE',  ( 8.657955327455969297, 40.00000000000002132, -53.21471618982314311 ) ) ;
#12003=EDGE_LOOP ( 'NONE', ( #18763, #9635, #18045, #17071 ) ) ;
#12008=AXIS2_PLACEMENT_3D ( 'NONE', #16211, #10826, #15865 ) ;
#12009=CARTESIAN_POINT ( 'NONE',  ( 0.000000000000000000, 40.00000000000000000, 9.068199145005368464E-15 ) ) ;
#12011=EDGE_CURVE ( 'NONE', #15997, #13383, #19892, .T. ) ;
#12013=EDGE_CURVE ( 'NONE', #18007, #21600, #10220, .T. ) ;
#12015=CARTESIAN_POINT ( 'NONE',  ( 1.040180180071618610, -3.147605209281759464, 46.52651510289677361 ) ) ;
#12018=CARTESIAN_POINT ( 'NONE',  ( -34.99999999999999289, 2.142135623730931471, 50.00000000000001421 ) ) ;
#12019=EDGE_LOOP ( 'NONE', ( #10989, #21452 ) ) ;
#12021=CARTESIAN_POINT ( 'NONE',  ( 12.48541242016034403, 11.67824612544539420, 44.64471390988170896 ) ) ;
#12024=CARTESIAN_POINT ( 'NONE',  ( -19.88513910325156431, 17.69449494136243572, -58.11726460477454737 ) ) ;
#12028=DIRECTION ( 'NONE',  ( -0.000000000000000000, -1.000000000000000000, -0.000000000000000000 ) ) ;
#12030=FACE_BOUND ( 'NONE', #3589, .T. ) ;
#12031=FACE_OUTER_BOUND ( 'NONE', #22474, .T. ) ;
#12032=ORIENTED_EDGE ( 'NONE', *, *, #4252, .T. ) ;
#12038=CARTESIAN_POINT ( 'NONE',  ( -22.05221796475962392, 24.18157222985895061, -58.58672997744003652 ) ) ;
#12040=EDGE_CURVE ( 'NONE', #21119, #8612, #6345, .T. ) ;
#12043=DIRECTION ( 'NONE',  ( -1.000000000000000000, 0.000000000000000000, 0.000000000000000000 ) ) ;
#12044=DIRECTION ( 'NONE',  ( -0.000000000000000000, -1.000000000000000000, -0.000000000000000000 ) ) ;
#12046=FACE_OUTER_BOUND ( 'NONE', #15531, .T. ) ;
#12048=CARTESIAN_POINT ( 'NONE',  ( -1.387778780781445518E-14, 20.00000000000000355, -102.9999999999999716 ) ) ;
#12049=CARTESIAN_POINT ( 'NONE',  ( -12.24744603030440970, 40.00000000000000000, 54.43639671998951002 ) ) ;
#12050=ORIENTED_EDGE ( 'NONE', *, *, #19732, .T. ) ;
#12051=LINE ( 'NONE', #8606, #8313 ) ;
#12052=ADVANCED_FACE ( 'NONE', ( #14087 ), #3595, .F. ) ;
#12053=FACE_OUTER_BOUND ( 'NONE', #16571, .T. ) ;
#12055=CARTESIAN_POINT ( 'NONE',  ( 5.400043148885023570, 39.81718169346567748, 52.45350586640867618 ) ) ;
#12056=CARTESIAN_POINT ( 'NONE',  ( -2.633052209763709239, 39.95897179397861265, -50.67294425775457967 ) ) ;
#12057=ORIENTED_EDGE ( 'NONE', *, *, #7731, .T. ) ;
#12059=CARTESIAN_POINT ( 'NONE',  ( -11.86180952234344588, 38.99999999999292299, 55.35904751185378103 ) ) ;
#12060=ORIENTED_EDGE ( 'NONE', *, *, #20881, .T. ) ;
#12063=( BOUNDED_SURFACE ( )  B_SPLINE_SURFACE ( 3, 2, ( 
 ( #13551, #4870, #6472 ),
 ( #20229, #18501, #20344 ),
 ( #17000, #4651, #11624 ),
 ( #18628, #11844, #1308 ),
 ( #1195, #13437, #2933 ),
 ( #10120, #16896, #18846 ),
 ( #3150, #12080, #10667 ),
 ( #13778, #17674, #1774 ),
 ( #21018, #1984, #1877 ),
 ( #17227, #8758, #3495 ) ),
 .UNSPECIFIED., .F., .F., .F. ) 
 B_SPLINE_SURFACE_WITH_KNOTS ( ( 4, 2, 2, 2, 4 ),
 ( 3, 3 ),
 ( 0.02809317535148383310, 0.03071213539476958312, 0.03333109543805533315, 0.03595005548134108664, 0.03856901552462683319 ),
 ( 0.2389732943673004428, 1.000000000000000000 ),
 .UNSPECIFIED. ) 
 GEOMETRIC_REPRESENTATION_ITEM ( )  RATIONAL_B_SPLINE_SURFACE ( (
 ( 0.9723126933862541454, 0.9420702913958439728, 1.000000000000000000),
 ( 0.9749922925143332808, 0.9476767737753362120, 1.000000000000000000),
 ( 0.9774153414778116167, 0.9527464803504863688, 1.000000000000000000),
 ( 0.9815341666524188824, 0.9613642323581159665, 1.000000000000000000),
 ( 0.9832251939807838959, 0.9649023417791752211, 1.000000000000000000),
 ( 0.9856873122312947988, 0.9700537923984370314, 1.000000000000000000),
 ( 0.9864553338148032147, 0.9716607116685207490, 1.000000000000000000),
 ( 0.9870557760262982372, 0.9729170072999733243, 1.000000000000000000),
 ( 0.9868934176577572881, 0.9725773074833666820, 1.000000000000000000),
 ( 0.9863383242652690175, 0.9714158944602964141, 1.000000000000000000) ) ) 
 REPRESENTATION_ITEM ( '' )  SURFACE ( )  );
#12070=VERTEX_POINT ( 'NONE', #15597 ) ;
#12071=ORIENTED_EDGE ( 'NONE', *, *, #13589, .F. ) ;
#12072=CARTESIAN_POINT ( 'NONE',  ( 42.50000000000000711, -12.00000000000000000, 47.50000000000000711 ) ) ;
#12077=CARTESIAN_POINT ( 'NONE',  ( 8.410512267088693150, 40.00000000000000711, -53.12343718209208987 ) ) ;
#12079=DIRECTION ( 'NONE',  ( -0.000000000000000000, 1.000000000000000000, -0.000000000000000000 ) ) ;
#12080=CARTESIAN_POINT ( 'NONE',  ( -2.419767991116313688, -3.149022461034792109, -49.02154318834896429 ) ) ;
#12082=EDGE_CURVE ( 'NONE', #20866, #7020, #7124, .T. ) ;
#12083=CARTESIAN_POINT ( 'NONE',  ( -12.99999999999980282, -2.516660498395516310, 100.0000000000000000 ) ) ;
#12086=CARTESIAN_POINT ( 'NONE',  ( 4.078319513017754971, 34.44279552714540671, 39.58919430873140755 ) ) ;
#12090=ADVANCED_FACE ( 'NONE', ( #5306 ), #11094, .T. ) ;
#12098=ORIENTED_EDGE ( 'NONE', *, *, #14031, .T. ) ;
#12099=CARTESIAN_POINT ( 'NONE',  ( 35.00000000000000000, -9.000000000000001776, -18.00000000000000000 ) ) ;
#12102=CARTESIAN_POINT ( 'NONE',  ( 3.655628638892812088, 39.91824801334192330, 51.36063814675617323 ) ) ;
#12103=EDGE_CURVE ( 'NONE', #12952, #15024, #17436, .T. ) ;
#12109=CARTESIAN_POINT ( 'NONE',  ( 9.689843208404399277, 39.33333333333334281, -54.54983754392740281 ) ) ;
#12113=VERTEX_POINT ( 'NONE', #8742 ) ;
#12114=CARTESIAN_POINT ( 'NONE',  ( -8.620004424458363346, 38.06588350694461553, 54.65497187427080661 ) ) ;
#12117=EDGE_CURVE ( 'NONE', #7482, #21816, #477, .T. ) ;
#12120=EDGE_CURVE ( 'NONE', #17695, #6172, #21110, .T. ) ;
#12123=DIRECTION ( 'NONE',  ( -0.000000000000000000, -0.000000000000000000, -1.000000000000000000 ) ) ;
#12125=ADVANCED_FACE ( 'NONE', ( #1969 ), #18407, .T. ) ;
#12126=ORIENTED_EDGE ( 'NONE', *, *, #14203, .T. ) ;
#12129=LINE ( 'NONE', #6635, #9960 ) ;
#12131=CARTESIAN_POINT ( 'NONE',  ( -21.16618710811416904, 27.45243199383212485, -58.38369730662816437 ) ) ;
#12132=EDGE_CURVE ( 'NONE', #478, #2004, #14061, .T. ) ;
#12134=ORIENTED_EDGE ( 'NONE', *, *, #1184, .F. ) ;
#12136=B_SPLINE_CURVE_WITH_KNOTS ( 'NONE', 3,
 ( #16389, #15099, #20739, #17174, #2987, #20403, #2876, #16947, #1037, #11786, #22238, #3093, #9956, #6758, #17061, #8472, #1253, #15440, #15218, #10063, #13720, #20615, #4927, #22462 ),
 .UNSPECIFIED., .F., .F.,
 ( 4, 2, 2, 2, 2, 2, 2, 2, 2, 2, 2, 4 ),
 ( 0.02614117015034102265, 0.02729036340605313360, 0.02843955666176524455, 0.03073794317318946645, 0.03188713642890157740, 0.03303632968461368141, 0.03533471619603791025, 0.03648390945175002120, 0.03763310270746213215, 0.03993148921888635405, 0.04222987573031057595, 0.04452826224173479785 ),
 .UNSPECIFIED. ) ;
#12138=FACE_OUTER_BOUND ( 'NONE', #14781, .T. ) ;
#12139=DIRECTION ( 'NONE',  ( 0.000000000000000000, 0.000000000000000000, 1.000000000000000000 ) ) ;
#12141=ORIENTED_EDGE ( 'NONE', *, *, #1295, .F. ) ;
#12144=CONICAL_SURFACE ( 'NONE', #15055, 2.099999999999997868, 1.029744258676652091 ) ;
#12148=CARTESIAN_POINT ( 'NONE',  ( -35.00000000000058265, 40.00000000000000711, -57.52500000000076597 ) ) ;
#12153=VERTEX_POINT ( 'NONE', #3704 ) ;
#12154=CARTESIAN_POINT ( 'NONE',  ( -42.50000000000000711, -12.00000000000012434, -47.50000000000000000 ) ) ;
#12159=CARTESIAN_POINT ( 'NONE',  ( 14.27302218980889315, 2.669631712211250285, -56.31136122552219803 ) ) ;
#12167=DIRECTION ( 'NONE',  ( 0.000000000000000000, 0.000000000000000000, 1.000000000000000000 ) ) ;
#12168=ORIENTED_EDGE ( 'NONE', *, *, #9555, .T. ) ;
#12170=EDGE_CURVE ( 'NONE', #15875, #6249, #5599, .T. ) ;
#12180=CARTESIAN_POINT ( 'NONE',  ( 16.26546936781294050, 4.421830200407478983, 57.01255691153428984 ) ) ;
#12181=EDGE_CURVE ( 'NONE', #11321, #5360, #14208, .T. ) ;
#12182=DIRECTION ( 'NONE',  ( 0.000000000000000000, 0.000000000000000000, 1.000000000000000000 ) ) ;
#12183=CARTESIAN_POINT ( 'NONE',  ( 8.540030399951877627, 39.99999999999999289, 53.17106804086055405 ) ) ;
#12186=CARTESIAN_POINT ( 'NONE',  ( -3.604218085003659588, 5.430620144867039478, 39.39148225573723749 ) ) ;
#12189=CARTESIAN_POINT ( 'NONE',  ( 5.422702462874749330, 33.99260377204210926, 40.31673423471877271 ) ) ;
#12191=CARTESIAN_POINT ( 'NONE',  ( 2.576224933359552605, 39.84426458497861034, -51.65025110506227435 ) ) ;
#12192=CARTESIAN_POINT ( 'NONE',  ( -0.7806882667109514840, 39.98538465716378454, 49.65403242876611500 ) ) ;
#12194=AXIS2_PLACEMENT_3D ( 'NONE', #21716, #5554, #19546 ) ;
#12206=EDGE_CURVE ( 'NONE', #6302, #13976, #8180, .T. ) ;
#12207=CARTESIAN_POINT ( 'NONE',  ( 42.50000000000000711, -5.000000000000000000, 49.60000000000000853 ) ) ;
#12208=B_SPLINE_SURFACE_WITH_KNOTS ( 'NONE', 1, 3, ( 
 ( #21813, #20093, #4398, #2910, #11373, #2789, #20321, #11714, #20886, #9983, #15248, #21, #20646, #13968, #7011, #1285, #20766, #17202, #4745, #3015 ),
 ( #22268, #10315, #15705, #8277, #17311, #5078, #17089, #1515, #12055, #8498, #16976, #15472, #3243, #22612, #5186, #22492, #18710, #6566, #13527, #3122 ) ),
 .UNSPECIFIED., .F., .F., .F.,
 ( 2, 2 ),
 ( 4, 2, 2, 2, 2, 2, 2, 2, 2, 4 ),
 ( 0.000000000000000000, 1.000000000000000000 ),
 ( 0.000000000000000000, 0.002777081730120475617, 0.004165622595180713643, 0.005554163460240951235, 0.006942704325301189694, 0.008331245190361427286, 0.009025515622891545214, 0.009719786055421664878, 0.01041405648795178454, 0.01110832692048190247 ),
 .UNSPECIFIED. ) ;
#12209=AXIS2_PLACEMENT_3D ( 'NONE', #11282, #3035, #20340 ) ;
#12213=CARTESIAN_POINT ( 'NONE',  ( 0.06362111936223997788, 39.99997618853521431, 48.78343666895094088 ) ) ;
#12215=CARTESIAN_POINT ( 'NONE',  ( -42.50000000000000711, -12.00000000000012434, 47.50000000000000711 ) ) ;
#12218=DIRECTION ( 'NONE',  ( 0.000000000000000000, 0.000000000000000000, -1.000000000000000000 ) ) ;
#12222=AXIS2_PLACEMENT_3D ( 'NONE', #18891, #6290, #2975 ) ;
#12223=LINE ( 'NONE', #7302, #21369 ) ;
#12224=CYLINDRICAL_SURFACE ( 'NONE', #4581, 18.00000000000000000 ) ;
#12225=FACE_BOUND ( 'NONE', #4138, .T. ) ;
#12228=VERTEX_POINT ( 'NONE', #12831 ) ;
#12231=CARTESIAN_POINT ( 'NONE',  ( 0.6683989176551251576, -3.155640224521520043, -47.80307817979551288 ) ) ;
#12233=VERTEX_POINT ( 'NONE', #18002 ) ;
#12235=B_SPLINE_CURVE_WITH_KNOTS ( 'NONE', 3,
 ( #3769, #322, #10970, #2265, #5703, #7655, #12452, #1928, #21066, #9028, #12564, #9249, #7312, #14277, #21294, #5583, #16234, #19575, #3883, #10850 ),
 .UNSPECIFIED., .F., .F.,
 ( 4, 2, 2, 2, 2, 2, 2, 2, 2, 4 ),
 ( 0.02328883130680912961, 0.02567687977621935583, 0.02687090401092446373, 0.02806492824562957511, 0.03284102518444999286, 0.03522907365386020867, 0.03761712212327042448, 0.03881114635797552198, 0.04000517059268062642, 0.04239321906209084223 ),
 .UNSPECIFIED. ) ;
#12236=CARTESIAN_POINT ( 'NONE',  ( 5.833333333333328596, 33.81926995981416439, -40.61164310337066041 ) ) ;
#12238=CARTESIAN_POINT ( 'NONE',  ( -18.68837533793345784, 7.522086334128091245, -57.74247137455871126 ) ) ;
#12239=AXIS2_PLACEMENT_3D ( 'NONE', #1998, #9207, #10923 ) ;
#12244=LINE ( 'NONE', #19251, #18897 ) ;
#12245=CARTESIAN_POINT ( 'NONE',  ( 11.38359864655681086, 10.20536502146449109, -44.07478837098130242 ) ) ;
#12247=CARTESIAN_POINT ( 'NONE',  ( -35.00000000000000000, -9.000000000000001776, 1.387778780781445676E-14 ) ) ;
#12249=EDGE_CURVE ( 'NONE', #6323, #6579, #117, .T. ) ;
#12250=EDGE_CURVE ( 'NONE', #12705, #19146, #8903, .T. ) ;
#12253=ORIENTED_EDGE ( 'NONE', *, *, #3080, .T. ) ;
#12255=AXIS2_PLACEMENT_3D ( 'NONE', #18718, #9894, #16883 ) ;
#12259=AXIS2_PLACEMENT_3D ( 'NONE', #22459, #15214, #13717 ) ;
#12265=CARTESIAN_POINT ( 'NONE',  ( 25.99999999999998579, 19.99999999999999645, 105.0000000000000142 ) ) ;
#12272=CARTESIAN_POINT ( 'NONE',  ( 6.426802710256903417, 33.56875711009141838, -41.03786381671498873 ) ) ;
#12275=CARTESIAN_POINT ( 'NONE',  ( -21.20802570598058878, 27.37171784732027291, 58.39394879075536693 ) ) ;
#12277=CARTESIAN_POINT ( 'NONE',  ( -5.833333333333329485, 0.000000000000000000, 40.61164310337067462 ) ) ;
#12281=AXIS2_PLACEMENT_3D ( 'NONE', #10598, #67, #21044 ) ;
#12282=AXIS2_PLACEMENT_3D ( 'NONE', #12435, #3750, #10709 ) ;
#12284=CIRCLE ( 'NONE', #5346, 2.499999999999998668 ) ;
#12285=ORIENTED_EDGE ( 'NONE', *, *, #18744, .F. ) ;
#12287=CIRCLE ( 'NONE', #9369, 60.00000000000000000 ) ;
#12293=CYLINDRICAL_SURFACE ( 'NONE', #4890, 49.99999999999998579 ) ;
#12298=CARTESIAN_POINT ( 'NONE',  ( -2.605854907981514312, 5.225826804957995009, 39.07589943342649974 ) ) ;
#12299=VERTEX_POINT ( 'NONE', #18455 ) ;
#12301=VECTOR ( 'NONE', #12563, 1000.000000000000000 ) ;
#12302=VECTOR ( 'NONE', #17093, 1000.000000000000000 ) ;
#12306=ORIENTED_EDGE ( 'NONE', *, *, #20161, .F. ) ;
#12307=CARTESIAN_POINT ( 'NONE',  ( 5.833333333333338366, 33.81926995981415729, 40.61164310337067462 ) ) ;
#12308=CARTESIAN_POINT ( 'NONE',  ( -8.331955809010628045, 38.18181818181818699, 56.36098470834075158 ) ) ;
#12309=CARTESIAN_POINT ( 'NONE',  ( 35.00000000000058265, 39.97500000000000142, -57.50000000000076028 ) ) ;
#12310=CARTESIAN_POINT ( 'NONE',  ( 17.35828117057767273, 30.07901706855390600, 57.39628071424991873 ) ) ;
#12313=AXIS2_PLACEMENT_3D ( 'NONE', #923, #4256, #14428 ) ;
#12316=ORIENTED_EDGE ( 'NONE', *, *, #18899, .F. ) ;
#12322=CARTESIAN_POINT ( 'NONE',  ( 1.038202552616665164, 39.99359457986729893, 49.52478249909115959 ) ) ;
#12325=CIRCLE ( 'NONE', #2465, 60.00000000000000000 ) ;
#12326=DIRECTION ( 'NONE',  ( 0.000000000000000000, 0.000000000000000000, 1.000000000000000000 ) ) ;
#12328=DIRECTION ( 'NONE',  ( -0.000000000000000000, -1.000000000000000000, -0.000000000000000000 ) ) ;
#12331=CARTESIAN_POINT ( 'NONE',  ( -19.41351212956693573, 24.83257706694780609, 60.47995209899217883 ) ) ;
#12334=CARTESIAN_POINT ( 'NONE',  ( -7.073836202554792507, 38.72384538518738140, 54.13588025449750063 ) ) ;
#12335=DIRECTION ( 'NONE',  ( -0.000000000000000000, 1.000000000000000000, -0.000000000000000000 ) ) ;
#12336=CARTESIAN_POINT ( 'NONE',  ( 90.00000000000000000, 26.00000000000000355, -9.108981535246192915E-16 ) ) ;
#12337=B_SPLINE_CURVE_WITH_KNOTS ( 'NONE', 3,
 ( #15612, #374, #22637, #3714, #8856, #139, #1770, #6929, #15827, #5207, #7365, #21123, #13889, #17670, #7135, #20905, #1981, #17337, #5424, #14102, #1654, #21341, #5526, #19629, #10664, #16065, #12402, #14333, #3937, #1874, #5639, #256, #7252, #8633, #17449, #12183, #8964, #8755, #19185, #13985, #3491, #10450, #19413, #15725, #38, #15944, #10785, #7028, #3820 ),
 .UNSPECIFIED., .F., .F.,
 ( 4, 1, 1, 1, 2, 2, 1, 1, 1, 1, 2, 2, 1, 1, 1, 2, 2, 1, 1, 1, 1, 2, 2, 1, 1, 1, 1, 2, 2, 1, 1, 1, 2, 2, 4 ),
 ( 0.000000000000000000, 0.1249999999999921729, 0.1874999999999877598, 0.2187499999999850953, 0.2343749999999842626, 0.2499999999999834577, 0.3749999999999780731, 0.4374999999999754086, 0.4687499999999746314, 0.4843749999999746314, 0.4921874999999742428, 0.4999999999999739098, 0.5624999999999701350, 0.5937499999999682476, 0.6093749999999673594, 0.6171874999999674705, 0.6249999999999674705, 0.6874999999999683586, 0.7187499999999685807, 0.7343749999999686917, 0.7421874999999690248, 0.7460937499999691358, 0.7499999999999692468, 0.8124999999999739098, 0.8437499999999762412, 0.8593749999999771294, 0.8671874999999773515, 0.8710937499999776845, 0.8749999999999779066, 0.9062499999999816813, 0.9218749999999836797, 0.9296874999999847899, 0.9335937499999855671, 0.9374999999999864553, 1.000000000000000000 ),
 .UNSPECIFIED. ) ;
#12344=CARTESIAN_POINT ( 'NONE',  ( -35.00000000000000000, 25.00000000000000000, 1.387778780781445676E-14 ) ) ;
#12345=VECTOR ( 'NONE', #4752, 1000.000000000000000 ) ;
#12347=DIRECTION ( 'NONE',  ( -0.000000000000000000, -1.000000000000000000, -0.000000000000000000 ) ) ;
#12350=CARTESIAN_POINT ( 'NONE',  ( -14.19004819996300348, 37.38003124960519585, -56.27686160268856952 ) ) ;
#12352=CIRCLE ( 'NONE', #9076, 18.00000000000000000 ) ;
#12356=FACE_BOUND ( 'NONE', #4808, .T. ) ;
#12358=CARTESIAN_POINT ( 'NONE',  ( 11.84669267190943209, 10.76938159504123149, -44.31876460048058419 ) ) ;
#12359=EDGE_CURVE ( 'NONE', #13092, #16803, #6368, .T. ) ;
#12362=DIRECTION ( 'NONE',  ( 0.000000000000000000, -1.000000000000000000, 0.000000000000000000 ) ) ;
#12365=AXIS2_PLACEMENT_3D ( 'NONE', #6354, #6471, #2590 ) ;
#12368=VECTOR ( 'NONE', #9912, 1000.000000000000000 ) ;
#12371=DIRECTION ( 'NONE',  ( 0.000000000000000000, 0.000000000000000000, -1.000000000000000000 ) ) ;
#12372=DIRECTION ( 'NONE',  ( -0.000000000000000000, 1.000000000000000000, -0.000000000000000000 ) ) ;
#12376=CARTESIAN_POINT ( 'NONE',  ( -10.34137811700765397, 39.99999999999997868, 53.75702834151201870 ) ) ;
#12379=DIRECTION ( 'NONE',  ( 0.000000000000000000, 0.000000000000000000, -1.000000000000000000 ) ) ;
#12382=DIRECTION ( 'NONE',  ( 1.224646799147353207E-16, 1.000000000000000000, -0.000000000000000000 ) ) ;
#12383=CARTESIAN_POINT ( 'NONE',  ( -3.801357191711898231, 39.91216781306113859, -51.45795414075008267 ) ) ;
#12387=CARTESIAN_POINT ( 'NONE',  ( -5.042540965661301833, 39.84191928929035242, -52.23966299716700235 ) ) ;
#12389=CARTESIAN_POINT ( 'NONE',  ( -1.387778780781445518E-14, 20.00000000000000355, -105.0000000000000142 ) ) ;
#12390=CARTESIAN_POINT ( 'NONE',  ( -35.00000000000058265, 40.00000000000000711, -55.00000000000076028 ) ) ;
#12396=ADVANCED_FACE ( 'NONE', ( #6310 ), #867, .T. ) ;
#12398=ORIENTED_EDGE ( 'NONE', *, *, #540, .T. ) ;
#12399=CARTESIAN_POINT ( 'NONE',  ( 9.952189117650862116, 40.00000000000000000, -53.64426396172072486 ) ) ;
#12400=CARTESIAN_POINT ( 'NONE',  ( 12.60179598819646429, 38.53795549125497644, 55.66391160832503715 ) ) ;
#12401=CARTESIAN_POINT ( 'NONE',  ( 0.7796804372245736969, 40.00000000000002132, -49.24007646455138598 ) ) ;
#12402=CARTESIAN_POINT ( 'NONE',  ( 7.158017760915646122, 39.99999999999999289, 52.61520709092953041 ) ) ;
#12409=CARTESIAN_POINT ( 'NONE',  ( -18.32709649528716866, 33.00101640267667591, -57.63983358650814637 ) ) ;
#12410=DIRECTION ( 'NONE',  ( 0.000000000000000000, 0.000000000000000000, -1.000000000000000000 ) ) ;
#12411=CARTESIAN_POINT ( 'NONE',  ( 7.545596340795487578, -0.4932457138281565179, 52.99914579202447129 ) ) ;
#12413=CARTESIAN_POINT ( 'NONE',  ( -35.00000000000058265, 39.97500000000000142, -52.50000000000076739 ) ) ;
#12415=CARTESIAN_POINT ( 'NONE',  ( -90.00000000000000000, 39.97500000000000142, -2.500000000000003109 ) ) ;
#12416=CIRCLE ( 'NONE', #14235, 6.499999999999999112 ) ;
#12417=CARTESIAN_POINT ( 'NONE',  ( 17.76477806472427545, 33.73774409952945064, 57.47211831788253278 ) ) ;
#12420=VERTEX_POINT ( 'NONE', #22129 ) ;
#12421=ORIENTED_EDGE ( 'NONE', *, *, #3728, .F. ) ;
#12423=ORIENTED_EDGE ( 'NONE', *, *, #4016, .F. ) ;
#12424=DIRECTION ( 'NONE',  ( -0.000000000000000000, -1.000000000000000000, -0.000000000000000000 ) ) ;
#12426=DIRECTION ( 'NONE',  ( -0.5002637533272169534, 0.000000000000000000, -0.8658730721687594167 ) ) ;
#12430=CARTESIAN_POINT ( 'NONE',  ( 0.2542260610985473956, 39.99961928011452983, 48.93085117298642928 ) ) ;
#12432=CYLINDRICAL_SURFACE ( 'NONE', #10186, 2.500000000000002220 ) ;
#12434=CARTESIAN_POINT ( 'NONE',  ( 42.50000000000000711, -12.00000000000000000, -41.00000000000000000 ) ) ;
#12435=CARTESIAN_POINT ( 'NONE',  ( -35.00000000000000000, -9.000000000000001776, 1.387778780781445676E-14 ) ) ;
#12437=ADVANCED_FACE ( 'NONE', ( #18689 ), #14765, .F. ) ;
#12439=DIRECTION ( 'NONE',  ( 0.000000000000000000, 0.000000000000000000, -1.000000000000000000 ) ) ;
#12443=ORIENTED_EDGE ( 'NONE', *, *, #13091, .F. ) ;
#12446=ORIENTED_EDGE ( 'NONE', *, *, #4292, .T. ) ;
#12447=CARTESIAN_POINT ( 'NONE',  ( 4.842578813366696266, -0.8535550256994554053, -51.47191290771694838 ) ) ;
#12452=CARTESIAN_POINT ( 'NONE',  ( -19.52068517772380574, 15.62943592677016191, 60.50640500721819848 ) ) ;
#12455=ORIENTED_EDGE ( 'NONE', *, *, #8147, .F. ) ;
#12456=DIRECTION ( 'NONE',  ( 0.000000000000000000, 0.000000000000000000, 1.000000000000000000 ) ) ;
#12457=CARTESIAN_POINT ( 'NONE',  ( -5.833333333333341919, 33.81926995981417150, -40.61164310337066041 ) ) ;
#12458=CARTESIAN_POINT ( 'NONE',  ( -35.00000000000058265, 26.00000000000000355, -55.00000000000076028 ) ) ;
#12459=CARTESIAN_POINT ( 'NONE',  ( 14.76055860720887836, 17.30233064284068334, -45.72055682016586076 ) ) ;
#12465=ORIENTED_EDGE ( 'NONE', *, *, #16184, .F. ) ;
#12469=CARTESIAN_POINT ( 'NONE',  ( -1.387778780781445676E-14, 40.00000000000000000, -48.73397172404481381 ) ) ;
#12472=CARTESIAN_POINT ( 'NONE',  ( 90.00000000000000000, 28.00000000000000000, 2.500000000000001332 ) ) ;
#12474=VERTEX_POINT ( 'NONE', #1838 ) ;
#12475=CARTESIAN_POINT ( 'NONE',  ( 42.50000000000000711, -11.97499999999999964, -47.50000000000000000 ) ) ;
#12476=CARTESIAN_POINT ( 'NONE',  ( -8.835430549262724753, 40.00000000000000711, 53.27933386073573985 ) ) ;
#12477=ORIENTED_EDGE ( 'NONE', *, *, #20243, .F. ) ;
#12478=CARTESIAN_POINT ( 'NONE',  ( 25.99999999999998579, 19.99999999999999645, -105.0010000000000048 ) ) ;
#12479=CARTESIAN_POINT ( 'NONE',  ( 16.84758200736122546, 5.154512310752989102, -57.18908790048117652 ) ) ;
#12484=CARTESIAN_POINT ( 'NONE',  ( -6.646840153610217961, 39.71385754597948647, -53.15684335981527653 ) ) ;
#12485=ORIENTED_EDGE ( 'NONE', *, *, #6467, .T. ) ;
#12487=EDGE_CURVE ( 'NONE', #12153, #2477, #18804, .T. ) ;
#12494=ORIENTED_EDGE ( 'NONE', *, *, #17408, .F. ) ;
#12496=ORIENTED_EDGE ( 'NONE', *, *, #5369, .T. ) ;
#12500=CARTESIAN_POINT ( 'NONE',  ( 2.636011669654858558, 39.95887917521793753, -50.67499985581887501 ) ) ;
#12503=DIRECTION ( 'NONE',  ( -0.000000000000000000, -0.000000000000000000, -1.000000000000000000 ) ) ;
#12505=EDGE_LOOP ( 'NONE', ( #1655, #8126, #21738, #14212 ) ) ;
#12506=CARTESIAN_POINT ( 'NONE',  ( -0.6814780602828901523, -1.267001069680700365, 48.72478509528001922 ) ) ;
#12509=ORIENTED_EDGE ( 'NONE', *, *, #14724, .T. ) ;
#12513=CARTESIAN_POINT ( 'NONE',  ( -6.775203351379203376, 38.82189279864962117, 55.41163305959242535 ) ) ;
#12517=ADVANCED_FACE ( 'NONE', ( #10407 ), #18059, .T. ) ;
#12518=CARTESIAN_POINT ( 'NONE',  ( 19.88513910325152523, 17.69449494136076950, 58.11726460477455447 ) ) ;
#12520=AXIS2_PLACEMENT_3D ( 'NONE', #9248, #3882, #10729 ) ;
#12527=EDGE_CURVE ( 'NONE', #3040, #3905, #20520, .T. ) ;
#12531=DIRECTION ( 'NONE',  ( -0.000000000000000000, 1.000000000000000000, -0.000000000000000000 ) ) ;
#12536=CARTESIAN_POINT ( 'NONE',  ( 0.4769526114005525619, 39.99865964525184125, 49.10162959029930363 ) ) ;
#12541=CARTESIAN_POINT ( 'NONE',  ( 35.00000000000058265, 26.00000000000000355, -57.10000000000076170 ) ) ;
#12543=FACE_OUTER_BOUND ( 'NONE', #11740, .T. ) ;
#12544=CARTESIAN_POINT ( 'NONE',  ( -1.387778780781445518E-14, 20.00000000000000355, 102.0000000000000142 ) ) ;
#12545=CARTESIAN_POINT ( 'NONE',  ( -35.00000000000000000, -9.000000000000001776, 18.00000000000001421 ) ) ;
#12550=DIRECTION ( 'NONE',  ( 0.000000000000000000, 0.000000000000000000, -1.000000000000000000 ) ) ;
#12556=ORIENTED_EDGE ( 'NONE', *, *, #5405, .F. ) ;
#12558=CARTESIAN_POINT ( 'NONE',  ( 12.15643230334913660, 40.00000000000000711, -54.39836425128640940 ) ) ;
#12562=EDGE_CURVE ( 'NONE', #17863, #18194, #21005, .T. ) ;
#12563=DIRECTION ( 'NONE',  ( 0.7071067811865426878, 0.000000000000000000, 0.7071067811865524577 ) ) ;
#12564=CARTESIAN_POINT ( 'NONE',  ( -16.97539716422060962, 9.395639044392956052, 59.81372721910508972 ) ) ;
#12565=CARTESIAN_POINT ( 'NONE',  ( -15.91596560756144996, 32.12719615765574588, -56.91747558600052059 ) ) ;
#12567=VECTOR ( 'NONE', #10963, 1000.000000000000000 ) ;
#12570=B_SPLINE_CURVE_WITH_KNOTS ( 'NONE', 3,
 ( #1174, #15023, #952, #16647, #9775, #7948, #6229, #13294, #14909, #16877, #22041, #18361, #2681, #21935, #6334, #13189, #20324, #1075 ),
 .UNSPECIFIED., .F., .F.,
 ( 4, 2, 2, 2, 2, 2, 2, 2, 4 ),
 ( -3.543127106801270167E-05, 0.0006851204654910545561, 0.001405672202050121814, 0.002846775675168256546, 0.005728982621404526444, 0.007170086094522653587, 0.008611189567640779863, 0.01005229304075890701, 0.01149339651387703241 ),
 .UNSPECIFIED. ) ;
#12572=DIRECTION ( 'NONE',  ( 1.000000000000000000, 0.000000000000000000, -1.224646799147353207E-16 ) ) ;
#12573=ORIENTED_EDGE ( 'NONE', *, *, #20055, .F. ) ;
#12575=FACE_OUTER_BOUND ( 'NONE', #3067, .T. ) ;
#12576=CARTESIAN_POINT ( 'NONE',  ( -1.387778780781445676E-14, 20.00000000000000000, -102.0000000000000142 ) ) ;
#12579=VERTEX_POINT ( 'NONE', #1723 ) ;
#12581=ORIENTED_EDGE ( 'NONE', *, *, #3412, .F. ) ;
#12584=CARTESIAN_POINT ( 'NONE',  ( -18.00000000000001421, 20.00000000000000355, -105.0000000000000142 ) ) ;
#12587=CARTESIAN_POINT ( 'NONE',  ( -1.387778780781445518E-14, 20.00000000000000355, 102.0000000000000142 ) ) ;
#12591=DIRECTION ( 'NONE',  ( 0.000000000000000000, -1.000000000000000000, 0.000000000000000000 ) ) ;
#12594=CARTESIAN_POINT ( 'NONE',  ( -35.00000000000000000, 2.142135623730931471, -49.99999999999998579 ) ) ;
#12596=LINE ( 'NONE', #19841, #154 ) ;
#12597=CARTESIAN_POINT ( 'NONE',  ( -5.466611548547432697, 39.81233001754419121, -52.49274982270507195 ) ) ;
#12600=DIRECTION ( 'NONE',  ( 1.000000000000000000, 0.000000000000000000, 0.000000000000000000 ) ) ;
#12602=CARTESIAN_POINT ( 'NONE',  ( -1.243967489023287243, -3.506377588453899790E-14, 51.43875557960417666 ) ) ;
#12605=AXIS2_PLACEMENT_3D ( 'NONE', #18149, #2686, #2462 ) ;
#12611=DIRECTION ( 'NONE',  ( 1.000000000000000000, 0.000000000000000000, 0.000000000000000000 ) ) ;
#12615=EDGE_LOOP ( 'NONE', ( #9984, #5592, #5171, #18005 ) ) ;
#12618=EDGE_LOOP ( 'NONE', ( #10608, #17915, #2412, #18713 ) ) ;
#12620=CARTESIAN_POINT ( 'NONE',  ( -22.41556111754674063, 20.62010838399689305, -58.66542762804073163 ) ) ;
#12622=ORIENTED_EDGE ( 'NONE', *, *, #19638, .T. ) ;
#12623=CARTESIAN_POINT ( 'NONE',  ( 2.517875701374014508, 0.1458803431926766758, 52.33410116371960896 ) ) ;
#12627=ADVANCED_FACE ( 'NONE', ( #12575 ), #7094, .T. ) ;
#12629=DIRECTION ( 'NONE',  ( -1.000000000000000000, 0.000000000000000000, 0.000000000000000000 ) ) ;
#12630=CARTESIAN_POINT ( 'NONE',  ( 1.247275002120749043, 0.02903096490061087345, 51.42826582519167999 ) ) ;
#12631=AXIS2_PLACEMENT_3D ( 'NONE', #20011, #18285, #2363 ) ;
#12633=CARTESIAN_POINT ( 'NONE',  ( 21.72501817863376061, 25.59362490671916390, 58.51313831023582424 ) ) ;
#12634=DIRECTION ( 'NONE',  ( -0.000000000000000000, 1.000000000000000000, -0.000000000000000000 ) ) ;
#12635=EDGE_CURVE ( 'NONE', #9318, #18860, #7453, .T. ) ;
#12636=CIRCLE ( 'NONE', #3140, 2.499999999999995115 ) ;
#12637=FACE_OUTER_BOUND ( 'NONE', #8812, .T. ) ;
#12638=ORIENTED_EDGE ( 'NONE', *, *, #8578, .F. ) ;
#12640=( BOUNDED_SURFACE ( )  B_SPLINE_SURFACE ( 3, 2, ( 
 ( #7499, #3842, #5662 ),
 ( #18267, #2117, #2578 ),
 ( #7727, #9108, #19654 ),
 ( #3960, #10928, #14472 ),
 ( #4075, #14698, #21708 ),
 ( #13307, #18721, #11386 ),
 ( #15031, #20448, #15375 ),
 ( #4857, #2804, #13537 ),
 ( #10109, #9897, #16885 ),
 ( #1182, #21946, #3136 ),
 ( #4639, #1417, #11726 ),
 ( #18613, #8292, #11504 ),
 ( #22163, #3025, #11828 ),
 ( #1084, #6462, #9994 ),
 ( #9783, #18372, #15143 ),
 ( #22284, #8179, #16657 ),
 ( #16778, #6344, #8074 ),
 ( #964, #22050, #18831 ),
 ( #22392, #13423, #20218 ),
 ( #4755, #16988, #1296 ),
 ( #20332, #13090, #7959 ),
 ( #14923, #15260, #17101 ),
 ( #6577, #8403, #2690 ),
 ( #9669, #20555, #6239 ),
 ( #11615, #20107, #4413 ),
 ( #2923, #13197, #4522 ),
 ( #18489, #14293, #9269 ),
 ( #21416, #19059, #7435 ),
 ( #4020, #3781, #10744 ),
 ( #4967, #12694, #11950 ),
 ( #18948, #15599, #16130 ),
 ( #22504, #19715, #17748 ) ),
 .UNSPECIFIED., .F., .F., .F. ) 
 B_SPLINE_SURFACE_WITH_KNOTS ( ( 4, 2, 2, 2, 2, 2, 2, 2, 2, 2, 2, 2, 2, 2, 2, 4 ),
 ( 3, 3 ),
 ( 0.000000000000000000, 0.005810029919203046553, 0.008715044878804568962, 0.01162005983840609311, 0.01452507479800761551, 0.01743008975760913792, 0.02033510471721066207, 0.02324011967681218621, 0.02614513463641370689, 0.02905014959601523103, 0.03486017951521827585, 0.03631268699501903618, 0.03776519447481979652, 0.04067020943442132414, 0.04357522439402285175, 0.04648023935362437242 ),
 ( 0.000000000000000000, 1.000000000000000000 ),
 .UNSPECIFIED. ) 
 GEOMETRIC_REPRESENTATION_ITEM ( )  RATIONAL_B_SPLINE_SURFACE ( (
 ( 1.000000000000000000, 0.6428092274089103331, 1.000000000000000000),
 ( 1.000000000000000000, 0.6349692141176793703, 1.000000000000000000),
 ( 1.000000000000000000, 0.6297610438357627016, 1.000000000000000000),
 ( 1.000000000000000000, 0.6250724677584068578, 1.000000000000000000),
 ( 1.000000000000000000, 0.6240291009521173882, 1.000000000000000000),
 ( 1.000000000000000000, 0.6228114827670524489, 1.000000000000000000),
 ( 1.000000000000000000, 0.6226217323249612079, 1.000000000000000000),
 ( 1.000000000000000000, 0.6227877533346650729, 1.000000000000000000),
 ( 1.000000000000000000, 0.6231437405070447966, 1.000000000000000000),
 ( 1.000000000000000000, 0.6241327156850213775, 1.000000000000000000),
 ( 1.000000000000000000, 0.6247528374326117850, 1.000000000000000000),
 ( 1.000000000000000000, 0.6259854008239856826, 1.000000000000000000),
 ( 1.000000000000000000, 0.6265990906519964820, 1.000000000000000000),
 ( 1.000000000000000000, 0.6276348137186016363, 1.000000000000000000),
 ( 1.000000000000000000, 0.6280565648738838380, 1.000000000000000000),
 ( 1.000000000000000000, 0.6285705475686420574, 1.000000000000000000),
 ( 1.000000000000000000, 0.6286676444210588244, 1.000000000000000000),
 ( 1.000000000000000000, 0.6285219413506923924, 1.000000000000000000),
 ( 1.000000000000000000, 0.6282782847648648028, 1.000000000000000000),
 ( 1.000000000000000000, 0.6271139948487377547, 1.000000000000000000),
 ( 1.000000000000000000, 0.6257653971627769041, 1.000000000000000000),
 ( 1.000000000000000000, 0.6242767683747761920, 1.000000000000000000),
 ( 1.000000000000000000, 0.6239908339052062658, 1.000000000000000000),
 ( 1.000000000000000000, 0.6234800620773224278, 1.000000000000000000),
 ( 1.000000000000000000, 0.6232570855785173336, 1.000000000000000000),
 ( 1.000000000000000000, 0.6227348070526912416, 1.000000000000000000),
 ( 1.000000000000000000, 0.6225812994807357059, 1.000000000000000000),
 ( 1.000000000000000000, 0.6229454059011351186, 1.000000000000000000),
 ( 1.000000000000000000, 0.6234652178689191748, 1.000000000000000000),
 ( 1.000000000000000000, 0.6254772350198137820, 1.000000000000000000),
 ( 1.000000000000000000, 0.6269570472270592498, 1.000000000000000000),
 ( 1.000000000000000000, 0.6290213284793358950, 1.000000000000000000) ) ) 
 REPRESENTATION_ITEM ( '' )  SURFACE ( )  );
#12642=CONICAL_SURFACE ( 'NONE', #201, 2.099999999999990763, 1.029744258676652091 ) ;
#12644=CYLINDRICAL_SURFACE ( 'NONE', #442, 6.499999999999999112 ) ;
#12645=CARTESIAN_POINT ( 'NONE',  ( -42.50000000000000711, -5.000000000000000000, 47.50000000000000711 ) ) ;
#12648=ADVANCED_FACE ( 'NONE', ( #14526 ), #19903, .T. ) ;
#12653=ORIENTED_EDGE ( 'NONE', *, *, #13130, .T. ) ;
#12656=EDGE_CURVE ( 'NONE', #7389, #1702, #12931, .T. ) ;
#12657=DIRECTION ( 'NONE',  ( -0.000000000000000000, 1.000000000000000000, -0.000000000000000000 ) ) ;
#12658=CARTESIAN_POINT ( 'NONE',  ( -19.98183132229268466, 20.98212305896295504, -60.61750244562276890 ) ) ;
#12661=VECTOR ( 'NONE', #3064, 1000.000000000000000 ) ;
#12663=LINE ( 'NONE', #9479, #11489 ) ;
#12667=CIRCLE ( 'NONE', #6838, 10.00000000000000178 ) ;
#12668=ORIENTED_EDGE ( 'NONE', *, *, #6519, .T. ) ;
#12669=ORIENTED_EDGE ( 'NONE', *, *, #1320, .F. ) ;
#12672=DIRECTION ( 'NONE',  ( 0.000000000000000000, -0.000000000000000000, -1.000000000000000000 ) ) ;
#12676=FACE_OUTER_BOUND ( 'NONE', #14268, .T. ) ;
#12677=CARTESIAN_POINT ( 'NONE',  ( -9.081037608035938291, 37.83854577724346768, -56.73868670302932316 ) ) ;
#12679=CIRCLE ( 'NONE', #18869, 2.499999999999998668 ) ;
#12680=VERTEX_POINT ( 'NONE', #1939 ) ;
#12681=LINE ( 'NONE', #17856, #14142 ) ;
#12682=CARTESIAN_POINT ( 'NONE',  ( -42.50000000000000711, -12.00000000000000000, -45.00000000000000000 ) ) ;
#12686=EDGE_CURVE ( 'NONE', #22510, #15748, #14060, .T. ) ;
#12687=ORIENTED_EDGE ( 'NONE', *, *, #16315, .F. ) ;
#12691=AXIS2_PLACEMENT_3D ( 'NONE', #2216, #16296, #607 ) ;
#12692=DIRECTION ( 'NONE',  ( 0.000000000000000000, -0.000000000000000000, -1.000000000000000000 ) ) ;
#12694=CARTESIAN_POINT ( 'NONE',  ( 13.52717286024270216, 5.231573370292008640, -56.05142967219527605 ) ) ;
#12704=CIRCLE ( 'NONE', #2858, 2.500000000000002220 ) ;
#12705=VERTEX_POINT ( 'NONE', #16129 ) ;
#12707=CARTESIAN_POINT ( 'NONE',  ( -9.433062738409624615, 40.00000000000000711, 53.48670742531720634 ) ) ;
#12710=CARTESIAN_POINT ( 'NONE',  ( -22.00000000000001421, 20.00000000000000000, -98.00000000000000000 ) ) ;
#12711=CIRCLE ( 'NONE', #7227, 2.524999999999999467 ) ;
#12714=EDGE_LOOP ( 'NONE', ( #9891, #12909 ) ) ;
#12715=CARTESIAN_POINT ( 'NONE',  ( -35.00000000000000000, -4.999999999999997335, 1.387778780781445676E-14 ) ) ;
#12718=ADVANCED_FACE ( 'NONE', ( #21193 ), #10466, .F. ) ;
#12721=CARTESIAN_POINT ( 'NONE',  ( -12.48541242016036179, 28.32175387455462712, 44.64471390988171606 ) ) ;
#12725=EDGE_CURVE ( 'NONE', #11771, #11765, #19992, .T. ) ;
#12726=VECTOR ( 'NONE', #7854, 1000.000000000000000 ) ;
#12727=VECTOR ( 'NONE', #13281, 1000.000000000000000 ) ;
#12729=ORIENTED_EDGE ( 'NONE', *, *, #13506, .F. ) ;
#12730=EDGE_LOOP ( 'NONE', ( #16929, #5552, #8043, #8269 ) ) ;
#12732=ADVANCED_FACE ( 'NONE', ( #21304, #16249 ), #16021, .F. ) ;
#12735=CARTESIAN_POINT ( 'NONE',  ( 2.777950727038989154, 39.99999999999999289, -50.42550754305786853 ) ) ;
#12738=ORIENTED_EDGE ( 'NONE', *, *, #19008, .F. ) ;
#12744=CIRCLE ( 'NONE', #21543, 2.099999999999997868 ) ;
#12745=EDGE_CURVE ( 'NONE', #6428, #16050, #3542, .T. ) ;
#12751=CARTESIAN_POINT ( 'NONE',  ( 5.133442403747772609, 39.34078726959584316, 53.02546941656563462 ) ) ;
#12754=CYLINDRICAL_SURFACE ( 'NONE', #4523, 60.00000000000000000 ) ;
#12756=CARTESIAN_POINT ( 'NONE',  ( 21.22368364729369361, 12.66551901741837405, 58.39771426751187278 ) ) ;
#12757=DIRECTION ( 'NONE',  ( -1.000000000000000000, 0.000000000000000000, 0.000000000000000000 ) ) ;
#12758=FACE_BOUND ( 'NONE', #15467, .T. ) ;
#12760=ORIENTED_EDGE ( 'NONE', *, *, #10857, .F. ) ;
#12767=CARTESIAN_POINT ( 'NONE',  ( -11.25639079541607934, 39.09917355307971576, -55.11545576720666162 ) ) ;
#12768=FACE_OUTER_BOUND ( 'NONE', #22663, .T. ) ;
#12770=CARTESIAN_POINT ( 'NONE',  ( -0.7809641287213069383, -4.625293788889051072, 46.06432795380178646 ) ) ;
#12774=DIRECTION ( 'NONE',  ( 0.000000000000000000, 0.000000000000000000, 1.000000000000000000 ) ) ;
#12775=CARTESIAN_POINT ( 'NONE',  ( -42.50000000000000711, -12.00000000000000000, 47.50000000000000711 ) ) ;
#12779=CARTESIAN_POINT ( 'NONE',  ( -1.485790755603442514E-14, 40.00000000000000000, 48.73397172404484223 ) ) ;
#12780=EDGE_CURVE ( 'NONE', #10746, #22194, #9739, .T. ) ;
#12781=( BOUNDED_SURFACE ( )  B_SPLINE_SURFACE ( 3, 2, ( 
 ( #5320, #19304, #10236 ),
 ( #17229, #1542, #14108 ),
 ( #17571, #22521, #8639 ),
 ( #20911, #13780, #486 ),
 ( #17796, #21346, #21463 ),
 ( #18135, #5766, #8969 ),
 ( #9434, #16175, #12506 ),
 ( #7483, #15951, #19757 ) ),
 .UNSPECIFIED., .F., .F., .F. ) 
 B_SPLINE_SURFACE_WITH_KNOTS ( ( 4, 2, 2, 4 ),
 ( 3, 3 ),
 ( 0.000000000000000000, 0.005621242337451588626, 0.008431863506177382506, 0.01124248467490317725 ),
 ( 0.000000000000000000, 1.000000000000000000 ),
 .UNSPECIFIED. ) 
 GEOMETRIC_REPRESENTATION_ITEM ( )  RATIONAL_B_SPLINE_SURFACE ( (
 ( 1.000000000000000000, 0.7200096751079151369, 1.000000000000000000),
 ( 1.000000000000000000, 0.7496970740839632441, 1.000000000000000000),
 ( 1.000000000000000000, 0.7737958965667965927, 1.000000000000000000),
 ( 1.000000000000000000, 0.8024469391899264892, 1.000000000000000000),
 ( 1.000000000000000000, 0.8107372619350866616, 1.000000000000000000),
 ( 1.000000000000000000, 0.8249110457735379098, 1.000000000000000000),
 ( 1.000000000000000000, 0.8307983230915116923, 1.000000000000000000),
 ( 1.000000000000000000, 0.8354958991656090683, 1.000000000000000000) ) ) 
 REPRESENTATION_ITEM ( '' )  SURFACE ( )  );
#12786=EDGE_CURVE ( 'NONE', #20078, #15733, #6826, .T. ) ;
#12790=CARTESIAN_POINT ( 'NONE',  ( 7.538500903810520626, 38.52938254314626221, 55.92181088654620424 ) ) ;
#12792=CARTESIAN_POINT ( 'NONE',  ( -10.88890858922316163, 36.78121034548709645, -57.56873443368869658 ) ) ;
#12795=ORIENTED_EDGE ( 'NONE', *, *, #13335, .T. ) ;
#12796=DIRECTION ( 'NONE',  ( -0.000000000000000000, 1.000000000000000000, -0.000000000000000000 ) ) ;
#12803=EDGE_CURVE ( 'NONE', #19609, #13854, #4234, .T. ) ;
#12808=ORIENTED_EDGE ( 'NONE', *, *, #14311, .F. ) ;
#12810=CARTESIAN_POINT ( 'NONE',  ( 5.553314835777164227, 39.99999999999998579, -51.88330480362772335 ) ) ;
#12813=CARTESIAN_POINT ( 'NONE',  ( 4.557463200991922037, 39.87073523829934629, -51.93758469931694322 ) ) ;
#12817=EDGE_LOOP ( 'NONE', ( #5150, #18723 ) ) ;
#12819=DIRECTION ( 'NONE',  ( 1.000000000000000000, 0.000000000000000000, 0.000000000000000000 ) ) ;
#12821=CARTESIAN_POINT ( 'NONE',  ( 35.00000000000000711, 0.000000000000000000, 49.99999999999999289 ) ) ;
#12822=FACE_OUTER_BOUND ( 'NONE', #9309, .T. ) ;
#12823=CARTESIAN_POINT ( 'NONE',  ( -8.194244601622644453, 39.99999999999999289, 53.04029799712058235 ) ) ;
#12824=AXIS2_PLACEMENT_3D ( 'NONE', #8520, #19184, #19069 ) ;
#12825=CARTESIAN_POINT ( 'NONE',  ( 42.50000000000000711, -5.000000000000000000, -47.50000000000000000 ) ) ;
#12830=CARTESIAN_POINT ( 'NONE',  ( -12.68897045256290035, 28.00829229206842896, 44.74667050109238886 ) ) ;
#12831=CARTESIAN_POINT ( 'NONE',  ( 13.56354382738800268, 2.142135623730931471, 56.03997097393685323 ) ) ;
#12841=CARTESIAN_POINT ( 'NONE',  ( 3.182708703124521588, 40.00000000000000711, -50.65274029778007048 ) ) ;
#12842=ADVANCED_FACE ( 'NONE', ( #13145 ), #18316, .F. ) ;
#12850=CARTESIAN_POINT ( 'NONE',  ( -17.68664055422813774, 6.162676607241205140, -57.44855069909471013 ) ) ;
#12851=CIRCLE ( 'NONE', #9933, 2.500000000000002220 ) ;
#12853=ORIENTED_EDGE ( 'NONE', *, *, #11414, .T. ) ;
#12857=CARTESIAN_POINT ( 'NONE',  ( 1.268121568163981028, 39.97056933375354504, 50.22305475356784399 ) ) ;
#12860=ORIENTED_EDGE ( 'NONE', *, *, #11175, .F. ) ;
#12862=PLANE ( 'NONE',  #12605 ) ;
#12863=CARTESIAN_POINT ( 'NONE',  ( 15.50000000000024336, -2.516660498395250301, 60.00099999999999767 ) ) ;
#12867=CIRCLE ( 'NONE', #13221, 10.00000000000000355 ) ;
#12870=ORIENTED_EDGE ( 'NONE', *, *, #6949, .T. ) ;
#12876=CARTESIAN_POINT ( 'NONE',  ( 1.387778780781445676E-14, 40.00000000000000000, 48.73397172404482802 ) ) ;
#12880=CYLINDRICAL_SURFACE ( 'NONE', #12631, 60.00000000000000000 ) ;
#12881=CARTESIAN_POINT ( 'NONE',  ( -35.00000000000000000, 25.00000000000000000, -8.999999999999989342 ) ) ;
#12883=VECTOR ( 'NONE', #7967, 1000.000000000000000 ) ;
#12884=CARTESIAN_POINT ( 'NONE',  ( -20.00000000000001421, 20.00000000000000355, -105.0020000000000095 ) ) ;
#12888=FACE_OUTER_BOUND ( 'NONE', #367, .T. ) ;
#12896=CARTESIAN_POINT ( 'NONE',  ( -42.50000000000000711, -9.600000000000001421, -49.60000000000000142 ) ) ;
#12897=AXIS2_PLACEMENT_3D ( 'NONE', #11154, #12634, #11040 ) ;
#12900=CARTESIAN_POINT ( 'NONE',  ( -8.619968867809234325, 38.06589896304013365, -54.65505050754611460 ) ) ;
#12901=DIRECTION ( 'NONE',  ( -0.000000000000000000, -1.000000000000000000, -0.000000000000000000 ) ) ;
#12904=CARTESIAN_POINT ( 'NONE',  ( 34.99999999999980815, 28.00000000000000000, 54.99999999999922551 ) ) ;
#12905=DIRECTION ( 'NONE',  ( -1.000000000000000000, 0.000000000000000000, 0.000000000000000000 ) ) ;
#12909=ORIENTED_EDGE ( 'NONE', *, *, #18855, .F. ) ;
#12910=CARTESIAN_POINT ( 'NONE',  ( 5.833333333333339255, 0.000000000000000000, 40.61164310337067462 ) ) ;
#12911=CIRCLE ( 'NONE', #7431, 2.499999999999996891 ) ;
#12912=FACE_OUTER_BOUND ( 'NONE', #19307, .T. ) ;
#12915=AXIS2_PLACEMENT_3D ( 'NONE', #18685, #18792, #6539 ) ;
#12917=ORIENTED_EDGE ( 'NONE', *, *, #871, .F. ) ;
#12919=AXIS2_PLACEMENT_3D ( 'NONE', #21389, #4324, #2488 ) ;
#12920=CARTESIAN_POINT ( 'NONE',  ( 2.734686107766180818, 40.00000000000000000, -50.39884022139948172 ) ) ;
#12922=CARTESIAN_POINT ( 'NONE',  ( 1.109394314766096068, 39.99267486917625547, -49.57771226710639212 ) ) ;
#12924=AXIS2_PLACEMENT_3D ( 'NONE', #18728, #9792, #10004 ) ;
#12927=LINE ( 'NONE', #11343, #15083 ) ;
#12928=CARTESIAN_POINT ( 'NONE',  ( -6.257499475795364141, 39.99999999999999289, 52.21447189357184726 ) ) ;
#12930=CARTESIAN_POINT ( 'NONE',  ( -11.68090480754633553, 3.765577839755393619, -57.90797000640142045 ) ) ;
#12931=CIRCLE ( 'NONE', #3076, 2.000000000000000444 ) ;
#12932=CARTESIAN_POINT ( 'NONE',  ( -6.488130988471835892, 39.99999999999999289, 52.32258080686172264 ) ) ;
#12935=DIRECTION ( 'NONE',  ( 0.000000000000000000, -1.000000000000000000, 0.000000000000000000 ) ) ;
#12936=CARTESIAN_POINT ( 'NONE',  ( -11.68987541779232764, 3.735186999639990013, 55.40064774141873016 ) ) ;
#12940=ADVANCED_FACE ( 'NONE', ( #5247, #15315, #1233, #18769, #3418, #12225, #6738, #19226 ), #20719, .T. ) ;
#12941=ORIENTED_EDGE ( 'NONE', *, *, #17816, .T. ) ;
#12949=ORIENTED_EDGE ( 'NONE', *, *, #6806, .T. ) ;
#12950=ORIENTED_EDGE ( 'NONE', *, *, #12249, .T. ) ;
#12952=VERTEX_POINT ( 'NONE', #4908 ) ;
#12953=CARTESIAN_POINT ( 'NONE',  ( 15.27654436812519023, 32.91718622474422773, 59.27094897435730303 ) ) ;
#12959=FACE_OUTER_BOUND ( 'NONE', #5772, .T. ) ;
#12965=CARTESIAN_POINT ( 'NONE',  ( -21.90353326617357510, 15.16496266307569130, -58.55331524747136029 ) ) ;
#12966=DIRECTION ( 'NONE',  ( -0.000000000000000000, -1.000000000000000000, -0.000000000000000000 ) ) ;
#12968=LINE ( 'NONE', #3644, #11940 ) ;
#12971=CARTESIAN_POINT ( 'NONE',  ( -42.50000000000000711, -5.000000000000000000, -49.60000000000000142 ) ) ;
#12972=CARTESIAN_POINT ( 'NONE',  ( -9.103081159019568602, 0.03030367950605257835, -53.87333532811887693 ) ) ;
#12975=CARTESIAN_POINT ( 'NONE',  ( 9.814839119318500948, 37.44644195123049002, 57.08682537453372419 ) ) ;
#12976=CARTESIAN_POINT ( 'NONE',  ( 42.50000000000000711, -12.00000000000000000, 50.00000000000000711 ) ) ;
#12978=EDGE_CURVE ( 'NONE', #11729, #12233, #17412, .T. ) ;
#12979=EDGE_CURVE ( 'NONE', #10389, #15662, #3139, .T. ) ;
#12981=EDGE_LOOP ( 'NONE', ( #10225, #112, #8752, #5519 ) ) ;
#12988=EDGE_LOOP ( 'NONE', ( #19710, #2550, #19262, #5989 ) ) ;
#12991=EDGE_LOOP ( 'NONE', ( #4868, #19259, #13577, #4840 ) ) ;
#12994=DIRECTION ( 'NONE',  ( 0.000000000000000000, 0.000000000000000000, -1.000000000000000000 ) ) ;
#12998=CARTESIAN_POINT ( 'NONE',  ( -1.387778780781445518E-14, 20.00000000000000355, -102.0000000000000142 ) ) ;
#13000=AXIS2_PLACEMENT_3D ( 'NONE', #12390, #2196, #19398 ) ;
#13007=EDGE_CURVE ( 'NONE', #10753, #9264, #15935, .T. ) ;
#13009=CARTESIAN_POINT ( 'NONE',  ( 1.575352350796998202, 39.94051438458651404, 50.55779643183549155 ) ) ;
#13011=AXIS2_PLACEMENT_3D ( 'NONE', #20828, #10371, #17029 ) ;
#13012=CARTESIAN_POINT ( 'NONE',  ( 5.816608766681834908, -4.770324936805408811, 49.23968220743229551 ) ) ;
#13018=ORIENTED_EDGE ( 'NONE', *, *, #22202, .T. ) ;
#13024=EDGE_LOOP ( 'NONE', ( #2299, #1092 ) ) ;
#13025=DIRECTION ( 'NONE',  ( 0.000000000000000000, -0.000000000000000000, -1.000000000000000000 ) ) ;
#13030=B_SPLINE_CURVE_WITH_KNOTS ( 'NONE', 1,
 ( #22117, #2981 ),
 .UNSPECIFIED., .F., .F.,
 ( 2, 2 ),
 ( 0.000000000000000000, 1.000000000000000000 ),
 .UNSPECIFIED. ) ;
#13031=CARTESIAN_POINT ( 'NONE',  ( 6.445000816259396359, 40.00000000000000000, -52.30046220936269918 ) ) ;
#13034=CARTESIAN_POINT ( 'NONE',  ( 4.517337970793025015, 39.87308997424864287, -51.91252392995636455 ) ) ;
#13036=CARTESIAN_POINT ( 'NONE',  ( 11.86180952233168995, 38.99999999999999289, 55.35904751184886408 ) ) ;
#13040=FACE_OUTER_BOUND ( 'NONE', #16649, .T. ) ;
#13041=EDGE_CURVE ( 'NONE', #15736, #10123, #22198, .T. ) ;
#13042=CARTESIAN_POINT ( 'NONE',  ( 34.99999999999980815, 28.00000000000000000, 54.99999999999922551 ) ) ;
#13044=DIRECTION ( 'NONE',  ( -0.000000000000000000, -0.000000000000000000, 1.000000000000000000 ) ) ;
#13045=AXIS2_PLACEMENT_3D ( 'NONE', #21556, #2186, #12379 ) ;
#13047=CYLINDRICAL_SURFACE ( 'NONE', #17323, 2.499999999999998668 ) ;
#13048=CONICAL_SURFACE ( 'NONE', #9044, 2.525000000000110489, 0.7853981633971014453 ) ;
#13050=CARTESIAN_POINT ( 'NONE',  ( 9.744263423230279386, 2.495070046657416718, 54.63687069583267686 ) ) ;
#13051=CARTESIAN_POINT ( 'NONE',  ( -11.38359864655678244, 29.79463497853559417, 44.07478837098130953 ) ) ;
#13054=ORIENTED_EDGE ( 'NONE', *, *, #7770, .F. ) ;
#13060=AXIS2_PLACEMENT_3D ( 'NONE', #8688, #20953, #5257 ) ;
#13062=CARTESIAN_POINT ( 'NONE',  ( 11.49399598612405349, 36.39311532300401097, 57.83624353974210663 ) ) ;
#13063=CARTESIAN_POINT ( 'NONE',  ( 9.079900084790089920, 0.2952492082894785375, 53.92155889450688733 ) ) ;
#13066=CARTESIAN_POINT ( 'NONE',  ( 28.49999999999998224, 19.99999999999999645, -105.0010000000000048 ) ) ;
#13070=EDGE_LOOP ( 'NONE', ( #21484, #3718, #7304, #13771 ) ) ;
#13075=CARTESIAN_POINT ( 'NONE',  ( 35.00000000000058265, 26.00000000000000355, -55.00000000000076028 ) ) ;
#13079=CARTESIAN_POINT ( 'NONE',  ( -1.609530493688067216E-14, 40.00000000000000000, 48.73397172404481381 ) ) ;
#13080=EDGE_CURVE ( 'NONE', #14603, #4801, #19290, .T. ) ;
#13081=CARTESIAN_POINT ( 'NONE',  ( -4.529250793106221700E-15, -0.2027636850925037537, -49.39727160457752575 ) ) ;
#13082=ORIENTED_EDGE ( 'NONE', *, *, #14888, .T. ) ;
#13086=CARTESIAN_POINT ( 'NONE',  ( 90.00000000000000000, 40.00000000000000000, -2.500000000000003109 ) ) ;
#13088=CIRCLE ( 'NONE', #5439, 2.500000000000002220 ) ;
#13090=CARTESIAN_POINT ( 'NONE',  ( 18.99835506942486418, 13.52193747355529219, -57.87905887291312723 ) ) ;
#13091=EDGE_CURVE ( 'NONE', #19599, #22642, #8661, .T. ) ;
#13092=VERTEX_POINT ( 'NONE', #7303 ) ;
#13095=EDGE_LOOP ( 'NONE', ( #1950, #19384, #20677, #13832 ) ) ;
#13096=ADVANCED_FACE ( 'NONE', ( #2147 ), #9015, .T. ) ;
#13098=DIRECTION ( 'NONE',  ( -0.000000000000000000, -1.000000000000000000, -0.000000000000000000 ) ) ;
#13101=CONICAL_SURFACE ( 'NONE', #3253, 57.00000000000002132, 0.7853981633974437271 ) ;
#13103=VERTEX_POINT ( 'NONE', #9236 ) ;
#13106=ORIENTED_EDGE ( 'NONE', *, *, #2825, .F. ) ;
#13114=CARTESIAN_POINT ( 'NONE',  ( -17.23507576850067835, 30.19164414353179637, -59.89185441256821463 ) ) ;
#13117=AXIS2_PLACEMENT_3D ( 'NONE', #12048, #13742, #5072 ) ;
#13118=CARTESIAN_POINT ( 'NONE',  ( -4.278324951949325161, 39.54020021135848140, 53.33400390260339918 ) ) ;
#13121=EDGE_LOOP ( 'NONE', ( #18006, #4525, #16422, #1851 ) ) ;
#13123=VERTEX_POINT ( 'NONE', #5573 ) ;
#13124=CARTESIAN_POINT ( 'NONE',  ( -18.03138881840362373, 11.33611194795425448, 60.11697748794932039 ) ) ;
#13125=DIRECTION ( 'NONE',  ( 0.000000000000000000, 0.000000000000000000, 1.000000000000000000 ) ) ;
#13126=STYLED_ITEM('',(#22727),#17721);
#13127=CIRCLE ( 'NONE', #6561, 2.499999999999998668 ) ;
#13130=EDGE_CURVE ( 'NONE', #16148, #18333, #8306, .T. ) ;
#13133=CARTESIAN_POINT ( 'NONE',  ( -5.702716825708717074, 39.17357718829572377, -54.58701425223105019 ) ) ;
#13135=ORIENTED_EDGE ( 'NONE', *, *, #5495, .F. ) ;
#13136=EDGE_CURVE ( 'NONE', #13854, #16362, #3867, .T. ) ;
#13137=DIRECTION ( 'NONE',  ( 0.000000000000000000, 0.000000000000000000, -1.000000000000000000 ) ) ;
#13138=CARTESIAN_POINT ( 'NONE',  ( -35.00000000000058265, 28.00000000000000000, -57.50000000000076028 ) ) ;
#13139=CARTESIAN_POINT ( 'NONE',  ( 17.58064943503729083, 10.42262370234225166, 57.45835854660180786 ) ) ;
#13141=ORIENTED_EDGE ( 'NONE', *, *, #4723, .T. ) ;
#13144=CIRCLE ( 'NONE', #20122, 2.499999999999996891 ) ;
#13145=FACE_OUTER_BOUND ( 'NONE', #5600, .T. ) ;
#13147=CARTESIAN_POINT ( 'NONE',  ( -34.99999999999980815, 28.00000000000000000, 52.89999999999922409 ) ) ;
#13150=CARTESIAN_POINT ( 'NONE',  ( 6.816855646551482018, 40.00000000000000711, -52.46799118524486971 ) ) ;
#13151=VERTEX_POINT ( 'NONE', #10836 ) ;
#13152=CARTESIAN_POINT ( 'NONE',  ( 1.095802490588493994, 39.99285411162865955, -49.56761786991830121 ) ) ;
#13156=DIRECTION ( 'NONE',  ( -0.5002637533272162873, 0.000000000000000000, -0.8658730721687598608 ) ) ;
#13157=CARTESIAN_POINT ( 'NONE',  ( -90.00000000000000000, 39.97500000000000142, -9.108981535246192915E-16 ) ) ;
#13159=CARTESIAN_POINT ( 'NONE',  ( -8.774779751595641386, 39.47272031439209883, 54.19450202971452768 ) ) ;
#13160=CARTESIAN_POINT ( 'NONE',  ( 35.00000000000000000, 40.00000000000000000, -49.99999999999997868 ) ) ;
#13162=DIRECTION ( 'NONE',  ( 0.000000000000000000, 0.000000000000000000, -1.000000000000000000 ) ) ;
#13163=CARTESIAN_POINT ( 'NONE',  ( 90.00000000000000000, 40.00000000000000711, -2.525000000000000355 ) ) ;
#13164=CARTESIAN_POINT ( 'NONE',  ( -0.02784959653163695745, 39.99999544702608745, -48.75564068409102703 ) ) ;
#13165=EDGE_LOOP ( 'NONE', ( #3033, #12622, #5622, #5155 ) ) ;
#13166=CARTESIAN_POINT ( 'NONE',  ( -15.00000000000001421, 20.00000000000000355, 45.82575694955841072 ) ) ;
#13168=EDGE_CURVE ( 'NONE', #22583, #13103, #7185, .T. ) ;
#13169=ORIENTED_EDGE ( 'NONE', *, *, #16776, .T. ) ;
#13170=ADVANCED_FACE ( 'NONE', ( #21171 ), #532, .T. ) ;
#13174=CARTESIAN_POINT ( 'NONE',  ( 19.64447802513831220, 23.87744830687368136, 60.53680291695862792 ) ) ;
#13175=DIRECTION ( 'NONE',  ( -0.000000000000000000, 1.000000000000000000, -0.000000000000000000 ) ) ;
#13178=LINE ( 'NONE', #13066, #18237 ) ;
#13180=DIRECTION ( 'NONE',  ( 0.000000000000000000, 0.000000000000000000, 1.000000000000000000 ) ) ;
#13184=CARTESIAN_POINT ( 'NONE',  ( 7.088850870549147224E-15, -5.000000000000000000, 44.98888751680801334 ) ) ;
#13185=CARTESIAN_POINT ( 'NONE',  ( 14.58570206007858694, 6.310259562106195652, -59.03202081059063033 ) ) ;
#13186=ORIENTED_EDGE ( 'NONE', *, *, #3170, .T. ) ;
#13189=CARTESIAN_POINT ( 'NONE',  ( 7.538461658765248430, 38.52939893239186375, -55.92178727523597814 ) ) ;
#13191=CARTESIAN_POINT ( 'NONE',  ( 6.297058390208000844, 38.99690150456885362, 53.73986305459201418 ) ) ;
#13192=ORIENTED_EDGE ( 'NONE', *, *, #14888, .F. ) ;
#13193=CARTESIAN_POINT ( 'NONE',  ( 13.88612301964874796, 34.41939562427457844, 58.78253654025287034 ) ) ;
#13194=CARTESIAN_POINT ( 'NONE',  ( -18.00000000000001421, 20.00000000000000711, 105.0000000000000142 ) ) ;
#13197=CARTESIAN_POINT ( 'NONE',  ( 16.72418712224170534, 8.992692292686992772, -57.18730031742025943 ) ) ;
#13198=ORIENTED_EDGE ( 'NONE', *, *, #22362, .F. ) ;
#13200=ORIENTED_EDGE ( 'NONE', *, *, #16777, .T. ) ;
#13201=ORIENTED_EDGE ( 'NONE', *, *, #2148, .F. ) ;
#13203=CARTESIAN_POINT ( 'NONE',  ( -35.00000000000000000, 39.00000000000000711, 1.387778780781445676E-14 ) ) ;
#13205=CIRCLE ( 'NONE', #2979, 2.525000000000110489 ) ;
#13211=CARTESIAN_POINT ( 'NONE',  ( 34.99999999999980815, 28.00000000000000000, 52.89999999999922409 ) ) ;
#13217=CARTESIAN_POINT ( 'NONE',  ( -19.43416121892457582, 24.82270088923175777, -60.48577746614100192 ) ) ;
#13219=EDGE_CURVE ( 'NONE', #5859, #12070, #13762, .T. ) ;
#13221=AXIS2_PLACEMENT_3D ( 'NONE', #6301, #22236, #16614 ) ;
#13227=CARTESIAN_POINT ( 'NONE',  ( -17.19628968518555823, 9.778502620742683504, 59.87797704339187277 ) ) ;
#13228=FACE_OUTER_BOUND ( 'NONE', #17220, .T. ) ;
#13230=DIRECTION ( 'NONE',  ( 0.000000000000000000, 0.000000000000000000, -1.000000000000000000 ) ) ;
#13235=CARTESIAN_POINT ( 'NONE',  ( -7.073806678778195689, 38.72385539215704142, -54.13592748070715288 ) ) ;
#13242=CARTESIAN_POINT ( 'NONE',  ( -5.816608766684079335, -4.770324936805427463, -49.23968220743358160 ) ) ;
#13249=CARTESIAN_POINT ( 'NONE',  ( 0.6792558703086061245, -1.217297189599438445, 47.76386722475271540 ) ) ;
#13253=CARTESIAN_POINT ( 'NONE',  ( 5.178711896350565169, 39.83381987255487644, -52.32443819789842365 ) ) ;
#13256=CARTESIAN_POINT ( 'NONE',  ( -90.00000000000000000, 40.00000000000000000, -9.108981535246192915E-16 ) ) ;
#13258=CARTESIAN_POINT ( 'NONE',  ( 42.50000000000000711, -5.000000000000000000, -45.40000000000000568 ) ) ;
#13259=VECTOR ( 'NONE', #3517, 1000.000000000000000 ) ;
#13267=VECTOR ( 'NONE', #1527, 1000.000000000000000 ) ;
#13271=ORIENTED_EDGE ( 'NONE', *, *, #6708, .F. ) ;
#13272=CIRCLE ( 'NONE', #17321, 30.00000000000000000 ) ;
#13273=VERTEX_POINT ( 'NONE', #2372 ) ;
#13276=ORIENTED_EDGE ( 'NONE', *, *, #5673, .T. ) ;
#13277=CARTESIAN_POINT ( 'NONE',  ( 15.58771758597473500, 32.56665981830160206, -59.37826087086040872 ) ) ;
#13278=CARTESIAN_POINT ( 'NONE',  ( 42.50000000000000711, -12.00000000000012434, -47.50000000000000000 ) ) ;
#13281=DIRECTION ( 'NONE',  ( -0.000000000000000000, -1.000000000000000000, -0.000000000000000000 ) ) ;
#13283=DIRECTION ( 'NONE',  ( 0.000000000000000000, -1.000000000000000000, 0.000000000000000000 ) ) ;
#13285=ORIENTED_EDGE ( 'NONE', *, *, #18029, .F. ) ;
#13286=CARTESIAN_POINT ( 'NONE',  ( -5.249999999999990230, 40.00000000000000000, -41.42387596543809991 ) ) ;
#13291=FACE_OUTER_BOUND ( 'NONE', #5575, .T. ) ;
#13294=CARTESIAN_POINT ( 'NONE',  ( 2.546709079545405707, 39.84786395731773467, -51.61893211308333917 ) ) ;
#13300=LINE ( 'NONE', #4635, #3225 ) ;
#13303=AXIS2_PLACEMENT_3D ( 'NONE', #21063, #6976, #1583 ) ;
#13304=CARTESIAN_POINT ( 'NONE',  ( 15.39832585462649028, 32.77960222724997408, 56.73873823673486783 ) ) ;
#13305=CARTESIAN_POINT ( 'NONE',  ( -1.387778780781445518E-14, 20.00000000000000355, -102.0000000000000142 ) ) ;
#13307=CARTESIAN_POINT ( 'NONE',  ( 15.06903587914752229, 33.17837898604023650, -59.20328215072071742 ) ) ;
#13309=ORIENTED_EDGE ( 'NONE', *, *, #4115, .F. ) ;
#13312=ORIENTED_EDGE ( 'NONE', *, *, #680, .T. ) ;
#13313=ORIENTED_EDGE ( 'NONE', *, *, #11800, .F. ) ;
#13326=CARTESIAN_POINT ( 'NONE',  ( -42.50000000000000711, -12.00000000000000000, -50.00000000000000000 ) ) ;
#13327=CARTESIAN_POINT ( 'NONE',  ( -3.949642717238829380E-15, -1.890954608135210879, -47.89513957784965470 ) ) ;
#13328=CARTESIAN_POINT ( 'NONE',  ( -19.85669122310597601, 22.43861522864551006, -60.58781117059879762 ) ) ;
#13335=EDGE_CURVE ( 'NONE', #9888, #16403, #12667, .T. ) ;
#13338=CARTESIAN_POINT ( 'NONE',  ( -18.69481036107322325, 7.531781294122753323, 57.74428367179859833 ) ) ;
#13340=CIRCLE ( 'NONE', #6774, 2.499999999999998668 ) ;
#13342=FACE_OUTER_BOUND ( 'NONE', #17898, .T. ) ;
#13344=VECTOR ( 'NONE', #6224, 1000.000000000000114 ) ;
#13348=CARTESIAN_POINT ( 'NONE',  ( -35.00000000000058265, 40.00000000000000000, -57.10000000000076170 ) ) ;
#13349=DIRECTION ( 'NONE',  ( 0.000000000000000000, 0.000000000000000000, -1.000000000000000000 ) ) ;
#13351=DIRECTION ( 'NONE',  ( 0.000000000000000000, 0.000000000000000000, 1.000000000000000000 ) ) ;
#13353=ADVANCED_FACE ( 'NONE', ( #7750 ), #14719, .F. ) ;
#13361=DIRECTION ( 'NONE',  ( 0.000000000000000000, -1.000000000000000000, 0.000000000000000000 ) ) ;
#13366=EDGE_LOOP ( 'NONE', ( #13917, #2911, #12853, #17073 ) ) ;
#13371=CARTESIAN_POINT ( 'NONE',  ( -42.50000000000000711, -3.738192700042122674, 47.50000000000000711 ) ) ;
#13373=ORIENTED_EDGE ( 'NONE', *, *, #8006, .F. ) ;
#13374=AXIS2_PLACEMENT_3D ( 'NONE', #5328, #1887, #14118 ) ;
#13377=DIRECTION ( 'NONE',  ( -0.000000000000000000, 1.000000000000000000, -0.000000000000000000 ) ) ;
#13378=CARTESIAN_POINT ( 'NONE',  ( -15.03694978696328732, 3.237610724667264961, -56.60357944353420123 ) ) ;
#13379=EDGE_CURVE ( 'NONE', #454, #18218, #21588, .T. ) ;
#13380=CARTESIAN_POINT ( 'NONE',  ( -13.07600923154788575, 27.35939529837144235, -44.93756990742565449 ) ) ;
#13381=AXIS2_PLACEMENT_3D ( 'NONE', #6971, #15196, #17154 ) ;
#13383=VERTEX_POINT ( 'NONE', #11031 ) ;
#13384=DIRECTION ( 'NONE',  ( 0.000000000000000000, -1.000000000000000000, 0.000000000000000000 ) ) ;
#13386=CARTESIAN_POINT ( 'NONE',  ( 9.062586715439639562, 2.130694986424134907, -54.31128890271873644 ) ) ;
#13388=EDGE_LOOP ( 'NONE', ( #20575, #20232, #13276 ) ) ;
#13394=AXIS2_PLACEMENT_3D ( 'NONE', #12336, #7525, #5689 ) ;
#13398=CARTESIAN_POINT ( 'NONE',  ( 19.29031483250422596, 25.30268833713984122, -60.44930483060156945 ) ) ;
#13402=CARTESIAN_POINT ( 'NONE',  ( 2.855944605007590287, 5.272200938804487258, -39.14690304189951320 ) ) ;
#13406=ORIENTED_EDGE ( 'NONE', *, *, #10554, .T. ) ;
#13409=CARTESIAN_POINT ( 'NONE',  ( 2.995584608082006106, -1.237002266245721627, -50.27666343020538164 ) ) ;
#13411=CARTESIAN_POINT ( 'NONE',  ( 19.99999999999998579, 19.20373330966867442, -60.62177826491069510 ) ) ;
#13412=EDGE_LOOP ( 'NONE', ( #8802, #4035, #12950, #6009, #5964, #20173, #15137 ) ) ;
#13413=CARTESIAN_POINT ( 'NONE',  ( -3.995109296550547473, 40.00000000000000711, -51.09401224245644357 ) ) ;
#13420=DIRECTION ( 'NONE',  ( -0.000000000000000000, -0.000000000000000000, -1.000000000000000000 ) ) ;
#13423=CARTESIAN_POINT ( 'NONE',  ( 19.88905041091779324, 17.72428093567802776, -58.11830361001567979 ) ) ;
#13425=AXIS2_PLACEMENT_3D ( 'NONE', #3333, #8700, #19130 ) ;
#13427=VERTEX_POINT ( 'NONE', #8972 ) ;
#13437=CARTESIAN_POINT ( 'NONE',  ( -5.079212789376158277, -3.097595057465493795, -50.74825967503716839 ) ) ;
#13442=CARTESIAN_POINT ( 'NONE',  ( 5.702716825709497783, 39.17357718829546798, -54.58701425223458870 ) ) ;
#13443=CIRCLE ( 'NONE', #4690, 18.00000000000000000 ) ;
#13445=CARTESIAN_POINT ( 'NONE',  ( 12.99999999999993960, 42.51666049839543149, 105.0000000000000142 ) ) ;
#13447=CARTESIAN_POINT ( 'NONE',  ( -9.940687323067972869, 37.37897894777885455, -57.14641600008366851 ) ) ;
#13448=CARTESIAN_POINT ( 'NONE',  ( -14.52224280010138280, 16.16745304956414486, 45.61498238574518638 ) ) ;
#13453=CIRCLE ( 'NONE', #6527, 2.499999999999995115 ) ;
#13456=CARTESIAN_POINT ( 'NONE',  ( -14.69246073108895168, 6.394048232430655787, 56.48929660089485338 ) ) ;
#13457=EDGE_CURVE ( 'NONE', #17863, #15580, #5534, .T. ) ;
#13459=DIRECTION ( 'NONE',  ( 0.000000000000000000, 0.000000000000000000, 1.000000000000000000 ) ) ;
#13460=DIRECTION ( 'NONE',  ( 1.000000000000000000, 0.000000000000000000, 0.000000000000000000 ) ) ;
#13465=CARTESIAN_POINT ( 'NONE',  ( -5.345263555475219697, 39.99999999999999289, -51.78208643630931363 ) ) ;
#13466=AXIS2_PLACEMENT_3D ( 'NONE', #12154, #3463, #5290 ) ;
#13472=CARTESIAN_POINT ( 'NONE',  ( -10.78076590482871211, 39.17366535989417287, 54.93576791444288432 ) ) ;
#13482=CIRCLE ( 'NONE', #8387, 2.500000000000002220 ) ;
#13484=LINE ( 'NONE', #22111, #1609 ) ;
#13487=DIRECTION ( 'NONE',  ( 0.5002637533272700221, 0.000000000000000000, -0.8658730721687286636 ) ) ;
#13488=CARTESIAN_POINT ( 'NONE',  ( 35.00000000000058265, 28.00000000000000000, -57.10000000000076170 ) ) ;
#13489=CARTESIAN_POINT ( 'NONE',  ( -2.425350241063221279, 40.00000000000000000, 50.22136039941155161 ) ) ;
#13490=CARTESIAN_POINT ( 'NONE',  ( -21.22368364729210910, 12.66551901741667585, -58.39771426751148198 ) ) ;
#13491=CARTESIAN_POINT ( 'NONE',  ( -7.259789697909740269, 39.65417261969281526, 53.48039063277445848 ) ) ;
#13492=CARTESIAN_POINT ( 'NONE',  ( -17.17026400045400436, 34.49621688465821023, 57.29349885535140174 ) ) ;
#13493=ADVANCED_FACE ( 'NONE', ( #17573 ), #17914, .F. ) ;
#13499=DIRECTION ( 'NONE',  ( 0.000000000000000000, 0.000000000000000000, 1.000000000000000000 ) ) ;
#13501=CARTESIAN_POINT ( 'NONE',  ( -13.56354382738803466, 2.142135623730931471, 56.03997097393687454 ) ) ;
#13502=DIRECTION ( 'NONE',  ( 0.000000000000000000, 0.000000000000000000, 1.000000000000000000 ) ) ;
#13506=EDGE_CURVE ( 'NONE', #13935, #21335, #9201, .T. ) ;
#13509=VECTOR ( 'NONE', #20014, 1000.000000000000000 ) ;
#13510=EDGE_CURVE ( 'NONE', #17179, #11978, #488, .T. ) ;
#13511=ORIENTED_EDGE ( 'NONE', *, *, #18574, .F. ) ;
#13512=PRODUCT_CONTEXT ( 'NONE', #14261, 'mechanical' ) ;
#13513=ORIENTED_EDGE ( 'NONE', *, *, #590, .F. ) ;
#13517=CARTESIAN_POINT ( 'NONE',  ( 21.99999999999998579, 20.00000000000000355, -100.0000000000000000 ) ) ;
#13518=DIRECTION ( 'NONE',  ( -1.000000000000000000, 0.000000000000000000, 0.000000000000000000 ) ) ;
#13521=DIRECTION ( 'NONE',  ( 0.000000000000000000, -1.000000000000000000, 0.000000000000000000 ) ) ;
#13523=DIRECTION ( 'NONE',  ( 1.000000000000000000, 0.000000000000000000, 0.000000000000000000 ) ) ;
#13527=CARTESIAN_POINT ( 'NONE',  ( 9.455104429560558188, 39.37252125300741312, 54.46735621542109840 ) ) ;
#13532=CARTESIAN_POINT ( 'NONE',  ( -14.68518659845081409, 36.96998281527654484, 56.45735093204006461 ) ) ;
#13533=ORIENTED_EDGE ( 'NONE', *, *, #18889, .T. ) ;
#13537=CARTESIAN_POINT ( 'NONE',  ( 18.85220035178958042, 32.22744690108880405, -57.78902400853694843 ) ) ;
#13538=ORIENTED_EDGE ( 'NONE', *, *, #12170, .T. ) ;
#13541=ADVANCED_FACE ( 'NONE', ( #21932 ), #11143, .T. ) ;
#13547=DIRECTION ( 'NONE',  ( -0.000000000000000000, -0.000000000000000000, 1.000000000000000000 ) ) ;
#13551=CARTESIAN_POINT ( 'NONE',  ( -9.079900084793857573, 0.2952492082908969584, -53.92155889450898343 ) ) ;
#13552=ORIENTED_EDGE ( 'NONE', *, *, #5485, .F. ) ;
#13555=FACE_OUTER_BOUND ( 'NONE', #12817, .T. ) ;
#13559=CARTESIAN_POINT ( 'NONE',  ( -0.3011557478976217284, 39.99946772338066836, 48.96697170734454829 ) ) ;
#13561=EDGE_CURVE ( 'NONE', #20205, #3398, #12679, .T. ) ;
#13564=CONICAL_SURFACE ( 'NONE', #19453, 2.099999999999997868, 1.029744258676653867 ) ;
#13567=ORIENTED_EDGE ( 'NONE', *, *, #14974, .T. ) ;
#13568=CARTESIAN_POINT ( 'NONE',  ( -17.29817675749697514, 30.08054145047330508, 57.37022932959109056 ) ) ;
#13571=CARTESIAN_POINT ( 'NONE',  ( -11.59091061707577275, 39.99999999999998579, 54.17810196248734655 ) ) ;
#13574=CARTESIAN_POINT ( 'NONE',  ( -8.616492346064047680, 40.00000000000000000, -53.19943576996322321 ) ) ;
#13576=EDGE_CURVE ( 'NONE', #1383, #16162, #1171, .T. ) ;
#13577=ORIENTED_EDGE ( 'NONE', *, *, #13947, .T. ) ;
#13579=EDGE_CURVE ( 'NONE', #6038, #3138, #6657, .T. ) ;
#13585=ORIENTED_EDGE ( 'NONE', *, *, #11777, .F. ) ;
#13587=CARTESIAN_POINT ( 'NONE',  ( -0.2357944722115355995, -1.232758281750954144, 48.43260639659581557 ) ) ;
#13589=EDGE_CURVE ( 'NONE', #17185, #4605, #20021, .T. ) ;
#13591=ORIENTED_EDGE ( 'NONE', *, *, #21032, .F. ) ;
#13592=CARTESIAN_POINT ( 'NONE',  ( 19.99999999999998579, 20.00000000000000000, 98.00000000000000000 ) ) ;
#13595=CARTESIAN_POINT ( 'NONE',  ( 90.00000000000000000, 28.00000000000000000, -9.108981535246192915E-16 ) ) ;
#13597=CARTESIAN_POINT ( 'NONE',  ( -22.38794582965170221, 21.29119307984318255, -58.65949541090341057 ) ) ;
#13598=CARTESIAN_POINT ( 'NONE',  ( -7.899720326450768049, 39.58366711203084520, 53.79762300408461329 ) ) ;
#13599=CARTESIAN_POINT ( 'NONE',  ( -15.21899206303018026, 36.51951236530621969, 56.65045400726779690 ) ) ;
#13602=FACE_BOUND ( 'NONE', #19074, .T. ) ;
#13603=DIRECTION ( 'NONE',  ( -0.000000000000000000, -0.000000000000000000, -1.000000000000000000 ) ) ;
#13604=CARTESIAN_POINT ( 'NONE',  ( -26.00000000000001421, 19.99999999999982947, 60.00099999999999767 ) ) ;
#13611=ORIENTED_EDGE ( 'NONE', *, *, #12656, .T. ) ;
#13612=EDGE_CURVE ( 'NONE', #105, #15831, #13781, .T. ) ;
#13616=DIRECTION ( 'NONE',  ( 3.585095183685401065E-15, 0.000000000000000000, 1.000000000000000000 ) ) ;
#13618=CARTESIAN_POINT ( 'NONE',  ( 19.99999999999998934, 18.38876824873586102, 60.62177826491085852 ) ) ;
#13622=CARTESIAN_POINT ( 'NONE',  ( -10.15869103000896345, 39.99999999999999289, -53.70409622859170895 ) ) ;
#13623=ORIENTED_EDGE ( 'NONE', *, *, #4648, .T. ) ;
#13624=EDGE_CURVE ( 'NONE', #5986, #4461, #17043, .T. ) ;
#13626=AXIS2_PLACEMENT_3D ( 'NONE', #15713, #30, #17554 ) ;
#13628=CARTESIAN_POINT ( 'NONE',  ( -13.56354382738803999, 2.142135623730931471, -56.03997097393684612 ) ) ;
#13630=ORIENTED_EDGE ( 'NONE', *, *, #2047, .F. ) ;
#13633=CARTESIAN_POINT ( 'NONE',  ( 10.49999999999994316, 42.51666049839543149, 60.00099999999999767 ) ) ;
#13635=CARTESIAN_POINT ( 'NONE',  ( -21.93942599038056684, 24.73590942562832140, 58.56147853046847018 ) ) ;
#13637=CARTESIAN_POINT ( 'NONE',  ( -90.00000000000000000, 28.00000000000000000, 2.500000000000001332 ) ) ;
#13638=( BOUNDED_SURFACE ( )  B_SPLINE_SURFACE ( 3, 2, ( 
 ( #8905, #15879, #17269 ),
 ( #193, #17727, #7308 ),
 ( #17615, #1922, #14158 ),
 ( #15544, #21176, #7074 ),
 ( #5476, #6863, #12447 ),
 ( #22570, #10723, #9021 ),
 ( #19119, #5256, #10387 ),
 ( #1705, #12231, #19235 ),
 ( #19460, #21286, #3545 ),
 ( #10502, #21861, #17844 ) ),
 .UNSPECIFIED., .F., .F., .F. ) 
 B_SPLINE_SURFACE_WITH_KNOTS ( ( 4, 2, 2, 2, 4 ),
 ( 3, 3 ),
 ( 0.02809317535148400657, 0.03071213539476974272, 0.03333109543805547886, 0.03595005548134121154, 0.03856901552462695115 ),
 ( 0.000000000000000000, 0.7610267056326938118 ),
 .UNSPECIFIED. ) 
 GEOMETRIC_REPRESENTATION_ITEM ( )  RATIONAL_B_SPLINE_SURFACE ( (
 ( 1.000000000000000000, 0.9420702913958448610, 0.9723126933862540344),
 ( 1.000000000000000000, 0.9476767737754007159, 0.9749922925143632568),
 ( 1.000000000000000000, 0.9527464803503639112, 0.9774153414777524418),
 ( 1.000000000000000000, 0.9613642323582910487, 0.9815341666525020381),
 ( 1.000000000000000000, 0.9649023417790275614, 0.9832251939807128416),
 ( 1.000000000000000000, 0.9700537923985854682, 0.9856873122313654090),
 ( 1.000000000000000000, 0.9716607116685208601, 0.9864553338148029926),
 ( 1.000000000000000000, 0.9729170072999735464, 0.9870557760262979041),
 ( 1.000000000000000000, 0.9725773074833657938, 0.9868934176577563999),
 ( 1.000000000000000000, 0.9714158944602965251, 0.9863383242652685734) ) ) 
 REPRESENTATION_ITEM ( '' )  SURFACE ( )  );
#13640=ADVANCED_FACE ( 'NONE', ( #13291 ), #12208, .T. ) ;
#13641=DIRECTION ( 'NONE',  ( 0.000000000000000000, 0.000000000000000000, -1.000000000000000000 ) ) ;
#13653=CARTESIAN_POINT ( 'NONE',  ( 18.32709649528715090, 33.00101640267666880, 57.63983358650816768 ) ) ;
#13655=CARTESIAN_POINT ( 'NONE',  ( 9.952189117650862116, 40.00000000000000000, -53.64426396172072486 ) ) ;
#13660=FACE_OUTER_BOUND ( 'NONE', #12618, .T. ) ;
#13663=CARTESIAN_POINT ( 'NONE',  ( 5.833333333333329485, 39.00000000000000711, -40.61164310337066041 ) ) ;
#13664=CIRCLE ( 'NONE', #1925, 2.500000000000002220 ) ;
#13666=DIRECTION ( 'NONE',  ( -1.000000000000000000, 0.000000000000000000, 0.000000000000000000 ) ) ;
#13667=CARTESIAN_POINT ( 'NONE',  ( -2.247171121184980525, 39.96957905804138278, 50.40104600615941166 ) ) ;
#13672=CARTESIAN_POINT ( 'NONE',  ( -42.50000000000000711, -9.600000000000001421, 47.50000000000000711 ) ) ;
#13673=EDGE_CURVE ( 'NONE', #19784, #21644, #3357, .T. ) ;
#13680=EDGE_LOOP ( 'NONE', ( #906, #4279 ) ) ;
#13681=CARTESIAN_POINT ( 'NONE',  ( -12.91716037299260122, 4.693711897366395824, 55.81219010901885724 ) ) ;
#13682=CARTESIAN_POINT ( 'NONE',  ( -11.99035502499710937, 39.33333333333332860, 55.05149724789903587 ) ) ;
#13683=CARTESIAN_POINT ( 'NONE',  ( -35.00000000000000000, 40.00000000000000000, -58.99999999999992895 ) ) ;
#13685=CARTESIAN_POINT ( 'NONE',  ( -12.01755860117731523, 39.99999999999999289, 54.34185968360770147 ) ) ;
#13687=CARTESIAN_POINT ( 'NONE',  ( -42.50000000000000711, -9.600000000000001421, 45.00000000000000711 ) ) ;
#13688=CARTESIAN_POINT ( 'NONE',  ( 34.99999999999980815, 40.00000000000000000, 57.49999999999921840 ) ) ;
#13690=FACE_BOUND ( 'NONE', #15123, .T. ) ;
#13702=ORIENTED_EDGE ( 'NONE', *, *, #5495, .T. ) ;
#13703=VECTOR ( 'NONE', #14629, 1000.000000000000000 ) ;
#13706=ORIENTED_EDGE ( 'NONE', *, *, #22049, .F. ) ;
#13707=CIRCLE ( 'NONE', #8608, 2.500000000000002220 ) ;
#13708=CARTESIAN_POINT ( 'NONE',  ( -2.438270697430720446, -3.148887331866972783, 49.03407609142411872 ) ) ;
#13716=CARTESIAN_POINT ( 'NONE',  ( -16.23901130407228166, 8.288052467681200852, -57.02826995000967258 ) ) ;
#13717=DIRECTION ( 'NONE',  ( 0.000000000000000000, 0.000000000000000000, -1.000000000000000000 ) ) ;
#13718=CIRCLE ( 'NONE', #14090, 2.499999999999996891 ) ;
#13720=CARTESIAN_POINT ( 'NONE',  ( 8.188149873056865147, 32.58630821608365835, 42.20917188641859497 ) ) ;
#13723=CARTESIAN_POINT ( 'NONE',  ( 42.50000000000000711, -5.000000000000000000, -47.50000000000000000 ) ) ;
#13724=CIRCLE ( 'NONE', #19607, 58.99999999999994316 ) ;
#13728=AXIS2_PLACEMENT_3D ( 'NONE', #18356, #7944, #2676 ) ;
#13731=AXIS2_PLACEMENT_3D ( 'NONE', #18853, #20570, #3387 ) ;
#13734=DIRECTION ( 'NONE',  ( -0.000000000000000000, -1.000000000000000000, -0.000000000000000000 ) ) ;
#13738=DIRECTION ( 'NONE',  ( 0.000000000000000000, 0.000000000000000000, -1.000000000000000000 ) ) ;
#13741=EDGE_LOOP ( 'NONE', ( #20474, #18366, #21710, #11436 ) ) ;
#13742=DIRECTION ( 'NONE',  ( -0.000000000000000000, -0.000000000000000000, 1.000000000000000000 ) ) ;
#13743=FACE_OUTER_BOUND ( 'NONE', #11198, .T. ) ;
#13745=CARTESIAN_POINT ( 'NONE',  ( -42.50000000000000711, -11.97499999999999964, 45.00000000000000711 ) ) ;
#13747=CARTESIAN_POINT ( 'NONE',  ( -35.00000000000000000, 40.00000000000000000, 1.387778780781445676E-14 ) ) ;
#13749=DIRECTION ( 'NONE',  ( -1.000000000000000000, 0.000000000000000000, 0.000000000000000000 ) ) ;
#13751=DIRECTION ( 'NONE',  ( -0.000000000000000000, -1.000000000000000000, -0.000000000000000000 ) ) ;
#13753=CIRCLE ( 'NONE', #2808, 2.499999999999998668 ) ;
#13755=CIRCLE ( 'NONE', #16322, 2.499999999999995115 ) ;
#13756=VECTOR ( 'NONE', #19134, 1000.000000000000000 ) ;
#13762=CIRCLE ( 'NONE', #617, 2.525000000000110489 ) ;
#13763=CARTESIAN_POINT ( 'NONE',  ( -1.387778780781445518E-14, 20.00000000000000355, -105.0000000000000142 ) ) ;
#13764=EDGE_CURVE ( 'NONE', #19146, #121, #9252, .T. ) ;
#13767=EDGE_LOOP ( 'NONE', ( #8715, #15359, #2552, #4552 ) ) ;
#13768=EDGE_LOOP ( 'NONE', ( #17092, #7145, #20769, #7101 ) ) ;
#13770=AXIS2_PLACEMENT_3D ( 'NONE', #7457, #21560, #4479 ) ;
#13771=ORIENTED_EDGE ( 'NONE', *, *, #12786, .F. ) ;
#13773=CARTESIAN_POINT ( 'NONE',  ( -13.00000000000011546, 42.51666049839536043, -105.0000000000000142 ) ) ;
#13776=ORIENTED_EDGE ( 'NONE', *, *, #9112, .F. ) ;
#13777=PLANE ( 'NONE',  #18606 ) ;
#13778=CARTESIAN_POINT ( 'NONE',  ( -0.2227364088731864089, -1.232651810764356037, -48.42315971483976966 ) ) ;
#13780=CARTESIAN_POINT ( 'NONE',  ( -3.313694450323563689, 0.2469464189807611398, 51.08096178187792447 ) ) ;
#13781=CIRCLE ( 'NONE', #10122, 51.00000000000002132 ) ;
#13782=CARTESIAN_POINT ( 'NONE',  ( 2.095812652544434496, 34.85510830401392468, 38.95253985045414424 ) ) ;
#13784=CARTESIAN_POINT ( 'NONE',  ( 8.123113521816467397, 39.63127166633003640, -53.85467626787994533 ) ) ;
#13788=CARTESIAN_POINT ( 'NONE',  ( -0.4976657361290892090, 39.99853738388662805, 49.11742177756252659 ) ) ;
#13800=CARTESIAN_POINT ( 'NONE',  ( 90.00000000000000000, 26.00000000000000355, -9.108981535246192915E-16 ) ) ;
#13802=AXIS2_PLACEMENT_3D ( 'NONE', #2562, #17792, #19632 ) ;
#13804=ADVANCED_FACE ( 'NONE', ( #19914 ), #7659, .F. ) ;
#13806=CARTESIAN_POINT ( 'NONE',  ( 4.273192510725268178, 39.88698591164679641, 51.75894906208631596 ) ) ;
#13810=LINE ( 'NONE', #13348, #12661 ) ;
#13812=DIRECTION ( 'NONE',  ( -0.000000000000000000, 1.000000000000000000, -0.000000000000000000 ) ) ;
#13814=ORIENTED_EDGE ( 'NONE', *, *, #14399, .T. ) ;
#13817=CARTESIAN_POINT ( 'NONE',  ( -20.00000000000001421, 20.97067337953453858, 60.62177826491070221 ) ) ;
#13826=ORIENTED_EDGE ( 'NONE', *, *, #7776, .F. ) ;
#13832=ORIENTED_EDGE ( 'NONE', *, *, #5039, .F. ) ;
#13834=CARTESIAN_POINT ( 'NONE',  ( 12.68897045256288258, 11.99170770793158525, 44.74667050109238176 ) ) ;
#13835=ADVANCED_FACE ( 'NONE', ( #17852 ), #21857, .F. ) ;
#13836=CARTESIAN_POINT ( 'NONE',  ( -4.985660570713215556, 34.15523982581864715, -40.05045397208977676 ) ) ;
#13837=DIRECTION ( 'NONE',  ( -1.000000000000000000, 0.000000000000000000, 0.000000000000000000 ) ) ;
#13838=CARTESIAN_POINT ( 'NONE',  ( -21.98712579307494508, 15.48449832073882781, -58.57208548029186801 ) ) ;
#13840=CARTESIAN_POINT ( 'NONE',  ( -14.76055860720891033, 22.69766935715934508, -45.72055682016588918 ) ) ;
#13842=DIRECTION ( 'NONE',  ( 0.000000000000000000, 0.000000000000000000, -1.000000000000000000 ) ) ;
#13843=DIRECTION ( 'NONE',  ( -0.000000000000000000, 1.000000000000000000, -0.000000000000000000 ) ) ;
#13849=CIRCLE ( 'NONE', #20090, 9.000000000000003553 ) ;
#13851=DIRECTION ( 'NONE',  ( 1.000000000000000000, 0.000000000000000000, 0.000000000000000000 ) ) ;
#13854=VERTEX_POINT ( 'NONE', #10973 ) ;
#13858=CARTESIAN_POINT ( 'NONE',  ( -42.50000000000000711, -5.000000000000000000, -54.00000000000000000 ) ) ;
#13861=ORIENTED_EDGE ( 'NONE', *, *, #5392, .F. ) ;
#13862=DIRECTION ( 'NONE',  ( 0.000000000000000000, -1.000000000000000000, 0.000000000000000000 ) ) ;
#13865=CARTESIAN_POINT ( 'NONE',  ( 7.776554266669417956E-15, -4.648749848372173865, -45.43309249825056639 ) ) ;
#13866=CARTESIAN_POINT ( 'NONE',  ( 21.73016838732307576, 25.62687619368169223, -58.51481333197131818 ) ) ;
#13868=CARTESIAN_POINT ( 'NONE',  ( -7.474679935337165126, 39.63145871004727638, -53.58934899115953243 ) ) ;
#13870=DIRECTION ( 'NONE',  ( 0.000000000000000000, 0.000000000000000000, 1.000000000000000000 ) ) ;
#13871=CARTESIAN_POINT ( 'NONE',  ( 6.696867368503558448E-15, 40.00000000000000000, 48.73397172404481381 ) ) ;
#13878=CARTESIAN_POINT ( 'NONE',  ( 35.00000000000058265, 26.00000000000000355, -57.10000000000076170 ) ) ;
#13886=CARTESIAN_POINT ( 'NONE',  ( 18.74703631669234127, 7.639653230112233295, 57.75728470191489805 ) ) ;
#13889=CARTESIAN_POINT ( 'NONE',  ( 4.643077362641815142, 40.00000000000000711, 51.42938339147494275 ) ) ;
#13890=EDGE_CURVE ( 'NONE', #21191, #12680, #17405, .T. ) ;
#13891=ORIENTED_EDGE ( 'NONE', *, *, #20725, .F. ) ;
#13892=DIRECTION ( 'NONE',  ( -0.000000000000000000, -1.000000000000000000, -0.000000000000000000 ) ) ;
#13901=CARTESIAN_POINT ( 'NONE',  ( -6.401811138932623990, 38.95166772950821610, 55.13648753466793551 ) ) ;
#13902=CARTESIAN_POINT ( 'NONE',  ( -4.274778969419686270, 39.88689869269535393, 51.75995440011182325 ) ) ;
#13905=AXIS2_PLACEMENT_3D ( 'NONE', #12083, #15731, #8526 ) ;
#13906=CARTESIAN_POINT ( 'NONE',  ( -90.00000000000000000, 28.00000000000000000, -9.108981535246192915E-16 ) ) ;
#13907=ORIENTED_EDGE ( 'NONE', *, *, #20821, .T. ) ;
#13909=ORIENTED_EDGE ( 'NONE', *, *, #6122, .F. ) ;
#13914=CARTESIAN_POINT ( 'NONE',  ( -10.34137811700568932, 39.99999999999998579, -53.75702834151140763 ) ) ;
#13916=CARTESIAN_POINT ( 'NONE',  ( 5.042540895202911599, 39.84191929402975774, 52.23966295474247090 ) ) ;
#13917=ORIENTED_EDGE ( 'NONE', *, *, #17385, .F. ) ;
#13919=CARTESIAN_POINT ( 'NONE',  ( 35.00000000000000000, 2.142135623730931471, 4.258610482196280173E-15 ) ) ;
#13923=CARTESIAN_POINT ( 'NONE',  ( 10.72803533576303359, 40.00000000000000711, -53.87712872072452797 ) ) ;
#13927=DIRECTION ( 'NONE',  ( 0.000000000000000000, 0.000000000000000000, 1.000000000000000000 ) ) ;
#13934=CARTESIAN_POINT ( 'NONE',  ( 11.13570271988770877, 40.00000000000000711, -54.01634158485467907 ) ) ;
#13935=VERTEX_POINT ( 'NONE', #5383 ) ;
#13938=CARTESIAN_POINT ( 'NONE',  ( -1.833353995796109137, 34.88982467546053812, -38.89995731584649974 ) ) ;
#13940=CARTESIAN_POINT ( 'NONE',  ( -20.00279574339814559, 20.27588806490366125, -58.14815718763279762 ) ) ;
#13943=CARTESIAN_POINT ( 'NONE',  ( -34.99999999999980815, 28.00000000000000000, 57.49999999999921840 ) ) ;
#13947=EDGE_CURVE ( 'NONE', #249, #9389, #12284, .T. ) ;
#13954=EDGE_LOOP ( 'NONE', ( #16989, #9764, #16502, #12060, #12446, #21890 ) ) ;
#13956=CARTESIAN_POINT ( 'NONE',  ( 6.976853941411403248, 1.175947842326362069, -53.23020196595923181 ) ) ;
#13965=CARTESIAN_POINT ( 'NONE',  ( 21.20802570598056036, 27.37171784732025515, -58.39394879075534561 ) ) ;
#13967=DIRECTION ( 'NONE',  ( 0.000000000000000000, 0.000000000000000000, 1.000000000000000000 ) ) ;
#13968=CARTESIAN_POINT ( 'NONE',  ( 8.197131407637472833, 40.00000000000000711, 53.04141934721033635 ) ) ;
#13969=CARTESIAN_POINT ( 'NONE',  ( 12.70473862104218021, 28.00863069209355416, -44.75655646380167951 ) ) ;
#13970=VERTEX_POINT ( 'NONE', #9041 ) ;
#13971=LINE ( 'NONE', #20889, #8285 ) ;
#13972=CARTESIAN_POINT ( 'NONE',  ( -19.23435001722038251, 8.416038526954890742, 57.89219688981300749 ) ) ;
#13976=VERTEX_POINT ( 'NONE', #21303 ) ;
#13979=FACE_BOUND ( 'NONE', #7602, .T. ) ;
#13985=CARTESIAN_POINT ( 'NONE',  ( 8.743619455145315911, 40.00000000000000711, 53.24632774152720316 ) ) ;
#13987=FACE_BOUND ( 'NONE', #3962, .T. ) ;
#13990=CARTESIAN_POINT ( 'NONE',  ( -5.833333333333337478, 6.180730040185833829, -40.61164310337066041 ) ) ;
#13991=CARTESIAN_POINT ( 'NONE',  ( -8.566020585660502861E-14, -3.670992598665648643, 46.55272505131122074 ) ) ;
#13999=CIRCLE ( 'NONE', #5973, 17.00000000000001421 ) ;
#14000=B_SPLINE_CURVE_WITH_KNOTS ( 'NONE', 3,
 ( #9209, #16187, #496, #7495, #10680, #8981, #15962, #12000, #22000, #8020, #14978, #11099, #7781, #9511, #14534, #18091, #21545, #2525, #13150, #13031, #5843, #11338, #9727, #6292, #18323, #12810, #9612, #7901, #14646, #6186, #798, #14755, #20163, #2405, #12920, #4583, #4238, #18213, #21770, #11562, #14864 ),
 .UNSPECIFIED., .F., .F.,
 ( 4, 1, 1, 1, 1, 2, 2, 1, 1, 1, 1, 2, 2, 1, 1, 1, 2, 2, 1, 1, 1, 2, 2, 1, 1, 1, 2, 2, 4 ),
 ( 0.000000000000000000, 0.06250000000000577316, 0.09375000000000836831, 0.1093750000000093675, 0.1171875000000101585, 0.1210937500000100614, 0.1250000000000099643, 0.1875000000000074385, 0.2187500000000063283, 0.2343750000000055234, 0.2421875000000053568, 0.2460937500000053846, 0.2500000000000053846, 0.3125000000000038858, 0.3437500000000032196, 0.3593750000000023870, 0.3671875000000019984, 0.3750000000000016098, 0.4375000000000014433, 0.4687500000000018874, 0.4843750000000021094, 0.4921875000000017208, 0.5000000000000013323, 0.6249999999999993339, 0.6874999999999983347, 0.7187499999999977796, 0.7343749999999975575, 0.7499999999999973355, 1.000000000000000000 ),
 .UNSPECIFIED. ) ;
#14001=CARTESIAN_POINT ( 'NONE',  ( 19.02718446893024407, 26.17927818497044612, 57.88297158504753526 ) ) ;
#14002=LINE ( 'NONE', #1890, #20240 ) ;
#14003=TOROIDAL_SURFACE ( 'NONE', #11472, 18.00000000000000355, 4.000000000000000000 ) ;
#14005=DIRECTION ( 'NONE',  ( -0.000000000000000000, -0.000000000000000000, -1.000000000000000000 ) ) ;
#14011=ORIENTED_EDGE ( 'NONE', *, *, #1067, .F. ) ;
#14013=DIRECTION ( 'NONE',  ( -0.000000000000000000, -0.000000000000000000, 1.000000000000000000 ) ) ;
#14014=VECTOR ( 'NONE', #9119, 1000.000000000000114 ) ;
#14015=AXIS2_PLACEMENT_3D ( 'NONE', #18078, #9716, #7663 ) ;
#14017=LINE ( 'NONE', #2011, #2134 ) ;
#14018=CARTESIAN_POINT ( 'NONE',  ( 4.516277899324447453, 39.87315172198108826, 51.91186086883033113 ) ) ;
#14021=ORIENTED_EDGE ( 'NONE', *, *, #1550, .T. ) ;
#14022=CARTESIAN_POINT ( 'NONE',  ( 35.00000000000058265, 40.00000000000000000, -55.00000000000076028 ) ) ;
#14024=CYLINDRICAL_SURFACE ( 'NONE', #17499, 6.499999999999999112 ) ;
#14027=CIRCLE ( 'NONE', #2347, 30.00000000000000000 ) ;
#14030=CARTESIAN_POINT ( 'NONE',  ( -6.803227178529575703, 38.81166136533716582, 55.43135129401769490 ) ) ;
#14031=EDGE_CURVE ( 'NONE', #12228, #22506, #21075, .T. ) ;
#14034=VECTOR ( 'NONE', #18335, 1000.000000000000000 ) ;
#14035=ORIENTED_EDGE ( 'NONE', *, *, #18258, .T. ) ;
#14037=ADVANCED_FACE ( 'NONE', ( #6993, #334 ), #5276, .T. ) ;
#14041=AXIS2_PLACEMENT_3D ( 'NONE', #9291, #16269, #3696 ) ;
#14042=CYLINDRICAL_SURFACE ( 'NONE', #4694, 9.000000000000003553 ) ;
#14044=FACE_BOUND ( 'NONE', #3311, .T. ) ;
#14046=CARTESIAN_POINT ( 'NONE',  ( -42.50000000000000711, -9.600000000000001421, -47.50000000000000000 ) ) ;
#14048=CARTESIAN_POINT ( 'NONE',  ( -14.77818138858748931, 33.48299671873984806, -59.09975138256963589 ) ) ;
#14050=ORIENTED_EDGE ( 'NONE', *, *, #7174, .F. ) ;
#14053=EDGE_CURVE ( 'NONE', #6208, #6579, #21414, .T. ) ;
#14056=EDGE_LOOP ( 'NONE', ( #3800, #7941, #9686, #22037 ) ) ;
#14057=ADVANCED_FACE ( 'NONE', ( #16248 ), #20044, .T. ) ;
#14059=DIRECTION ( 'NONE',  ( -1.000000000000000000, 0.000000000000000000, 0.000000000000000000 ) ) ;
#14060=LINE ( 'NONE', #19586, #8264 ) ;
#14061=B_SPLINE_CURVE_WITH_KNOTS ( 'NONE', 1,
 ( #21330, #15930 ),
 .UNSPECIFIED., .F., .F.,
 ( 2, 2 ),
 ( 0.000000000000000000, 1.000000000000000000 ),
 .UNSPECIFIED. ) ;
#14064=VECTOR ( 'NONE', #16480, 1000.000000000000114 ) ;
#14065=EDGE_CURVE ( 'NONE', #18120, #15589, #3488, .T. ) ;
#14070=DIRECTION ( 'NONE',  ( -0.000000000000000000, -0.000000000000000000, 1.000000000000000000 ) ) ;
#14077=CYLINDRICAL_SURFACE ( 'NONE', #14877, 2.499999999999998668 ) ;
#14078=CARTESIAN_POINT ( 'NONE',  ( -6.696867368503558448E-15, 40.00000000000000000, -48.73397172404479960 ) ) ;
#14079=AXIS2_PLACEMENT_3D ( 'NONE', #18999, #16924, #15528 ) ;
#14082=ORIENTED_EDGE ( 'NONE', *, *, #19291, .T. ) ;
#14084=CARTESIAN_POINT ( 'NONE',  ( -35.00000000000000000, -9.000000000000001776, -8.999999999999989342 ) ) ;
#14085=VERTEX_POINT ( 'NONE', #18315 ) ;
#14087=FACE_OUTER_BOUND ( 'NONE', #16517, .T. ) ;
#14090=AXIS2_PLACEMENT_3D ( 'NONE', #13445, #1203, #13666 ) ;
#14091=VECTOR ( 'NONE', #3897, 1000.000000000000000 ) ;
#14092=EDGE_LOOP ( 'NONE', ( #16301, #745, #3190, #8471 ) ) ;
#14094=VERTEX_POINT ( 'NONE', #792 ) ;
#14098=ORIENTED_EDGE ( 'NONE', *, *, #9867, .T. ) ;
#14099=CARTESIAN_POINT ( 'NONE',  ( -35.00000000000058265, 40.00000000000000000, -55.00000000000076028 ) ) ;
#14102=CARTESIAN_POINT ( 'NONE',  ( 5.890136539964617057, 39.99999999999999289, 52.04311943146325348 ) ) ;
#14104=FACE_OUTER_BOUND ( 'NONE', #535, .T. ) ;
#14105=CARTESIAN_POINT ( 'NONE',  ( -1.387778780781445676E-14, 20.00000000000000000, 102.0000000000000142 ) ) ;
#14108=CARTESIAN_POINT ( 'NONE',  ( -7.544777747232855880, -0.4935208846046454934, 52.99868632946503766 ) ) ;
#14113=ORIENTED_EDGE ( 'NONE', *, *, #9724, .F. ) ;
#14118=DIRECTION ( 'NONE',  ( 0.000000000000000000, 0.000000000000000000, -1.000000000000000000 ) ) ;
#14120=CARTESIAN_POINT ( 'NONE',  ( 15.62751878813134532, 32.48885827236527035, 59.38785559521994628 ) ) ;
#14123=CIRCLE ( 'NONE', #9023, 58.99999999999994316 ) ;
#14127=B_SPLINE_CURVE_WITH_KNOTS ( 'NONE', 3,
 ( #19832, #11108, #12707, #17644, #12476, #21206, #16038, #19601, #7564, #19488, #8938, #14305, #3794, #17987, #17761, #16140, #1953, #14543, #2067, #348, #12928, #7337, #21553, #3911, #10878, #2183, #2870, #1030, #2754, #16723, #8134, #20060, #7911, #18328, #21897, #14985, #9736, #13489, #16842, #9951, #14763 ),
 .UNSPECIFIED., .F., .F.,
 ( 4, 1, 1, 1, 1, 2, 2, 1, 1, 1, 1, 2, 2, 1, 1, 1, 2, 2, 1, 1, 1, 2, 2, 1, 1, 1, 2, 2, 4 ),
 ( 0.000000000000000000, 0.06250000000000066613, 0.09375000000000077716, 0.1093750000000005412, 0.1171875000000003331, 0.1210937500000000278, 0.1249999999999997224, 0.1874999999999943101, 0.2187499999999919509, 0.2343749999999911182, 0.2421874999999908129, 0.2460937499999905353, 0.2499999999999902855, 0.3124999999999911737, 0.3437499999999912292, 0.3593749999999912847, 0.3671874999999913958, 0.3749999999999915623, 0.4374999999999924505, 0.4687499999999932276, 0.4843749999999932832, 0.4921874999999932832, 0.4999999999999933387, 0.6249999999999938938, 0.6874999999999937828, 0.7187499999999942268, 0.7343749999999944489, 0.7499999999999947820, 1.000000000000000000 ),
 .UNSPECIFIED. ) ;
#14129=ORIENTED_EDGE ( 'NONE', *, *, #11016, .T. ) ;
#14135=CARTESIAN_POINT ( 'NONE',  ( 0.03423019660800662167, 39.99999309938340275, 48.76060158720252957 ) ) ;
#14137=CARTESIAN_POINT ( 'NONE',  ( -34.99999999999980815, 40.00000000000000711, 57.52499999999922409 ) ) ;
#14138=VECTOR ( 'NONE', #10312, 1000.000000000000000 ) ;
#14140=DIRECTION ( 'NONE',  ( -0.000000000000000000, 1.000000000000000000, -0.000000000000000000 ) ) ;
#14142=VECTOR ( 'NONE', #12796, 1000.000000000000000 ) ;
#14143=CARTESIAN_POINT ( 'NONE',  ( -7.505578006075234399, 1.461761173328249175, -55.63523492904088386 ) ) ;
#14144=CARTESIAN_POINT ( 'NONE',  ( -17.21151300967881426, 30.19805602791846155, 59.88250013944312400 ) ) ;
#14148=DIRECTION ( 'NONE',  ( -0.000000000000000000, -1.000000000000000000, -0.000000000000000000 ) ) ;
#14158=CARTESIAN_POINT ( 'NONE',  ( 7.480086125711145506, -0.2526605362862675563, -53.02285530597580276 ) ) ;
#14160=CARTESIAN_POINT ( 'NONE',  ( -30.00000000000001421, 20.00000000000000355, 105.0000000000000142 ) ) ;
#14164=CARTESIAN_POINT ( 'NONE',  ( -11.57708680448422101, 39.19108614651867839, -55.24531487870292068 ) ) ;
#14171=DIRECTION ( 'NONE',  ( 1.000000000000000000, 0.000000000000000000, 0.000000000000000000 ) ) ;
#14172=DIRECTION ( 'NONE',  ( 0.000000000000000000, 0.000000000000000000, 1.000000000000000000 ) ) ;
#14173=EDGE_CURVE ( 'NONE', #12233, #11729, #22130, .T. ) ;
#14174=CARTESIAN_POINT ( 'NONE',  ( -34.99999999999980815, 28.00000000000000000, 52.49999999999922551 ) ) ;
#14179=ORIENTED_EDGE ( 'NONE', *, *, #2232, .T. ) ;
#14180=CIRCLE ( 'NONE', #4342, 9.000000000000003553 ) ;
#14189=CARTESIAN_POINT ( 'NONE',  ( 35.00000000000000000, -4.999999999999997335, 57.00000000000002842 ) ) ;
#14196=DIRECTION ( 'NONE',  ( 0.000000000000000000, 0.000000000000000000, -1.000000000000000000 ) ) ;
#14199=DIRECTION ( 'NONE',  ( -0.000000000000000000, 1.000000000000000000, -0.000000000000000000 ) ) ;
#14200=CARTESIAN_POINT ( 'NONE',  ( -8.923978417721194489, 2.083761144194138826, 56.51262908348098790 ) ) ;
#14203=EDGE_CURVE ( 'NONE', #21010, #10333, #9605, .T. ) ;
#14204=CARTESIAN_POINT ( 'NONE',  ( -1.107481333971237270, 39.99270069144557027, -49.57628751188472194 ) ) ;
#14208=LINE ( 'NONE', #21444, #15469 ) ;
#14212=ORIENTED_EDGE ( 'NONE', *, *, #9608, .F. ) ;
#14214=VERTEX_POINT ( 'NONE', #18885 ) ;
#14217=DIRECTION ( 'NONE',  ( 0.000000000000000000, 0.000000000000000000, -1.000000000000000000 ) ) ;
#14218=CARTESIAN_POINT ( 'NONE',  ( 8.774784205810801652, 39.47271969504190281, -54.19450391025852554 ) ) ;
#14223=EDGE_LOOP ( 'NONE', ( #14325, #14968, #15563 ) ) ;
#14226=CARTESIAN_POINT ( 'NONE',  ( 34.99999999999980815, 40.00000000000000711, 57.52499999999922409 ) ) ;
#14233=DIRECTION ( 'NONE',  ( -0.000000000000000000, -1.000000000000000000, -0.000000000000000000 ) ) ;
#14234=DIRECTION ( 'NONE',  ( 0.000000000000000000, 0.000000000000000000, 1.000000000000000000 ) ) ;
#14235=AXIS2_PLACEMENT_3D ( 'NONE', #4113, #11084, #2391 ) ;
#14236=CARTESIAN_POINT ( 'NONE',  ( 19.97206123483663731, 21.14267036293957247, 58.14006880918460496 ) ) ;
#14237=DIRECTION ( 'NONE',  ( 0.000000000000000000, 0.7071067811866457165, 0.7071067811864494290 ) ) ;
#14238=ADVANCED_FACE ( 'NONE', ( #3193 ), #15422, .F. ) ;
#14241=ORIENTED_EDGE ( 'NONE', *, *, #4469, .T. ) ;
#14242=AXIS2_PLACEMENT_3D ( 'NONE', #226, #14070, #17876 ) ;
#14243=ORIENTED_EDGE ( 'NONE', *, *, #11800, .T. ) ;
#14248=DIRECTION ( 'NONE',  ( -0.000000000000000000, -0.000000000000000000, 1.000000000000000000 ) ) ;
#14253=LINE ( 'NONE', #4161, #22283 ) ;
#14254=CARTESIAN_POINT ( 'NONE',  ( 4.556497390243006151, 39.87079205654652725, 51.93698194406282198 ) ) ;
#14256=DIRECTION ( 'NONE',  ( 0.000000000000000000, 0.7071067811865474617, 0.7071067811865474617 ) ) ;
#14258=CYLINDRICAL_SURFACE ( 'NONE', #7626, 2.099999999999997868 ) ;
#14259=CARTESIAN_POINT ( 'NONE',  ( -5.833333333333325932, 40.00000000000000000, 40.61164310337068883 ) ) ;
#14260=CARTESIAN_POINT ( 'NONE',  ( -10.99584631063759588, 3.272668205460579127, -57.61971594758655613 ) ) ;
#14261=APPLICATION_CONTEXT ( 'automotive_design' ) ;
#14262=EDGE_CURVE ( 'NONE', #22326, #19879, #10038, .T. ) ;
#14264=DIRECTION ( 'NONE',  ( -0.000000000000000000, -1.000000000000000000, -0.000000000000000000 ) ) ;
#14265=DIRECTION ( 'NONE',  ( -0.000000000000000000, -1.000000000000000000, -0.000000000000000000 ) ) ;
#14266=DIRECTION ( 'NONE',  ( 1.000000000000000000, 0.000000000000000000, -1.224646799147353207E-16 ) ) ;
#14267=VERTEX_POINT ( 'NONE', #1016 ) ;
#14268=EDGE_LOOP ( 'NONE', ( #4803, #17475, #2770, #22059 ) ) ;
#14269=ORIENTED_EDGE ( 'NONE', *, *, #19340, .T. ) ;
#14271=AXIS2_PLACEMENT_3D ( 'NONE', #15010, #5983, #11364 ) ;
#14276=EDGE_CURVE ( 'NONE', #16403, #20378, #22100, .T. ) ;
#14277=CARTESIAN_POINT ( 'NONE',  ( -14.84934717125631920, 6.596698521592471387, 59.12425370493867405 ) ) ;
#14281=EDGE_CURVE ( 'NONE', #3949, #21644, #18841, .T. ) ;
#14284=LINE ( 'NONE', #12682, #3423 ) ;
#14285=DIRECTION ( 'NONE',  ( 1.000000000000000000, 0.000000000000000000, 0.000000000000000000 ) ) ;
#14286=LINE ( 'NONE', #21530, #14064 ) ;
#14292=DIRECTION ( 'NONE',  ( 0.000000000000000000, 0.000000000000000000, 1.000000000000000000 ) ) ;
#14293=CARTESIAN_POINT ( 'NONE',  ( 16.25447798254043263, 8.309829536807932016, -57.03340146943282463 ) ) ;
#14295=ORIENTED_EDGE ( 'NONE', *, *, #4056, .F. ) ;
#14297=CIRCLE ( 'NONE', #10633, 9.000000000000003553 ) ;
#14299=ORIENTED_EDGE ( 'NONE', *, *, #12132, .T. ) ;
#14302=LINE ( 'NONE', #110, #2149 ) ;
#14305=CARTESIAN_POINT ( 'NONE',  ( -7.725157334975624401, 39.99999999999999289, 52.85293811915976647 ) ) ;
#14309=CARTESIAN_POINT ( 'NONE',  ( 19.23435001722034698, 8.416038526954860544, -57.89219688981297907 ) ) ;
#14311=EDGE_CURVE ( 'NONE', #22510, #21245, #3844, .T. ) ;
#14313=ORIENTED_EDGE ( 'NONE', *, *, #22285, .T. ) ;
#14316=CARTESIAN_POINT ( 'NONE',  ( -0.9607552338323060992, 39.99453550393771906, -49.46704700291807910 ) ) ;
#14318=CYLINDRICAL_SURFACE ( 'NONE', #21520, 30.00000000000000000 ) ;
#14323=EDGE_LOOP ( 'NONE', ( #18073, #7335, #21859, #15759 ) ) ;
#14325=ORIENTED_EDGE ( 'NONE', *, *, #18498, .F. ) ;
#14327=ADVANCED_FACE ( 'NONE', ( #19113 ), #12224, .F. ) ;
#14328=ORIENTED_EDGE ( 'NONE', *, *, #14532, .T. ) ;
#14331=AXIS2_PLACEMENT_3D ( 'NONE', #18680, #9623, #20401 ) ;
#14332=CARTESIAN_POINT ( 'NONE',  ( 7.259797106483209639, 39.65417185066220895, -53.48039442441829294 ) ) ;
#14333=CARTESIAN_POINT ( 'NONE',  ( 7.248955570856898234, 40.00000000000000000, 52.65401626641859423 ) ) ;
#14334=ORIENTED_EDGE ( 'NONE', *, *, #540, .F. ) ;
#14339=CARTESIAN_POINT ( 'NONE',  ( 1.607210943102148261E-12, -4.184048734395063640, 46.01969553071018026 ) ) ;
#14340=CARTESIAN_POINT ( 'NONE',  ( -42.50000000000000711, -12.00000000000000000, 47.50000000000000711 ) ) ;
#14341=ORIENTED_EDGE ( 'NONE', *, *, #14554, .T. ) ;
#14342=CARTESIAN_POINT ( 'NONE',  ( -0.05288783471921253143, -1.234056376215194817, 48.20419181041120993 ) ) ;
#14346=CARTESIAN_POINT ( 'NONE',  ( -5.666031183648452263, 39.18449859167989757, 54.55698311759263675 ) ) ;
#14348=ORIENTED_EDGE ( 'NONE', *, *, #2125, .F. ) ;
#14349=CARTESIAN_POINT ( 'NONE',  ( 20.11656324090261450, 10.00164725896550522, 58.12608834080169373 ) ) ;
#14350=CARTESIAN_POINT ( 'NONE',  ( 7.088850870549147224E-15, -5.000000000000000000, 44.98888751680801334 ) ) ;
#14351=ADVANCED_FACE ( 'NONE', ( #3539 ), #17730, .F. ) ;
#14352=AXIS2_PLACEMENT_3D ( 'NONE', #9616, #7910, #13156 ) ;
#14353=FACE_OUTER_BOUND ( 'NONE', #19099, .T. ) ;
#14357=ORIENTED_EDGE ( 'NONE', *, *, #6390, .F. ) ;
#14359=ORIENTED_EDGE ( 'NONE', *, *, #10148, .T. ) ;
#14367=B_SPLINE_CURVE_WITH_KNOTS ( 'NONE', 3,
 ( #14694, #11264, #22044, #2796, #6338, #20212 ),
 .UNSPECIFIED., .F., .F.,
 ( 4, 2, 4 ),
 ( 4.605519509344441270E-20, 0.005389490931282739546, 0.01077898186256547909 ),
 .UNSPECIFIED. ) ;
#14373=AXIS2_PLACEMENT_3D ( 'NONE', #21186, #5488, #5710 ) ;
#14380=CARTESIAN_POINT ( 'NONE',  ( 42.50000000000000711, -5.000000000000000000, -47.50000000000000000 ) ) ;
#14381=ORIENTED_EDGE ( 'NONE', *, *, #10991, .T. ) ;
#14382=ORIENTED_EDGE ( 'NONE', *, *, #18549, .T. ) ;
#14386=CARTESIAN_POINT ( 'NONE',  ( -42.50000000000000711, -5.000000000000000000, -41.00000000000000000 ) ) ;
#14397=ORIENTED_EDGE ( 'NONE', *, *, #2047, .T. ) ;
#14399=EDGE_CURVE ( 'NONE', #19879, #16727, #1669, .T. ) ;
#14404=CIRCLE ( 'NONE', #21028, 2.099999999999990763 ) ;
#14405=ORIENTED_EDGE ( 'NONE', *, *, #11267, .T. ) ;
#14407=CARTESIAN_POINT ( 'NONE',  ( -20.00000000000001421, 20.00000000000000000, 60.00200000000000244 ) ) ;
#14408=DIRECTION ( 'NONE',  ( -0.000000000000000000, -1.000000000000000000, -0.000000000000000000 ) ) ;
#14409=B_SPLINE_CURVE_WITH_KNOTS ( 'NONE', 1,
 ( #17770, #15924 ),
 .UNSPECIFIED., .F., .F.,
 ( 2, 2 ),
 ( 0.000000000000000000, 1.000000000000000000 ),
 .UNSPECIFIED. ) ;
#14411=LINE ( 'NONE', #5720, #6382 ) ;
#14414=EDGE_CURVE ( 'NONE', #7816, #6097, #927, .T. ) ;
#14415=AXIS2_PLACEMENT_3D ( 'NONE', #13871, #5190, #12167 ) ;
#14417=DIRECTION ( 'NONE',  ( 0.000000000000000000, 0.000000000000000000, -1.000000000000000000 ) ) ;
#14418=CARTESIAN_POINT ( 'NONE',  ( -12.09218358684865002, 1.291952833854525196, 55.42846997241219498 ) ) ;
#14420=CARTESIAN_POINT ( 'NONE',  ( 34.99999999999980815, 28.00000000000000000, 57.09999999999921982 ) ) ;
#14421=CARTESIAN_POINT ( 'NONE',  ( -10.62139969368320891, 0.6004703193304483655, -54.70636795414683462 ) ) ;
#14424=CARTESIAN_POINT ( 'NONE',  ( 23.49999999999998579, 19.99999999999999645, -105.0000000000000142 ) ) ;
#14425=CARTESIAN_POINT ( 'NONE',  ( 35.00000000000000000, 40.00000000000000000, -59.99999999999999289 ) ) ;
#14427=ORIENTED_EDGE ( 'NONE', *, *, #14483, .T. ) ;
#14428=DIRECTION ( 'NONE',  ( 0.000000000000000000, 0.000000000000000000, 1.000000000000000000 ) ) ;
#14430=CARTESIAN_POINT ( 'NONE',  ( -8.349099696861312481, 1.803277857259544925, 53.93591755799873511 ) ) ;
#14431=CARTESIAN_POINT ( 'NONE',  ( -1.076297586510878146, 39.99310908795442288, -49.55312039312080685 ) ) ;
#14432=AXIS2_PLACEMENT_3D ( 'NONE', #11882, #2969, #8896 ) ;
#14448=ORIENTED_EDGE ( 'NONE', *, *, #7650, .T. ) ;
#14449=FACE_OUTER_BOUND ( 'NONE', #21856, .T. ) ;
#14451=ORIENTED_EDGE ( 'NONE', *, *, #9671, .F. ) ;
#14452=B_SPLINE_CURVE_WITH_KNOTS ( 'NONE', 3,
 ( #8273, #15243, #4621, #9651, #14795, #18471, #22033, #947, #20431, #6327, #21812, #8162, #18706, #2786, #4283, #6444, #831, #19974, #9769, #16758, #4395, #22264, #9979, #18354 ),
 .UNSPECIFIED., .F., .F.,
 ( 4, 2, 2, 2, 2, 2, 2, 2, 2, 2, 2, 4 ),
 ( 0.02614117015034102959, 0.02729036340605314054, 0.02843955666176525149, 0.03073794317318947686, 0.03188713642890158434, 0.03303632968461369529, 0.03533471619603791025, 0.03648390945175002814, 0.03763310270746213909, 0.03993148921888636793, 0.04222987573031060371, 0.04452826224173483255 ),
 .UNSPECIFIED. ) ;
#14455=DIRECTION ( 'NONE',  ( -0.000000000000000000, -0.000000000000000000, -1.000000000000000000 ) ) ;
#14457=ADVANCED_FACE ( 'NONE', ( #13660 ), #17012, .F. ) ;
#14458=CARTESIAN_POINT ( 'NONE',  ( -5.833333333333339255, 0.000000000000000000, -40.61164310337066041 ) ) ;
#14459=CARTESIAN_POINT ( 'NONE',  ( 1.427811580246491241, 39.96253266219668632, -50.08434179903181160 ) ) ;
#14462=CARTESIAN_POINT ( 'NONE',  ( -13.00000000000011546, 42.51666049839536043, 105.0000000000000142 ) ) ;
#14465=CARTESIAN_POINT ( 'NONE',  ( 34.99999999999980815, 40.00000000000000711, 57.52499999999922409 ) ) ;
#14466=CARTESIAN_POINT ( 'NONE',  ( 19.27384183542241658, 25.35969264784004906, 57.95172789105618705 ) ) ;
#14472=CARTESIAN_POINT ( 'NONE',  ( 15.21899206303239360, 36.51951236530284461, -56.65045400726858560 ) ) ;
#14473=ORIENTED_EDGE ( 'NONE', *, *, #18385, .F. ) ;
#14475=ORIENTED_EDGE ( 'NONE', *, *, #21082, .F. ) ;
#14480=CARTESIAN_POINT ( 'NONE',  ( -11.12045539163121255, 39.12082365984661436, -55.06303111106303305 ) ) ;
#14481=CONICAL_SURFACE ( 'NONE', #2058, 2.099999999999997868, 1.029744258676653867 ) ;
#14483=EDGE_CURVE ( 'NONE', #12228, #5921, #15258, .T. ) ;
#14484=VERTEX_POINT ( 'NONE', #8091 ) ;
#14485=CARTESIAN_POINT ( 'NONE',  ( -10.06223851446356043, 39.28158160658968967, -54.67678195792213813 ) ) ;
#14488=EDGE_CURVE ( 'NONE', #18025, #3688, #13707, .T. ) ;
#14491=CYLINDRICAL_SURFACE ( 'NONE', #1782, 2.500000000000002220 ) ;
#14505=ADVANCED_FACE ( 'NONE', ( #10209, #4744 ), #20433, .F. ) ;
#14508=CARTESIAN_POINT ( 'NONE',  ( -7.505578006075234399, 1.461761173328249175, -55.63523492904088386 ) ) ;
#14511=CARTESIAN_POINT ( 'NONE',  ( -42.50000000000000711, -9.600000000000001421, 47.50000000000000711 ) ) ;
#14513=CARTESIAN_POINT ( 'NONE',  ( -9.165377225651191395, 37.79989650906291132, -54.16098472236620864 ) ) ;
#14520=DIRECTION ( 'NONE',  ( -0.000000000000000000, -1.000000000000000000, -0.000000000000000000 ) ) ;
#14525=CIRCLE ( 'NONE', #12691, 2.524999999999999467 ) ;
#14526=FACE_OUTER_BOUND ( 'NONE', #14673, .T. ) ;
#14528=EDGE_CURVE ( 'NONE', #7376, #15831, #8276, .T. ) ;
#14532=EDGE_CURVE ( 'NONE', #11692, #21115, #14969, .T. ) ;
#14534=CARTESIAN_POINT ( 'NONE',  ( 7.392698783198288659, 40.00000000000000711, -52.71482400407168001 ) ) ;
#14535=ORIENTED_EDGE ( 'NONE', *, *, #15319, .F. ) ;
#14539=CARTESIAN_POINT ( 'NONE',  ( 42.50000000000000711, -5.000000000000000000, 41.00000000000000711 ) ) ;
#14540=VECTOR ( 'NONE', #22329, 1000.000000000000000 ) ;
#14543=CARTESIAN_POINT ( 'NONE',  ( -7.130208587515866725, 39.99999999999998579, 52.60396388218742203 ) ) ;
#14544=VERTEX_POINT ( 'NONE', #2788 ) ;
#14550=LINE ( 'NONE', #14770, #20015 ) ;
#14552=CARTESIAN_POINT ( 'NONE',  ( -0.5415566488456911021, 39.99826507375607321, -49.15084919631396332 ) ) ;
#14553=ORIENTED_EDGE ( 'NONE', *, *, #3289, .T. ) ;
#14554=EDGE_CURVE ( 'NONE', #3760, #10900, #8961, .T. ) ;
#14558=AXIS2_PLACEMENT_3D ( 'NONE', #3149, #12079, #10119 ) ;
#14559=VECTOR ( 'NONE', #20465, 1000.000000000000000 ) ;
#14561=ORIENTED_EDGE ( 'NONE', *, *, #3684, .T. ) ;
#14570=EDGE_LOOP ( 'NONE', ( #5576, #10270 ) ) ;
#14572=CARTESIAN_POINT ( 'NONE',  ( 90.00000000000000000, 39.97500000000000142, -2.500000000000003109 ) ) ;
#14577=CARTESIAN_POINT ( 'NONE',  ( -18.74703631669237680, 7.639653230112246618, -57.75728470191489095 ) ) ;
#14581=EDGE_LOOP ( 'NONE', ( #15835, #13135, #2794, #14050 ) ) ;
#14585=DIRECTION ( 'NONE',  ( -1.000000000000000000, 0.000000000000000000, 0.000000000000000000 ) ) ;
#14588=ORIENTED_EDGE ( 'NONE', *, *, #18029, .T. ) ;
#14589=DIRECTION ( 'NONE',  ( 0.000000000000000000, -1.000000000000000000, 0.000000000000000000 ) ) ;
#14590=CARTESIAN_POINT ( 'NONE',  ( 90.00000000000000000, 28.00000000000000000, -2.500000000000003109 ) ) ;
#14601=CARTESIAN_POINT ( 'NONE',  ( -11.52370268861635161, 39.05614286682681779, -55.22012726398858717 ) ) ;
#14603=VERTEX_POINT ( 'NONE', #6565 ) ;
#14604=CARTESIAN_POINT ( 'NONE',  ( -11.51194040401124319, 39.05862814753013623, -55.21283662269279091 ) ) ;
#14609=DIRECTION ( 'NONE',  ( 0.000000000000000000, 0.000000000000000000, -1.000000000000000000 ) ) ;
#14610=CARTESIAN_POINT ( 'NONE',  ( -30.00000000000001421, 20.00000000000000711, -105.0000000000000142 ) ) ;
#14613=CARTESIAN_POINT ( 'NONE',  ( -2.881565232080841810, 39.80724445179826887, 51.34429047750199970 ) ) ;
#14614=CARTESIAN_POINT ( 'NONE',  ( -13.33780792070363219, 2.142135623730927918, -45.06383732350883520 ) ) ;
#14615=ORIENTED_EDGE ( 'NONE', *, *, #20849, .T. ) ;
#14616=EDGE_LOOP ( 'NONE', ( #20223, #17053, #8777, #19089 ) ) ;
#14617=EDGE_CURVE ( 'NONE', #3398, #17095, #16760, .T. ) ;
#14621=LINE ( 'NONE', #21743, #20047 ) ;
#14623=EDGE_CURVE ( 'NONE', #18681, #15589, #22381, .T. ) ;
#14627=CARTESIAN_POINT ( 'NONE',  ( -9.786528823783235964, 39.51685528920044277, -54.52238163179004005 ) ) ;
#14628=CARTESIAN_POINT ( 'NONE',  ( -90.00000000000000000, 28.00000000000000000, 2.099999999999989875 ) ) ;
#14629=DIRECTION ( 'NONE',  ( -0.000000000000000000, 1.000000000000000000, -0.000000000000000000 ) ) ;
#14630=CARTESIAN_POINT ( 'NONE',  ( -1.387778780781445676E-14, 20.00000000000000000, 60.00200000000000244 ) ) ;
#14632=ORIENTED_EDGE ( 'NONE', *, *, #3810, .T. ) ;
#14633=CARTESIAN_POINT ( 'NONE',  ( 10.50000000000024514, -2.516660498395250745, -100.0000000000000000 ) ) ;
#14638=VERTEX_POINT ( 'NONE', #13628 ) ;
#14645=FACE_OUTER_BOUND ( 'NONE', #698, .T. ) ;
#14646=CARTESIAN_POINT ( 'NONE',  ( 4.925985921465350081, 39.99999999999998579, -51.57279956358078010 ) ) ;
#14648=CARTESIAN_POINT ( 'NONE',  ( 0.4054037750498698522, 39.99903173806880829, -49.04694161421060983 ) ) ;
#14649=CARTESIAN_POINT ( 'NONE',  ( 10.06223851446352668, 39.28158160658968967, 54.67678195792215945 ) ) ;
#14651=ORIENTED_EDGE ( 'NONE', *, *, #7245, .T. ) ;
#14653=AXIS2_PLACEMENT_3D ( 'NONE', #22061, #16790, #6355 ) ;
#14654=CARTESIAN_POINT ( 'NONE',  ( -7.505578006075232622, 1.461761173328252283, -55.63523492904088386 ) ) ;
#14655=ORIENTED_EDGE ( 'NONE', *, *, #3992, .F. ) ;
#14657=EDGE_CURVE ( 'NONE', #15589, #16403, #7131, .T. ) ;
#14659=CIRCLE ( 'NONE', #392, 2.099999999999990763 ) ;
#14661=DIRECTION ( 'NONE',  ( 0.000000000000000000, -1.000000000000000000, 0.000000000000000000 ) ) ;
#14664=DIRECTION ( 'NONE',  ( -0.000000000000000000, -0.000000000000000000, 1.000000000000000000 ) ) ;
#14666=DIRECTION ( 'NONE',  ( -0.9012767464701406661, 1.437462578140670496E-16, -0.4332438415860032643 ) ) ;
#14670=CARTESIAN_POINT ( 'NONE',  ( -14.68506606271061443, 23.08193591670981348, 45.68712064066591694 ) ) ;
#14671=CARTESIAN_POINT ( 'NONE',  ( -35.00000000000058265, 26.00000000000000355, -55.00000000000076028 ) ) ;
#14673=EDGE_LOOP ( 'NONE', ( #11012, #22645, #22396, #5035, #370 ) ) ;
#14675=ORIENTED_EDGE ( 'NONE', *, *, #3810, .F. ) ;
#14676=CARTESIAN_POINT ( 'NONE',  ( 12.24033418603698209, 35.84417766536505212, 58.14550894043698293 ) ) ;
#14677=CARTESIAN_POINT ( 'NONE',  ( -13.00000000000011546, 42.51666049839536043, 60.00099999999999767 ) ) ;
#14682=DIRECTION ( 'NONE',  ( 1.000000000000000000, 0.000000000000000000, 0.000000000000000000 ) ) ;
#14686=DIRECTION ( 'NONE',  ( -0.000000000000000000, -1.000000000000000000, -0.000000000000000000 ) ) ;
#14687=AXIS2_PLACEMENT_3D ( 'NONE', #1501, #1730, #7000 ) ;
#14688=CARTESIAN_POINT ( 'NONE',  ( 19.74829075628832697, 16.81150045999882892, -60.56179516789183737 ) ) ;
#14690=DIRECTION ( 'NONE',  ( 0.000000000000000000, -1.000000000000000000, 0.000000000000000000 ) ) ;
#14693=CARTESIAN_POINT ( 'NONE',  ( 7.938322399560873599, 38.36220367130487574, 56.16250688145269976 ) ) ;
#14694=CARTESIAN_POINT ( 'NONE',  ( -4.295527433237782828E-15, -1.236374842841486021, 48.24164917503448180 ) ) ;
#14696=CARTESIAN_POINT ( 'NONE',  ( 11.93214024655333638, 36.05624711372924196, 58.01435237789500121 ) ) ;
#14698=CARTESIAN_POINT ( 'NONE',  ( 14.30127497006473547, 34.01755211514666399, -56.34491176086893205 ) ) ;
#14699=EDGE_CURVE ( 'NONE', #18704, #21119, #4953, .T. ) ;
#14704=EDGE_LOOP ( 'NONE', ( #17432, #13511, #22318, #10641 ) ) ;
#14705=CARTESIAN_POINT ( 'NONE',  ( 10.08226496203362110, 39.27879523430843989, 54.68359763861834466 ) ) ;
#14707=EDGE_CURVE ( 'NONE', #14638, #22326, #21417, .T. ) ;
#14709=EDGE_LOOP ( 'NONE', ( #14299, #16968, #12477, #14970 ) ) ;
#14711=ORIENTED_EDGE ( 'NONE', *, *, #22079, .T. ) ;
#14712=DIRECTION ( 'NONE',  ( 0.000000000000000000, 0.000000000000000000, 1.000000000000000000 ) ) ;
#14713=LINE ( 'NONE', #13326, #14559 ) ;
#14716=CIRCLE ( 'NONE', #12520, 1.999999999999999778 ) ;
#14718=CARTESIAN_POINT ( 'NONE',  ( -1.427812194317577887, 39.96253263129007394, 50.08434126564738165 ) ) ;
#14719=CYLINDRICAL_SURFACE ( 'NONE', #2817, 49.99999999999998579 ) ;
#14720=EDGE_CURVE ( 'NONE', #10179, #1794, #11538, .T. ) ;
#14722=ORIENTED_EDGE ( 'NONE', *, *, #10249, .F. ) ;
#14723=VERTEX_POINT ( 'NONE', #19276 ) ;
#14724=EDGE_CURVE ( 'NONE', #18953, #7816, #8834, .T. ) ;
#14728=CARTESIAN_POINT ( 'NONE',  ( 2.589862425843529881, 0.1394011931330937371, -50.61994180264545662 ) ) ;
#14729=AXIS2_PLACEMENT_3D ( 'NONE', #1862, #5196, #18945 ) ;
#14731=DIRECTION ( 'NONE',  ( -0.000000000000000000, -0.000000000000000000, 1.000000000000000000 ) ) ;
#14733=CARTESIAN_POINT ( 'NONE',  ( -4.750159105397525394, 39.43751337119567779, -52.76321094647789778 ) ) ;
#14746=DIRECTION ( 'NONE',  ( 0.000000000000000000, 0.000000000000000000, 1.000000000000000000 ) ) ;
#14755=CARTESIAN_POINT ( 'NONE',  ( 4.416369897321547278, 40.00000000000000000, -51.31508173270569984 ) ) ;
#14756=VERTEX_POINT ( 'NONE', #10314 ) ;
#14757=CARTESIAN_POINT ( 'NONE',  ( 8.492273976632109367, 39.51732055898253293, -54.09038579245198264 ) ) ;
#14763=CARTESIAN_POINT ( 'NONE',  ( 1.387778780781445676E-14, 40.00000000000000000, 48.73397172404482802 ) ) ;
#14765=CONICAL_SURFACE ( 'NONE', #1601, 15.00000000000000000, 0.7853981633974552734 ) ;
#14766=CARTESIAN_POINT ( 'NONE',  ( -3.997613013123614056, 39.99999999999999289, 51.09533622492809712 ) ) ;
#14767=DIRECTION ( 'NONE',  ( -0.000000000000000000, -0.000000000000000000, -1.000000000000000000 ) ) ;
#14768=EDGE_CURVE ( 'NONE', #19011, #5386, #17425, .T. ) ;
#14770=CARTESIAN_POINT ( 'NONE',  ( -35.00000000000000000, 39.00000000000000711, 50.00000000000000000 ) ) ;
#14773=ORIENTED_EDGE ( 'NONE', *, *, #3170, .F. ) ;
#14775=CIRCLE ( 'NONE', #21745, 30.00000000000000000 ) ;
#14778=EDGE_CURVE ( 'NONE', #15385, #15800, #15919, .T. ) ;
#14779=CIRCLE ( 'NONE', #20627, 51.00000000000002132 ) ;
#14781=EDGE_LOOP ( 'NONE', ( #14675, #19232, #18229, #10773 ) ) ;
#14785=CARTESIAN_POINT ( 'NONE',  ( 19.43416121892454385, 24.82270088923176132, 60.48577746614103035 ) ) ;
#14786=CARTESIAN_POINT ( 'NONE',  ( 6.661198439252276948, -4.819795714535265674, 49.67388352367134985 ) ) ;
#14787=CARTESIAN_POINT ( 'NONE',  ( -10.50000000000012079, 42.51666049839536043, 100.0000000000000000 ) ) ;
#14788=DIRECTION ( 'NONE',  ( 0.000000000000000000, 0.000000000000000000, 1.000000000000000000 ) ) ;
#14790=DIRECTION ( 'NONE',  ( -0.000000000000000000, 1.000000000000000000, -0.000000000000000000 ) ) ;
#14792=LINE ( 'NONE', #20088, #18638 ) ;
#14794=VERTEX_POINT ( 'NONE', #15704 ) ;
#14795=CARTESIAN_POINT ( 'NONE',  ( -14.87996495114181172, 18.06670563205964797, -45.77322900830824892 ) ) ;
#14796=CYLINDRICAL_SURFACE ( 'NONE', #8638, 2.500000000000002220 ) ;
#14798=VERTEX_POINT ( 'NONE', #3468 ) ;
#14799=CARTESIAN_POINT ( 'NONE',  ( -1.387778780781445518E-14, 20.00000000000000355, 105.0000000000000142 ) ) ;
#14800=CARTESIAN_POINT ( 'NONE',  ( 35.00000000000000000, -4.999999999999997335, 4.258610482196280173E-15 ) ) ;
#14801=ORIENTED_EDGE ( 'NONE', *, *, #6047, .T. ) ;
#14802=CARTESIAN_POINT ( 'NONE',  ( 5.204758277554829782, 39.83793674575848343, 52.32476555783389927 ) ) ;
#14803=ORIENTED_EDGE ( 'NONE', *, *, #680, .F. ) ;
#14804=DIRECTION ( 'NONE',  ( -0.000000000000000000, 1.000000000000000000, -0.000000000000000000 ) ) ;
#14810=EDGE_CURVE ( 'NONE', #3413, #9068, #15902, .T. ) ;
#14814=VERTEX_POINT ( 'NONE', #14628 ) ;
#14820=ORIENTED_EDGE ( 'NONE', *, *, #15001, .T. ) ;
#14822=CIRCLE ( 'NONE', #187, 2.499999999999998668 ) ;
#14823=ORIENTED_EDGE ( 'NONE', *, *, #7740, .T. ) ;
#14824=CARTESIAN_POINT ( 'NONE',  ( -42.50000000000000711, -9.600000000000001421, 47.50000000000000711 ) ) ;
#14830=ADVANCED_FACE ( 'NONE', ( #22095 ), #15201, .F. ) ;
#14831=CARTESIAN_POINT ( 'NONE',  ( -4.750178577765296950, 39.43750913335933461, 52.76318739013298398 ) ) ;
#14837=CARTESIAN_POINT ( 'NONE',  ( -17.96966555604169713, 28.82469637350494907, 60.10139901455269040 ) ) ;
#14841=CARTESIAN_POINT ( 'NONE',  ( 8.331955809010601399, 38.18181818181818699, 56.36098470834073026 ) ) ;
#14842=CARTESIAN_POINT ( 'NONE',  ( -9.857944917841409804, 0.2919354798322641997, -54.29891737064848201 ) ) ;
#14844=CIRCLE ( 'NONE', #8654, 2.500000000000002220 ) ;
#14848=EDGE_CURVE ( 'NONE', #9194, #10462, #12287, .T. ) ;
#14852=CARTESIAN_POINT ( 'NONE',  ( 13.56209497734233871, 5.196600802614999459, 56.07847567638239639 ) ) ;
#14864=CARTESIAN_POINT ( 'NONE',  ( -1.387778780781445676E-14, 40.00000000000000000, -48.73397172404481381 ) ) ;
#14866=CARTESIAN_POINT ( 'NONE',  ( 2.217097043154531821, 39.97039924782914966, -50.37983924381441625 ) ) ;
#14869=CARTESIAN_POINT ( 'NONE',  ( 35.00000000000000711, 40.00000000000000000, 58.99999999999995026 ) ) ;
#14871=EDGE_CURVE ( 'NONE', #18756, #1286, #13724, .T. ) ;
#14872=CARTESIAN_POINT ( 'NONE',  ( 11.53082054500845999, 39.05546563731292764, -55.22070542780790703 ) ) ;
#14873=CARTESIAN_POINT ( 'NONE',  ( -9.689843208404422370, 39.33333333333333570, 54.54983754392743833 ) ) ;
#14875=ORIENTED_EDGE ( 'NONE', *, *, #19638, .F. ) ;
#14877=AXIS2_PLACEMENT_3D ( 'NONE', #12478, #19388, #2295 ) ;
#14880=ORIENTED_EDGE ( 'NONE', *, *, #7208, .T. ) ;
#14881=LINE ( 'NONE', #9415, #10892 ) ;
#14882=CARTESIAN_POINT ( 'NONE',  ( -14.50678847729823850, 23.83439465050324912, 45.60743157421821792 ) ) ;
#14884=VECTOR ( 'NONE', #20550, 1000.000000000000114 ) ;
#14885=AXIS2_PLACEMENT_3D ( 'NONE', #14677, #4158, #9085 ) ;
#14887=AXIS2_PLACEMENT_3D ( 'NONE', #6560, #13521, #4839 ) ;
#14888=EDGE_CURVE ( 'NONE', #19609, #3399, #12636, .T. ) ;
#14889=VECTOR ( 'NONE', #2982, 1000.000000000000000 ) ;
#14893=CARTESIAN_POINT ( 'NONE',  ( 18.50805780747142393, 27.59542556733954655, 60.24679276096815528 ) ) ;
#14895=DIRECTION ( 'NONE',  ( 1.000000000000000000, 0.000000000000000000, 0.000000000000000000 ) ) ;
#14896=FACE_OUTER_BOUND ( 'NONE', #16766, .T. ) ;
#14897=CARTESIAN_POINT ( 'NONE',  ( -1.079570778443290191, 5.000568130954873070, -38.73482392062542345 ) ) ;
#14898=ORIENTED_EDGE ( 'NONE', *, *, #2201, .T. ) ;
#14899=DIRECTION ( 'NONE',  ( 0.000000000000000000, 0.000000000000000000, -1.000000000000000000 ) ) ;
#14903=ADVANCED_FACE ( 'NONE', ( #20376 ), #9830, .F. ) ;
#14906=DIRECTION ( 'NONE',  ( -0.000000000000000000, -1.000000000000000000, -0.000000000000000000 ) ) ;
#14909=CARTESIAN_POINT ( 'NONE',  ( 3.210361346424027484, 39.75306810546534564, -52.30715206667685635 ) ) ;
#14913=CARTESIAN_POINT ( 'NONE',  ( -1.438799862756543035, -1.268859023760806837, -49.24077205406572944 ) ) ;
#14914=AXIS2_PLACEMENT_3D ( 'NONE', #16666, #4534, #16999 ) ;
#14919=DIRECTION ( 'NONE',  ( 0.000000000000000000, 0.000000000000000000, 1.000000000000000000 ) ) ;
#14923=CARTESIAN_POINT ( 'NONE',  ( 18.03138881840328978, 11.33611194795357946, -60.11697748794928486 ) ) ;
#14926=AXIS2_PLACEMENT_3D ( 'NONE', #18529, #21555, #4447 ) ;
#14930=AXIS2_PLACEMENT_3D ( 'NONE', #10750, #21091, #17638 ) ;
#14939=DIRECTION ( 'NONE',  ( -0.000000000000000000, 1.000000000000000000, -0.000000000000000000 ) ) ;
#14940=CARTESIAN_POINT ( 'NONE',  ( -35.00000000000000000, 40.00000000000000000, 1.387778780781445676E-14 ) ) ;
#14944=AXIS2_PLACEMENT_3D ( 'NONE', #18306, #5585, #16475 ) ;
#14945=CIRCLE ( 'NONE', #22291, 6.499999999999999112 ) ;
#14950=VERTEX_POINT ( 'NONE', #3411 ) ;
#14953=CARTESIAN_POINT ( 'NONE',  ( -22.40268525210710848, 21.30540434957256934, 58.66274428449824541 ) ) ;
#14954=DIRECTION ( 'NONE',  ( -0.000000000000000000, -0.000000000000000000, 1.000000000000000000 ) ) ;
#14955=MECHANICAL_DESIGN_GEOMETRIC_PRESENTATION_REPRESENTATION('',(#13126),#3995);
#14959=DIRECTION ( 'NONE',  ( 0.000000000000000000, 0.000000000000000000, 1.000000000000000000 ) ) ;
#14960=CARTESIAN_POINT ( 'NONE',  ( 0.7810292038143733517, 39.98537128388858264, 49.65442669227650896 ) ) ;
#14961=CARTESIAN_POINT ( 'NONE',  ( -6.450211378059112377, 39.75599570130062688, -53.02618257463311835 ) ) ;
#14964=DIRECTION ( 'NONE',  ( 0.000000000000000000, 0.000000000000000000, -1.000000000000000000 ) ) ;
#14968=ORIENTED_EDGE ( 'NONE', *, *, #9112, .T. ) ;
#14969=B_SPLINE_CURVE_WITH_KNOTS ( 'NONE', 3,
 ( #13184, #11602, #11488, #10091 ),
 .UNSPECIFIED., .F., .F.,
 ( 4, 4 ),
 ( 0.000000000000000000, 0.0005662878734225370485 ),
 .UNSPECIFIED. ) ;
#14970=ORIENTED_EDGE ( 'NONE', *, *, #9562, .F. ) ;
#14972=DIRECTION ( 'NONE',  ( 0.000000000000000000, 0.000000000000000000, 1.000000000000000000 ) ) ;
#14974=EDGE_CURVE ( 'NONE', #10123, #16148, #15185, .T. ) ;
#14976=CIRCLE ( 'NONE', #21219, 60.00000000000000000 ) ;
#14978=CARTESIAN_POINT ( 'NONE',  ( 8.105735169339924440, 40.00000000000001421, -53.00649291450380929 ) ) ;
#14979=ORIENTED_EDGE ( 'NONE', *, *, #19076, .F. ) ;
#14980=ADVANCED_FACE ( 'NONE', ( #11876, #13690 ), #20707, .T. ) ;
#14985=CARTESIAN_POINT ( 'NONE',  ( -2.580942297915963746, 40.00000000000000000, 50.31086577932750714 ) ) ;
#14987=CARTESIAN_POINT ( 'NONE',  ( -12.68897045256290745, 28.00829229206842186, -44.74667050109236754 ) ) ;
#14994=CARTESIAN_POINT ( 'NONE',  ( -0.05198106984670706338, 39.99998426957630926, -48.77439678740044116 ) ) ;
#14997=AXIS2_PLACEMENT_3D ( 'NONE', #9141, #17959, #17846 ) ;
#15001=EDGE_CURVE ( 'NONE', #1314, #5420, #1298, .T. ) ;
#15006=CARTESIAN_POINT ( 'NONE',  ( 19.99999999999998579, 20.00000000000000711, -60.62177826491069510 ) ) ;
#15007=ADVANCED_FACE ( 'NONE', ( #10266 ), #11998, .T. ) ;
#15008=DIRECTION ( 'NONE',  ( -0.4332438415859278247, 0.000000000000000000, -0.9012767464701768594 ) ) ;
#15010=CARTESIAN_POINT ( 'NONE',  ( -42.50000000000000711, -12.00000000000000000, 47.50000000000000711 ) ) ;
#15011=CARTESIAN_POINT ( 'NONE',  ( 12.92329681834241484, 4.659497110088489435, 58.43073491095716321 ) ) ;
#15014=DIRECTION ( 'NONE',  ( -0.000000000000000000, -1.000000000000000000, -0.000000000000000000 ) ) ;
#15015=CARTESIAN_POINT ( 'NONE',  ( 34.99999999999980815, 39.97500000000000142, 52.49999999999922551 ) ) ;
#15017=DIRECTION ( 'NONE',  ( 0.000000000000000000, 0.000000000000000000, 1.000000000000000000 ) ) ;
#15018=CARTESIAN_POINT ( 'NONE',  ( -15.00000000000001421, 20.00000000000000000, -45.82575694955838230 ) ) ;
#15019=DIRECTION ( 'NONE',  ( 8.659560562354892183E-17, 0.7071067811865507924, -0.7071067811865441310 ) ) ;
#15020=CARTESIAN_POINT ( 'NONE',  ( -42.50000000000000711, -9.600000000000001421, -47.50000000000000000 ) ) ;
#15022=DIRECTION ( 'NONE',  ( 0.000000000000000000, 0.000000000000000000, 1.000000000000000000 ) ) ;
#15023=CARTESIAN_POINT ( 'NONE',  ( 0.1539325450101303450, 40.00000000000000000, -48.91834387730068556 ) ) ;
#15024=VERTEX_POINT ( 'NONE', #6614 ) ;
#15028=ADVANCED_FACE ( 'NONE', ( #4792 ), #8744, .T. ) ;
#15029=CARTESIAN_POINT ( 'NONE',  ( 14.30947201678935699, 34.00909065833927514, 56.34794761833577326 ) ) ;
#15031=CARTESIAN_POINT ( 'NONE',  ( 15.62385314663624669, 32.51590977305029639, -59.38867318806720164 ) ) ;
#15038=DIRECTION ( 'NONE',  ( -0.000000000000000000, -1.000000000000000000, -0.000000000000000000 ) ) ;
#15039=VECTOR ( 'NONE', #8853, 1000.000000000000000 ) ;
#15042=EDGE_LOOP ( 'NONE', ( #3300, #19518, #1848, #17380 ) ) ;
#15047=CARTESIAN_POINT ( 'NONE',  ( 42.50000000000000711, -11.97499999999999964, 47.50000000000000711 ) ) ;
#15049=CARTESIAN_POINT ( 'NONE',  ( -2.995584608082024758, -1.237002266245722515, -50.27666343020536743 ) ) ;
#15053=CARTESIAN_POINT ( 'NONE',  ( -9.144347024359422704, 37.80953375799288807, -56.77060857467738231 ) ) ;
#15054=EDGE_CURVE ( 'NONE', #10705, #10746, #7296, .T. ) ;
#15055=AXIS2_PLACEMENT_3D ( 'NONE', #1677, #19327, #17246 ) ;
#15060=VERTEX_POINT ( 'NONE', #5564 ) ;
#15061=CARTESIAN_POINT ( 'NONE',  ( -16.25447798254661791, 8.309829536803846395, 57.03340146943939004 ) ) ;
#15064=FACE_OUTER_BOUND ( 'NONE', #21175, .T. ) ;
#15066=CARTESIAN_POINT ( 'NONE',  ( 35.00000000000000000, 39.00000000000000711, 4.258610482196280173E-15 ) ) ;
#15067=EDGE_CURVE ( 'NONE', #6177, #10749, #15866, .T. ) ;
#15068=ORIENTED_EDGE ( 'NONE', *, *, #7889, .T. ) ;
#15071=DIRECTION ( 'NONE',  ( -0.000000000000000000, -1.000000000000000000, -0.000000000000000000 ) ) ;
#15072=CARTESIAN_POINT ( 'NONE',  ( -0.6290164960522119930, 40.00000000000000000, -49.48738346577703595 ) ) ;
#15073=ORIENTED_EDGE ( 'NONE', *, *, #356, .T. ) ;
#15076=FACE_BOUND ( 'NONE', #22062, .T. ) ;
#15078=DIRECTION ( 'NONE',  ( 0.000000000000000000, 1.000000000000000000, 0.000000000000000000 ) ) ;
#15083=VECTOR ( 'NONE', #9852, 1000.000000000000114 ) ;
#15085=EDGE_CURVE ( 'NONE', #548, #19255, #9006, .T. ) ;
#15086=ORIENTED_EDGE ( 'NONE', *, *, #16037, .T. ) ;
#15087=CARTESIAN_POINT ( 'NONE',  ( -3.328561921038571736, -3.140496874697064733, 49.62333327021501361 ) ) ;
#15089=ORIENTED_EDGE ( 'NONE', *, *, #3224, .T. ) ;
#15093=CARTESIAN_POINT ( 'NONE',  ( -1.387778780781445518E-14, 20.00000000000000355, -105.0000000000000142 ) ) ;
#15094=CARTESIAN_POINT ( 'NONE',  ( 17.99999999999998579, 20.00000000000000355, 102.0000000000000142 ) ) ;
#15095=DIRECTION ( 'NONE',  ( -0.000000000000000000, 1.000000000000000000, -0.000000000000000000 ) ) ;
#15099=CARTESIAN_POINT ( 'NONE',  ( 14.99999999999998579, 20.38555233723673155, 45.82575694955838941 ) ) ;
#15100=CARTESIAN_POINT ( 'NONE',  ( 2.995584608080545053, -1.237002266245787130, 50.27666343020442241 ) ) ;
#15101=AXIS2_PLACEMENT_3D ( 'NONE', #433, #9385, #670 ) ;
#15103=CARTESIAN_POINT ( 'NONE',  ( -0.06361866581498207274, 39.99997619040497909, -48.78343476366760001 ) ) ;
#15104=AXIS2_PLACEMENT_3D ( 'NONE', #20895, #5412, #13641 ) ;
#15107=DIRECTION ( 'NONE',  ( -1.000000000000000000, 0.000000000000000000, 0.000000000000000000 ) ) ;
#15110=( BOUNDED_SURFACE ( )  B_SPLINE_SURFACE ( 3, 2, ( 
 ( #17653, #14430, #21439 ),
 ( #21324, #5742, #4042 ),
 ( #10648, #21215, #14200 ),
 ( #5965, #5861, #19497 ),
 ( #11010, #12936, #19947 ),
 ( #2301, #1963, #3802 ) ),
 .UNSPECIFIED., .F., .F., .F. ) 
 B_SPLINE_SURFACE_WITH_KNOTS ( ( 4, 2, 4 ),
 ( 3, 3 ),
 ( 0.000000000000000000, 0.002858401832365848987, 0.005716803664731697973 ),
 ( 0.000000000000000000, 1.000000000000000000 ),
 .UNSPECIFIED. ) 
 GEOMETRIC_REPRESENTATION_ITEM ( )  RATIONAL_B_SPLINE_SURFACE ( (
 ( 1.000000000000000000, 0.7200096751079149149, 1.000000000000000000),
 ( 1.000000000000000000, 0.7065285139740180576, 1.000000000000000000),
 ( 1.000000000000000000, 0.6920701670995640375, 1.000000000000000000),
 ( 1.000000000000000000, 0.6615687397052482099, 1.000000000000000000),
 ( 1.000000000000000000, 0.6455195629506302879, 1.000000000000000000),
 ( 1.000000000000000000, 0.6290213284793395587, 1.000000000000000000) ) ) 
 REPRESENTATION_ITEM ( '' )  SURFACE ( )  );
#15113=CIRCLE ( 'NONE', #5265, 2.499999999999998668 ) ;
#15114=EDGE_LOOP ( 'NONE', ( #21993, #2235 ) ) ;
#15115=AXIS2_PLACEMENT_3D ( 'NONE', #436, #14520, #21301 ) ;
#15118=CARTESIAN_POINT ( 'NONE',  ( 11.06593724743305529, 40.00000000000000000, 53.99256019164672438 ) ) ;
#15121=LINE ( 'NONE', #19484, #1753 ) ;
#15122=CARTESIAN_POINT ( 'NONE',  ( 2.601474714586665016, 5.225049111783174105, -39.07471001004994093 ) ) ;
#15123=EDGE_LOOP ( 'NONE', ( #11929, #5216 ) ) ;
#15124=CARTESIAN_POINT ( 'NONE',  ( -42.50000000000000711, -12.00000000000000000, -47.50000000000000000 ) ) ;
#15129=DIRECTION ( 'NONE',  ( 0.000000000000000000, 0.000000000000000000, -1.000000000000000000 ) ) ;
#15131=CARTESIAN_POINT ( 'NONE',  ( 9.952189117650823036, 40.00000000000000000, 53.64426396172073197 ) ) ;
#15133=CARTESIAN_POINT ( 'NONE',  ( -5.651049805244181101, 39.99999999999999289, -51.93203809155826889 ) ) ;
#15134=ORIENTED_EDGE ( 'NONE', *, *, #11384, .F. ) ;
#15137=ORIENTED_EDGE ( 'NONE', *, *, #6352, .T. ) ;
#15139=AXIS2_PLACEMENT_3D ( 'NONE', #1239, #1358, #15428 ) ;
#15142=VECTOR ( 'NONE', #11903, 1000.000000000000000 ) ;
#15143=CARTESIAN_POINT ( 'NONE',  ( 22.20813536596259041, 23.24072130216428178, -58.62062866457824128 ) ) ;
#15145=EDGE_LOOP ( 'NONE', ( #19208, #22538 ) ) ;
#15147=VERTEX_POINT ( 'NONE', #16101 ) ;
#15150=AXIS2_PLACEMENT_3D ( 'NONE', #18083, #9391, #16365 ) ;
#15152=ADVANCED_FACE ( 'NONE', ( #17488 ), #5353, .F. ) ;
#15160=DIRECTION ( 'NONE',  ( -1.000000000000000000, 0.000000000000000000, 0.000000000000000000 ) ) ;
#15164=CARTESIAN_POINT ( 'NONE',  ( -0.09368727804205789766, 39.99996055794411376, 48.80679978730719881 ) ) ;
#15165=AXIS2_PLACEMENT_3D ( 'NONE', #8497, #15471, #15129 ) ;
#15169=CIRCLE ( 'NONE', #20682, 22.00000000000000000 ) ;
#15171=CARTESIAN_POINT ( 'NONE',  ( -18.34034842040193425, 28.02508533843026939, 60.20240101110111652 ) ) ;
#15175=CARTESIAN_POINT ( 'NONE',  ( -15.34286839272958147, 7.164559734098759236, -59.29291272740923091 ) ) ;
#15181=CARTESIAN_POINT ( 'NONE',  ( -4.110274091176338018, 39.99999999999999289, -51.15360534159206196 ) ) ;
#15185=LINE ( 'NONE', #6728, #22547 ) ;
#15187=CARTESIAN_POINT ( 'NONE',  ( -10.35284963923112933, 39.23826485901322769, 54.78050591838192673 ) ) ;
#15188=CARTESIAN_POINT ( 'NONE',  ( 15.03694978697417994, 3.237610724645296312, 56.60357944353837922 ) ) ;
#15189=CIRCLE ( 'NONE', #15551, 14.00000000000000000 ) ;
#15190=ADVANCED_FACE ( 'NONE', ( #5682 ), #16312, .F. ) ;
#15193=AXIS2_PLACEMENT_3D ( 'NONE', #21968, #4090, #9806 ) ;
#15195=CARTESIAN_POINT ( 'NONE',  ( -35.00000000000000000, 2.142135623730931471, 1.387778780781445676E-14 ) ) ;
#15196=DIRECTION ( 'NONE',  ( 0.000000000000000000, 0.000000000000000000, 1.000000000000000000 ) ) ;
#15197=ADVANCED_FACE ( 'NONE', ( #524 ), #4986, .F. ) ;
#15198=AXIS2_PLACEMENT_3D ( 'NONE', #1722, #7325, #8706 ) ;
#15199=B_SPLINE_CURVE_WITH_KNOTS ( 'NONE', 3,
 ( #9591, #9490, #9373, #6166, #2618, #22092, #11076, #16470, #7654, #18409 ),
 .UNSPECIFIED., .F., .F.,
 ( 4, 2, 2, 2, 4 ),
 ( 0.000000000000000000, 0.0006732693119717972395, 0.001346538623943594479, 0.002019807935915391827, 0.002693077247887188958 ),
 .UNSPECIFIED. ) ;
#15200=ORIENTED_EDGE ( 'NONE', *, *, #1802, .T. ) ;
#15201=CONICAL_SURFACE ( 'NONE', #17025, 2.525000000000110489, 0.7853981633971014453 ) ;
#15202=EDGE_LOOP ( 'NONE', ( #5872, #2854, #737, #5784 ) ) ;
#15203=CARTESIAN_POINT ( 'NONE',  ( 0.1895185485179805007, -3.154272558796861858, 47.17695316422283014 ) ) ;
#15205=VECTOR ( 'NONE', #20705, 1000.000000000000000 ) ;
#15212=DIRECTION ( 'NONE',  ( -1.000000000000000000, 0.000000000000000000, 0.000000000000000000 ) ) ;
#15213=CARTESIAN_POINT ( 'NONE',  ( -20.11656324090263936, 10.00164725896635076, -58.12608834080167952 ) ) ;
#15214=DIRECTION ( 'NONE',  ( -0.000000000000000000, -1.000000000000000000, -0.000000000000000000 ) ) ;
#15215=AXIS2_PLACEMENT_3D ( 'NONE', #10742, #17747, #9043 ) ;
#15216=DIRECTION ( 'NONE',  ( 0.000000000000000000, 0.000000000000000000, -1.000000000000000000 ) ) ;
#15218=CARTESIAN_POINT ( 'NONE',  ( 9.855264211176363531, 31.32970427768387722, 43.22210574525158933 ) ) ;
#15223=ORIENTED_EDGE ( 'NONE', *, *, #22619, .T. ) ;
#15226=CARTESIAN_POINT ( 'NONE',  ( 5.833333333333339255, 6.180730040185842711, 40.61164310337068173 ) ) ;
#15229=ORIENTED_EDGE ( 'NONE', *, *, #17462, .F. ) ;
#15231=VERTEX_POINT ( 'NONE', #14610 ) ;
#15233=DIRECTION ( 'NONE',  ( -0.000000000000000000, 1.000000000000000000, -0.000000000000000000 ) ) ;
#15237=DIRECTION ( 'NONE',  ( -1.000000000000000000, 0.000000000000000000, 0.000000000000000000 ) ) ;
#15241=DIRECTION ( 'NONE',  ( 0.000000000000000000, 0.000000000000000000, 1.000000000000000000 ) ) ;
#15242=ORIENTED_EDGE ( 'NONE', *, *, #7371, .F. ) ;
#15243=CARTESIAN_POINT ( 'NONE',  ( -15.00000000000001599, 19.61444766276327556, -45.82575694955838230 ) ) ;
#15248=CARTESIAN_POINT ( 'NONE',  ( 6.913287910056896912, 40.00000000000000711, 52.51234321215227396 ) ) ;
#15249=VERTEX_POINT ( 'NONE', #21726 ) ;
#15253=CARTESIAN_POINT ( 'NONE',  ( -19.51193873661508960, 31.10741194645162366, 57.96703944061304270 ) ) ;
#15255=DIRECTION ( 'NONE',  ( 0.000000000000000000, 1.000000000000000000, 0.000000000000000000 ) ) ;
#15257=CARTESIAN_POINT ( 'NONE',  ( 34.99999999999980815, 26.00000000000000355, 54.99999999999922551 ) ) ;
#15258=B_SPLINE_CURVE_WITH_KNOTS ( 'NONE', 3,
 ( #9802, #8419, #1097, #6358, #1198, #15389 ),
 .UNSPECIFIED., .F., .F.,
 ( 4, 2, 4 ),
 ( 1.939479807224432123E-18, 0.002694896630593770787, 0.005389793261187539840 ),
 .UNSPECIFIED. ) ;
#15259=TOROIDAL_SURFACE ( 'NONE', #5389, 50.00000000000000000, 10.00000000000000000 ) ;
#15260=CARTESIAN_POINT ( 'NONE',  ( 18.14868794606629265, 11.58103667096281875, -57.62894917896122138 ) ) ;
#15268=ORIENTED_EDGE ( 'NONE', *, *, #7467, .T. ) ;
#15272=AXIS2_PLACEMENT_3D ( 'NONE', #19512, #9426, #14217 ) ;
#15276=ORIENTED_EDGE ( 'NONE', *, *, #11635, .F. ) ;
#15278=AXIS2_PLACEMENT_3D ( 'NONE', #12587, #16382, #12819 ) ;
#15280=DIRECTION ( 'NONE',  ( -0.000000000000000000, 1.000000000000000000, -0.000000000000000000 ) ) ;
#15285=CARTESIAN_POINT ( 'NONE',  ( -8.759110511859015347, 7.803016162472652617, 42.56552456877081170 ) ) ;
#15286=ADVANCED_FACE ( 'NONE', ( #2597 ), #12880, .T. ) ;
#15292=ORIENTED_EDGE ( 'NONE', *, *, #2035, .T. ) ;
#15296=CARTESIAN_POINT ( 'NONE',  ( -18.97285531159713301, 26.38757670764340446, 60.36948798341369127 ) ) ;
#15298=B_SPLINE_SURFACE_WITH_KNOTS ( 'NONE', 1, 3, ( 
 ( #16876, #9657, #16646, #18479, #951, #13413, #7947, #1074, #15133, #8279, #8063, #22038, #4747, #1287, #11716, #18712, #3017, #19278, #17546, #5402 ),
 ( #15706, #8394, #8500, #12056, #17427, #12383, #6907, #1856, #22494, #10542, #1746, #7115, #13868, #20887, #22384, #15366, #15810, #6673, #19163, #1628 ) ),
 .UNSPECIFIED., .F., .F., .F.,
 ( 2, 2 ),
 ( 4, 2, 2, 2, 2, 2, 2, 2, 2, 4 ),
 ( 0.000000000000000000, 1.000000000000000000 ),
 ( 0.000000000000000000, 0.002777081680065593070, 0.004165622520098389604, 0.005554163360131186139, 0.006942704200163982674, 0.008331245040196779209, 0.009025515460213177910, 0.009719785880229574876, 0.01041405630024597358, 0.01110832672026237228 ),
 .UNSPECIFIED. ) ;
#15300=CARTESIAN_POINT ( 'NONE',  ( 6.692425168897880638, 39.70962082636729917, 53.18141012597577344 ) ) ;
#15302=AXIS2_PLACEMENT_3D ( 'NONE', #1458, #8331, #15304 ) ;
#15304=DIRECTION ( 'NONE',  ( 0.000000000000000000, 0.000000000000000000, 1.000000000000000000 ) ) ;
#15305=CARTESIAN_POINT ( 'NONE',  ( -6.286720893520962861, 40.00000000000000711, -52.22859683420058730 ) ) ;
#15309=DIRECTION ( 'NONE',  ( 0.000000000000000000, -0.7071067811867928210, -0.7071067811863022134 ) ) ;
#15312=CARTESIAN_POINT ( 'NONE',  ( -35.00000000000058265, 28.00000000000000000, -52.90000000000076597 ) ) ;
#15313=EDGE_CURVE ( 'NONE', #22096, #18746, #2771, .T. ) ;
#15314=CARTESIAN_POINT ( 'NONE',  ( 7.776554266669417956E-15, -4.648749848372173865, -45.43309249825056639 ) ) ;
#15315=FACE_BOUND ( 'NONE', #8957, .T. ) ;
#15319=EDGE_CURVE ( 'NONE', #3734, #4131, #10818, .T. ) ;
#15320=ORIENTED_EDGE ( 'NONE', *, *, #10957, .T. ) ;
#15321=CARTESIAN_POINT ( 'NONE',  ( -7.688876120686208182, -2.941163814652081321, 52.37456181060783678 ) ) ;
#15323=ORIENTED_EDGE ( 'NONE', *, *, #3552, .T. ) ;
#15326=DIRECTION ( 'NONE',  ( -0.000000000000000000, -0.000000000000000000, 1.000000000000000000 ) ) ;
#15327=CARTESIAN_POINT ( 'NONE',  ( 35.00000000000058265, 40.00000000000000000, -57.10000000000076170 ) ) ;
#15328=CARTESIAN_POINT ( 'NONE',  ( -17.96644252022830912, 11.16803817567492807, -57.57522208103581818 ) ) ;
#15329=B_SPLINE_CURVE_WITH_KNOTS ( 'NONE', 3,
 ( #21187, #21299, #5589, #19580, #786, #16122, #19919, #21639, #434, #4009, #6173, #16241, #9258, #7545, #18416, #20038, #5936, #551 ),
 .UNSPECIFIED., .F., .F.,
 ( 4, 2, 2, 2, 2, 2, 2, 2, 4 ),
 ( 0.000000000000000000, 0.001465012583164687458, 0.002930025166329374917, 0.004395037749494062375, 0.005860050332658749833, 0.008790075498988123015, 0.01025508808215280787, 0.01098759437373514510, 0.01172010066531747885 ),
 .UNSPECIFIED. ) ;
#15330=CARTESIAN_POINT ( 'NONE',  ( -7.033428926742907983, 33.31269054942710284, -41.47353357286036157 ) ) ;
#15331=EDGE_CURVE ( 'NONE', #5289, #938, #8259, .T. ) ;
#15332=CARTESIAN_POINT ( 'NONE',  ( -11.88509939556638351, 36.18356491088834304, 55.39957109942756119 ) ) ;
#15335=CARTESIAN_POINT ( 'NONE',  ( 42.50000000000000711, -12.00000000000000000, 47.50000000000000711 ) ) ;
#15336=FACE_BOUND ( 'NONE', #20875, .T. ) ;
#15337=FACE_OUTER_BOUND ( 'NONE', #5433, .T. ) ;
#15338=DIRECTION ( 'NONE',  ( -0.000000000000000000, -1.000000000000000000, -0.000000000000000000 ) ) ;
#15339=ORIENTED_EDGE ( 'NONE', *, *, #21626, .T. ) ;
#15340=EDGE_CURVE ( 'NONE', #20510, #14603, #6365, .T. ) ;
#15341=DIRECTION ( 'NONE',  ( 0.000000000000000000, 0.000000000000000000, -1.000000000000000000 ) ) ;
#15342=CARTESIAN_POINT ( 'NONE',  ( 4.106440533746705590, 5.536968433055398542, 39.55567250430844695 ) ) ;
#15345=AXIS2_PLACEMENT_3D ( 'NONE', #9474, #9233, #16456 ) ;
#15346=ORIENTED_EDGE ( 'NONE', *, *, #9129, .F. ) ;
#15348=EDGE_CURVE ( 'NONE', #13123, #3413, #18505, .T. ) ;
#15349=ORIENTED_EDGE ( 'NONE', *, *, #504, .F. ) ;
#15351=CARTESIAN_POINT ( 'NONE',  ( -0.1963897509097776439, -3.154216256273198571, 47.17168727994772581 ) ) ;
#15354=CARTESIAN_POINT ( 'NONE',  ( 17.38288706075490353, 10.07729229769341828, 59.93358289200956790 ) ) ;
#15359=ORIENTED_EDGE ( 'NONE', *, *, #145, .T. ) ;
#15360=DIRECTION ( 'NONE',  ( -0.000000000000000000, -0.000000000000000000, 1.000000000000000000 ) ) ;
#15366=CARTESIAN_POINT ( 'NONE',  ( -8.555717074797012600, 39.50215801696872830, -54.09939910646557593 ) ) ;
#15374=CARTESIAN_POINT ( 'NONE',  ( -1.387778780781445676E-14, 20.00000000000000000, 98.00000000000000000 ) ) ;
#15375=CARTESIAN_POINT ( 'NONE',  ( 17.76087593031624579, 33.76750075041049826, -57.47290953699885563 ) ) ;
#15376=ORIENTED_EDGE ( 'NONE', *, *, #22339, .T. ) ;
#15380=ADVANCED_FACE ( 'NONE', ( #2711 ), #761, .F. ) ;
#15383=LINE ( 'NONE', #19068, #5606 ) ;
#15384=DIRECTION ( 'NONE',  ( 0.000000000000000000, 0.000000000000000000, -1.000000000000000000 ) ) ;
#15385=VERTEX_POINT ( 'NONE', #3159 ) ;
#15387=FACE_OUTER_BOUND ( 'NONE', #18375, .T. ) ;
#15389=CARTESIAN_POINT ( 'NONE',  ( 9.103081159015154356, 0.03030367950454006254, 53.87333532811640424 ) ) ;
#15394=CARTESIAN_POINT ( 'NONE',  ( -1.328644774245273830, 39.98974582701344360, 49.74044376501583997 ) ) ;
#15397=EDGE_CURVE ( 'NONE', #18218, #15664, #13718, .T. ) ;
#15402=ORIENTED_EDGE ( 'NONE', *, *, #469, .T. ) ;
#15403=ORIENTED_EDGE ( 'NONE', *, *, #4272, .T. ) ;
#15405=CARTESIAN_POINT ( 'NONE',  ( -13.56354382738803288, 2.142135623730931471, 56.03997097393687454 ) ) ;
#15406=CARTESIAN_POINT ( 'NONE',  ( -13.00000000000011546, 42.51666049839536043, 60.00099999999999767 ) ) ;
#15408=CARTESIAN_POINT ( 'NONE',  ( 6.877234547883836591, 39.69228528355510832, 53.28061374633059444 ) ) ;
#15412=DIRECTION ( 'NONE',  ( 0.000000000000000000, 0.000000000000000000, 1.000000000000000000 ) ) ;
#15417=ORIENTED_EDGE ( 'NONE', *, *, #171, .T. ) ;
#15419=EDGE_CURVE ( 'NONE', #20378, #4759, #6997, .T. ) ;
#15422=CYLINDRICAL_SURFACE ( 'NONE', #9691, 2.099999999999997868 ) ;
#15428=DIRECTION ( 'NONE',  ( 0.000000000000000000, 0.000000000000000000, 1.000000000000000000 ) ) ;
#15429=CIRCLE ( 'NONE', #19845, 6.499999999999999112 ) ;
#15432=CARTESIAN_POINT ( 'NONE',  ( 13.76792553423402232, 13.99810558461763321, 45.26963775109940258 ) ) ;
#15436=CARTESIAN_POINT ( 'NONE',  ( -22.35494499951317948, 21.77768233190463576, -58.65240855008566712 ) ) ;
#15437=CARTESIAN_POINT ( 'NONE',  ( -2.636016739579310375, 39.95887900714455299, 50.67500335283390456 ) ) ;
#15438=CARTESIAN_POINT ( 'NONE',  ( -11.59291124596518863, 39.24500985576617040, 55.27372209264447633 ) ) ;
#15440=CARTESIAN_POINT ( 'NONE',  ( 10.38220159744132864, 30.85082733156616186, 43.52345836121337186 ) ) ;
#15445=DIRECTION ( 'NONE',  ( 1.000000000000000000, 0.000000000000000000, 0.000000000000000000 ) ) ;
#15451=ADVANCED_FACE ( 'NONE', ( #8310 ), #7906, .T. ) ;
#15456=CARTESIAN_POINT ( 'NONE',  ( 42.50000000000000711, -5.000000000000000000, -47.50000000000000000 ) ) ;
#15458=CARTESIAN_POINT ( 'NONE',  ( -35.00000000000000000, 0.000000000000000000, 1.387778780781445676E-14 ) ) ;
#15464=CARTESIAN_POINT ( 'NONE',  ( 6.696867368503558448E-15, 40.00000000000000000, 39.73397172404483513 ) ) ;
#15465=VECTOR ( 'NONE', #5588, 1000.000000000000000 ) ;
#15467=EDGE_LOOP ( 'NONE', ( #4865, #16711 ) ) ;
#15468=CARTESIAN_POINT ( 'NONE',  ( 9.377138775076085508, -4.928932188134512948, -51.00555535510811467 ) ) ;
#15469=VECTOR ( 'NONE', #19743, 1000.000000000000000 ) ;
#15470=CARTESIAN_POINT ( 'NONE',  ( 9.103081159019511759, 0.03030367950604059835, -53.87333532811884851 ) ) ;
#15471=DIRECTION ( 'NONE',  ( -0.000000000000000000, -1.000000000000000000, -0.000000000000000000 ) ) ;
#15472=CARTESIAN_POINT ( 'NONE',  ( 7.262748859126449297, 39.65386577974343396, 53.48190593274512139 ) ) ;
#15478=LINE ( 'NONE', #19054, #21391 ) ;
#15479=ORIENTED_EDGE ( 'NONE', *, *, #17683, .F. ) ;
#15480=CARTESIAN_POINT ( 'NONE',  ( 12.99999999999993960, 42.51666049839543149, -105.0010000000000048 ) ) ;
#15481=CARTESIAN_POINT ( 'NONE',  ( -10.27431133777641215, -4.928932188134511172, -51.43682631505697600 ) ) ;
#15484=CIRCLE ( 'NONE', #18056, 2.000000000000001776 ) ;
#15485=DIRECTION ( 'NONE',  ( 0.000000000000000000, 0.000000000000000000, 1.000000000000000000 ) ) ;
#15487=AXIS2_PLACEMENT_3D ( 'NONE', #6878, #6761, #13499 ) ;
#15491=DIRECTION ( 'NONE',  ( 0.000000000000000000, 0.000000000000000000, 1.000000000000000000 ) ) ;
#15494=CARTESIAN_POINT ( 'NONE',  ( 22.29010897948492698, 17.41268129326155645, 58.63841251601399307 ) ) ;
#15496=CARTESIAN_POINT ( 'NONE',  ( 7.549845394205005000, 39.99999999999999289, -52.78128352898642106 ) ) ;
#15499=DIRECTION ( 'NONE',  ( 1.000000000000000000, 0.000000000000000000, 0.000000000000000000 ) ) ;
#15500=VERTEX_POINT ( 'NONE', #4992 ) ;
#15503=ORIENTED_EDGE ( 'NONE', *, *, #13136, .F. ) ;
#15507=CARTESIAN_POINT ( 'NONE',  ( -9.177444842293963845, 39.41890427424159782, 54.36989715539939283 ) ) ;
#15518=CARTESIAN_POINT ( 'NONE',  ( 42.50000000000000711, -12.00000000000000000, 41.00000000000000711 ) ) ;
#15520=CARTESIAN_POINT ( 'NONE',  ( -9.952189117650851458, 40.00000000000000000, -53.64426396172072486 ) ) ;
#15522=CARTESIAN_POINT ( 'NONE',  ( 6.646840102370911829, 39.71385755071619172, 53.15684333213135204 ) ) ;
#15525=DIRECTION ( 'NONE',  ( 0.000000000000000000, 0.000000000000000000, -1.000000000000000000 ) ) ;
#15526=CARTESIAN_POINT ( 'NONE',  ( -7.325661951454969234, 39.99999999999998579, -52.68655285130741106 ) ) ;
#15527=DIRECTION ( 'NONE',  ( -1.000000000000000000, 0.000000000000000000, 0.000000000000000000 ) ) ;
#15528=DIRECTION ( 'NONE',  ( 0.000000000000000000, 0.000000000000000000, 1.000000000000000000 ) ) ;
#15531=EDGE_LOOP ( 'NONE', ( #874, #15603, #3167, #16419 ) ) ;
#15533=CARTESIAN_POINT ( 'NONE',  ( -16.16773315356748242, 31.81208924699231844, 59.56501305110273137 ) ) ;
#15538=CARTESIAN_POINT ( 'NONE',  ( -4.106440533746694932, 34.46303156694462189, 39.55567250430844695 ) ) ;
#15541=AXIS2_PLACEMENT_3D ( 'NONE', #20508, #4815, #11682 ) ;
#15542=ORIENTED_EDGE ( 'NONE', *, *, #20954, .T. ) ;
#15544=CARTESIAN_POINT ( 'NONE',  ( 6.661198439245855418, -4.819795714534470754, -49.67388352366880611 ) ) ;
#15545=DIRECTION ( 'NONE',  ( 1.000000000000000000, 0.000000000000000000, 0.000000000000000000 ) ) ;
#15547=ADVANCED_FACE ( 'NONE', ( #8869 ), #18883, .T. ) ;
#15548=CARTESIAN_POINT ( 'NONE',  ( 29.99999999999998579, 20.00000000000000711, 105.0000000000000142 ) ) ;
#15549=FACE_OUTER_BOUND ( 'NONE', #21542, .T. ) ;
#15551=AXIS2_PLACEMENT_3D ( 'NONE', #2768, #20299, #6309 ) ;
#15552=CARTESIAN_POINT ( 'NONE',  ( -19.80330599461106544, 22.93419722094641600, -60.57506235960028107 ) ) ;
#15554=EDGE_CURVE ( 'NONE', #7926, #7389, #15991, .T. ) ;
#15558=PLANE ( 'NONE',  #21760 ) ;
#15560=CARTESIAN_POINT ( 'NONE',  ( 21.99999999999998579, 20.00000000000000000, 98.00000000000000000 ) ) ;
#15562=AXIS2_PLACEMENT_3D ( 'NONE', #2505, #2845, #1122 ) ;
#15563=ORIENTED_EDGE ( 'NONE', *, *, #12250, .T. ) ;
#15565=DIRECTION ( 'NONE',  ( -0.000000000000000000, 1.000000000000000000, -0.000000000000000000 ) ) ;
#15567=ORIENTED_EDGE ( 'NONE', *, *, #21626, .F. ) ;
#15572=EDGE_CURVE ( 'NONE', #3415, #9032, #11197, .T. ) ;
#15580=VERTEX_POINT ( 'NONE', #12413 ) ;
#15585=CARTESIAN_POINT ( 'NONE',  ( 22.42598460344821376, 19.26775710289564714, -58.66769746720326850 ) ) ;
#15586=CARTESIAN_POINT ( 'NONE',  ( -35.00000000000000000, 2.142135623730931471, 1.387778780781445676E-14 ) ) ;
#15588=CARTESIAN_POINT ( 'NONE',  ( 13.59841332577228989, 26.34257281673388107, -45.18857684126743379 ) ) ;
#15589=VERTEX_POINT ( 'NONE', #7269 ) ;
#15590=DIRECTION ( 'NONE',  ( 0.000000000000000000, 0.000000000000000000, 1.000000000000000000 ) ) ;
#15593=CARTESIAN_POINT ( 'NONE',  ( -18.51338123223703747, 7.266791589766472548, 57.69263490290611429 ) ) ;
#15597=CARTESIAN_POINT ( 'NONE',  ( 42.50000000000000711, -12.00000000000012434, 44.97499999999989484 ) ) ;
#15598=VECTOR ( 'NONE', #8798, 1000.000000000000114 ) ;
#15599=CARTESIAN_POINT ( 'NONE',  ( 12.91716037299105757, 4.693711897361043661, -55.81219010903327415 ) ) ;
#15601=ORIENTED_EDGE ( 'NONE', *, *, #13335, .F. ) ;
#15602=VERTEX_POINT ( 'NONE', #50 ) ;
#15603=ORIENTED_EDGE ( 'NONE', *, *, #15916, .T. ) ;
#15604=( LENGTH_UNIT ( ) NAMED_UNIT ( * ) SI_UNIT ( .MILLI., .METRE. ) );
#15605=ADVANCED_FACE ( 'NONE', ( #17684 ), #14481, .F. ) ;
#15610=CARTESIAN_POINT ( 'NONE',  ( 13.67681338760603715, 37.77871559274756663, 56.08437820317178080 ) ) ;
#15611=CARTESIAN_POINT ( 'NONE',  ( 8.845644329309713783, 39.99999999999999289, -53.28398128908064280 ) ) ;
#15612=CARTESIAN_POINT ( 'NONE',  ( 1.387778780781445676E-14, 40.00000000000000000, 48.73397172404482802 ) ) ;
#15615=DIRECTION ( 'NONE',  ( 0.000000000000000000, 0.000000000000000000, 1.000000000000000000 ) ) ;
#15617=ORIENTED_EDGE ( 'NONE', *, *, #16314, .F. ) ;
#15619=ORIENTED_EDGE ( 'NONE', *, *, #18211, .T. ) ;
#15620=CARTESIAN_POINT ( 'NONE',  ( 6.297084008441820480, 38.99689388921666477, -53.73982653936155174 ) ) ;
#15623=CARTESIAN_POINT ( 'NONE',  ( -2.232801763152736818, 39.96997183162479672, 50.39091575928458155 ) ) ;
#15625=CARTESIAN_POINT ( 'NONE',  ( 17.42297160866501571, 10.14068842408646809, 59.94615209474302020 ) ) ;
#15634=ORIENTED_EDGE ( 'NONE', *, *, #5213, .F. ) ;
#15637=AXIS2_PLACEMENT_3D ( 'NONE', #21810, #22377, #20877 ) ;
#15638=B_SPLINE_CURVE_WITH_KNOTS ( 'NONE', 1,
 ( #10419, #8383 ),
 .UNSPECIFIED., .F., .F.,
 ( 2, 2 ),
 ( 0.000000000000000000, 1.000000000000000000 ),
 .UNSPECIFIED. ) ;
#15640=CARTESIAN_POINT ( 'NONE',  ( -11.49398617736659034, 40.00000000000000711, -54.13866599136176205 ) ) ;
#15642=CARTESIAN_POINT ( 'NONE',  ( 6.571663212755819217, 39.72078165691683438, 53.11617168483076057 ) ) ;
#15643=AXIS2_PLACEMENT_3D ( 'NONE', #21980, #19906, #12672 ) ;
#15645=ADVANCED_FACE ( 'NONE', ( #3951 ), #10580, .T. ) ;
#15648=CARTESIAN_POINT ( 'NONE',  ( -7.158017810174624351, 39.99999999999999289, -52.61520711206481593 ) ) ;
#15654=ADVANCED_FACE ( 'NONE', ( #21135 ), #18164, .T. ) ;
#15660=DIRECTION ( 'NONE',  ( 0.000000000000000000, -1.000000000000000000, 0.000000000000000000 ) ) ;
#15662=VERTEX_POINT ( 'NONE', #2223 ) ;
#15664=VERTEX_POINT ( 'NONE', #9661 ) ;
#15667=CARTESIAN_POINT ( 'NONE',  ( 11.28246622563954915, 40.00000000000000000, -54.06713842414182380 ) ) ;
#15670=AXIS2_PLACEMENT_3D ( 'NONE', #2383, #10730, #9374 ) ;
#15674=CARTESIAN_POINT ( 'NONE',  ( -20.00295458799181247, 20.28336436466281612, -60.62247787804551535 ) ) ;
#15675=AXIS2_PLACEMENT_3D ( 'NONE', #18096, #2411, #3372 ) ;
#15676=CARTESIAN_POINT ( 'NONE',  ( 35.00000000000000000, 2.142135623730931471, 4.258610482196280173E-15 ) ) ;
#15678=ORIENTED_EDGE ( 'NONE', *, *, #21210, .T. ) ;
#15679=CARTESIAN_POINT ( 'NONE',  ( 7.325260514639500961E-15, -4.648749848371387827, 45.43309249825157536 ) ) ;
#15680=CARTESIAN_POINT ( 'NONE',  ( 15.49999999999993783, 42.51666049839543149, 60.00099999999999767 ) ) ;
#15682=CARTESIAN_POINT ( 'NONE',  ( -35.00000000000000000, -4.999999999999997335, 1.387778780781445676E-14 ) ) ;
#15686=CARTESIAN_POINT ( 'NONE',  ( 35.00000000000000000, 40.00000000000000000, 4.258610482196280173E-15 ) ) ;
#15690=ORIENTED_EDGE ( 'NONE', *, *, #14720, .T. ) ;
#15693=ORIENTED_EDGE ( 'NONE', *, *, #12082, .F. ) ;
#15695=CARTESIAN_POINT ( 'NONE',  ( 9.103081159019511759, 0.03030367950604065386, -53.87333532811885561 ) ) ;
#15696=DIRECTION ( 'NONE',  ( 0.000000000000000000, 0.000000000000000000, -1.000000000000000000 ) ) ;
#15697=DIRECTION ( 'NONE',  ( -0.000000000000000000, -0.000000000000000000, -1.000000000000000000 ) ) ;
#15700=CARTESIAN_POINT ( 'NONE',  ( -10.95224849132202927, 40.00000000000000711, -53.95427542910578467 ) ) ;
#15702=CARTESIAN_POINT ( 'NONE',  ( -18.00000000000001421, 20.00000000000000355, -102.0000000000000142 ) ) ;
#15703=CARTESIAN_POINT ( 'NONE',  ( 18.35281960068861196, 33.06122318964057172, -57.65236019522514965 ) ) ;
#15704=CARTESIAN_POINT ( 'NONE',  ( -35.00000000000000000, 0.000000000000000000, -8.999999999999989342 ) ) ;
#15705=CARTESIAN_POINT ( 'NONE',  ( 1.485224240694672737, 39.99052334830943778, 49.86416386702911296 ) ) ;
#15706=CARTESIAN_POINT ( 'NONE',  ( -1.387778780781474075E-14, 40.00000000000002132, -48.73397172404482092 ) ) ;
#15713=CARTESIAN_POINT ( 'NONE',  ( 42.50000000000000711, -5.000000000000000000, -47.50000000000000000 ) ) ;
#15716=ORIENTED_EDGE ( 'NONE', *, *, #6147, .T. ) ;
#15722=CARTESIAN_POINT ( 'NONE',  ( 20.67483659015367436, 11.23071942442634885, 58.26617649125748954 ) ) ;
#15725=CARTESIAN_POINT ( 'NONE',  ( 9.233659691198207398, 40.00000000000000000, 53.41795191989319136 ) ) ;
#15730=ORIENTED_EDGE ( 'NONE', *, *, #11936, .F. ) ;
#15731=DIRECTION ( 'NONE',  ( 0.000000000000000000, 0.000000000000000000, 1.000000000000000000 ) ) ;
#15732=DIRECTION ( 'NONE',  ( -0.000000000000000000, 1.000000000000000000, -0.000000000000000000 ) ) ;
#15733=VERTEX_POINT ( 'NONE', #4820 ) ;
#15736=VERTEX_POINT ( 'NONE', #4481 ) ;
#15737=CARTESIAN_POINT ( 'NONE',  ( 2.881564033229496502, 39.80724459714780750, -51.34429167881276612 ) ) ;
#15740=CARTESIAN_POINT ( 'NONE',  ( 20.00295458799178405, 20.28336436466281612, 60.62247787804552956 ) ) ;
#15743=ADVANCED_FACE ( 'NONE', ( #22241 ), #8033, .F. ) ;
#15746=EDGE_LOOP ( 'NONE', ( #12738, #9698 ) ) ;
#15748=VERTEX_POINT ( 'NONE', #18791 ) ;
#15750=CARTESIAN_POINT ( 'NONE',  ( -1.387778780781445676E-14, 20.00000000000000000, 102.0000000000000142 ) ) ;
#15752=EDGE_CURVE ( 'NONE', #16159, #3040, #18518, .T. ) ;
#15754=CARTESIAN_POINT ( 'NONE',  ( -42.50000000000000711, -12.00000000000000000, -54.00000000000000000 ) ) ;
#15755=CARTESIAN_POINT ( 'NONE',  ( 0.02448413884701040183, 39.99999651920320076, 48.75302353242081210 ) ) ;
#15757=CIRCLE ( 'NONE', #16113, 58.99999999999994316 ) ;
#15759=ORIENTED_EDGE ( 'NONE', *, *, #10401, .T. ) ;
#15760=DIRECTION ( 'NONE',  ( 0.000000000000000000, 0.000000000000000000, 1.000000000000000000 ) ) ;
#15761=DIRECTION ( 'NONE',  ( -0.000000000000000000, 1.000000000000000000, -0.000000000000000000 ) ) ;
#15762=LINE ( 'NONE', #70, #22280 ) ;
#15765=CIRCLE ( 'NONE', #19088, 2.525000000000110489 ) ;
#15766=CARTESIAN_POINT ( 'NONE',  ( -9.786577258570266835, 39.51695195164889896, 54.52237260331529001 ) ) ;
#15768=DIRECTION ( 'NONE',  ( -1.000000000000000000, 0.000000000000000000, 0.000000000000000000 ) ) ;
#15776=AXIS2_PLACEMENT_3D ( 'NONE', #14099, #9310, #7587 ) ;
#15780=CARTESIAN_POINT ( 'NONE',  ( -16.16619463698821946, 31.79081685853821782, -57.00191113791401420 ) ) ;
#15782=ORIENTED_EDGE ( 'NONE', *, *, #13219, .F. ) ;
#15783=CARTESIAN_POINT ( 'NONE',  ( 9.103081159019511759, 0.03030367950604059835, -53.87333532811884851 ) ) ;
#15784=FACE_OUTER_BOUND ( 'NONE', #10288, .T. ) ;
#15785=FACE_OUTER_BOUND ( 'NONE', #20364, .T. ) ;
#15786=CARTESIAN_POINT ( 'NONE',  ( 13.25963002225075194, 12.97669314386527439, -45.02656532858657101 ) ) ;
#15791=CIRCLE ( 'NONE', #14331, 2.099999999999990763 ) ;
#15793=ADVANCED_FACE ( 'NONE', ( #15337 ), #339, .F. ) ;
#15794=ORIENTED_EDGE ( 'NONE', *, *, #7647, .F. ) ;
#15796=CARTESIAN_POINT ( 'NONE',  ( 1.522021317816235619, -4.618502324873039022, 46.61386490714507147 ) ) ;
#15799=CARTESIAN_POINT ( 'NONE',  ( 35.00000000000000711, 2.142135623730931471, 60.00000000000000711 ) ) ;
#15800=VERTEX_POINT ( 'NONE', #18684 ) ;
#15802=DIRECTION ( 'NONE',  ( -0.000000000000000000, 1.000000000000000000, -0.000000000000000000 ) ) ;
#15806=DIRECTION ( 'NONE',  ( -0.000000000000000000, -1.000000000000000000, -0.000000000000000000 ) ) ;
#15807=AXIS2_PLACEMENT_3D ( 'NONE', #14046, #2159, #16233 ) ;
#15808=CIRCLE ( 'NONE', #18754, 57.00000000000002132 ) ;
#15809=DIRECTION ( 'NONE',  ( -1.000000000000000000, 0.000000000000000000, 0.000000000000000000 ) ) ;
#15810=CARTESIAN_POINT ( 'NONE',  ( -8.776846322808903977, 39.47243301020848349, -54.19537465121766928 ) ) ;
#15813=CARTESIAN_POINT ( 'NONE',  ( -3.655629734721801416, 39.91824796244861773, -51.36063886735895068 ) ) ;
#15820=VERTEX_POINT ( 'NONE', #20406 ) ;
#15822=AXIS2_PLACEMENT_3D ( 'NONE', #10806, #21478, #12757 ) ;
#15824=DIRECTION ( 'NONE',  ( -0.000000000000000000, 1.000000000000000000, -0.000000000000000000 ) ) ;
#15827=CARTESIAN_POINT ( 'NONE',  ( 2.783900019938605919, 39.99999999999999289, 50.42898711214131424 ) ) ;
#15829=FACE_BOUND ( 'NONE', #2929, .T. ) ;
#15830=DIRECTION ( 'NONE',  ( 0.000000000000000000, -1.000000000000000000, 0.000000000000000000 ) ) ;
#15831=VERTEX_POINT ( 'NONE', #10518 ) ;
#15832=ADVANCED_FACE ( 'NONE', ( #1834 ), #17522, .F. ) ;
#15833=CARTESIAN_POINT ( 'NONE',  ( -16.62266455332489201, 35.11598757108757241, -57.12012504743137953 ) ) ;
#15835=ORIENTED_EDGE ( 'NONE', *, *, #10402, .T. ) ;
#15837=EDGE_LOOP ( 'NONE', ( #5250, #4862 ) ) ;
#15839=CARTESIAN_POINT ( 'NONE',  ( -2.669020651088310103, 39.95797167561620711, 50.69824585152028362 ) ) ;
#15842=CARTESIAN_POINT ( 'NONE',  ( 19.39432138270210260, 15.03492235294207546, 60.47577240662250375 ) ) ;
#15843=DIRECTION ( 'NONE',  ( 8.659560562351929024E-17, -0.7071067811867928210, 0.7071067811863022134 ) ) ;
#15844=CIRCLE ( 'NONE', #3793, 2.099999999999997868 ) ;
#15846=CARTESIAN_POINT ( 'NONE',  ( 10.49999999999994316, 42.51666049839543149, -100.0000000000000000 ) ) ;
#15847=VERTEX_POINT ( 'NONE', #17282 ) ;
#15850=ADVANCED_FACE ( 'NONE', ( #5050, #19471, #12030, #19369, #1597, #8585, #3336, #15785 ), #6877, .T. ) ;
#15852=ORIENTED_EDGE ( 'NONE', *, *, #9867, .F. ) ;
#15856=VECTOR ( 'NONE', #897, 1000.000000000000000 ) ;
#15858=CARTESIAN_POINT ( 'NONE',  ( 0.1974762773663032156, 39.99977543037353911, 48.88709678338103259 ) ) ;
#15859=EDGE_CURVE ( 'NONE', #18194, #17863, #22193, .T. ) ;
#15860=EDGE_CURVE ( 'NONE', #13273, #8612, #10834, .T. ) ;
#15861=AXIS2_PLACEMENT_3D ( 'NONE', #5055, #6764, #17528 ) ;
#15862=ORIENTED_EDGE ( 'NONE', *, *, #6122, .T. ) ;
#15864=DIRECTION ( 'NONE',  ( -0.000000000000000000, -0.000000000000000000, 1.000000000000000000 ) ) ;
#15865=DIRECTION ( 'NONE',  ( 0.000000000000000000, 0.000000000000000000, 1.000000000000000000 ) ) ;
#15866=LINE ( 'NONE', #9230, #8250 ) ;
#15867=( NAMED_UNIT ( * ) SI_UNIT ( $, .STERADIAN. ) SOLID_ANGLE_UNIT ( ) );
#15869=DIRECTION ( 'NONE',  ( -0.000000000000000000, -1.000000000000000000, -0.000000000000000000 ) ) ;
#15875=VERTEX_POINT ( 'NONE', #17400 ) ;
#15879=CARTESIAN_POINT ( 'NONE',  ( 9.327259721472362486, -2.742977016014242597, -53.40697688051515968 ) ) ;
#15880=AXIS2_PLACEMENT_3D ( 'NONE', #6568, #22153, #6450 ) ;
#15881=CARTESIAN_POINT ( 'NONE',  ( 9.952189117650862116, 40.00000000000000000, -53.64426396172072486 ) ) ;
#15883=EDGE_CURVE ( 'NONE', #6097, #7816, #3536, .T. ) ;
#15887=CARTESIAN_POINT ( 'NONE',  ( 35.00000000000000711, -4.928932188134504955, -57.07106781186551103 ) ) ;
#15893=PLANE ( 'NONE',  #16209 ) ;
#15897=AXIS2_PLACEMENT_3D ( 'NONE', #2851, #2965, #1666 ) ;
#15898=CARTESIAN_POINT ( 'NONE',  ( -26.00000000000001421, 19.99999999999982947, -100.0000000000000000 ) ) ;
#15902=CIRCLE ( 'NONE', #21802, 51.00000000000001421 ) ;
#15907=VECTOR ( 'NONE', #15095, 1000.000000000000000 ) ;
#15909=B_SPLINE_CURVE_WITH_KNOTS ( 'NONE', 3,
 ( #16866, #4390, #11480, #3006, #14897, #1164, #16753, #4278, #18349, #15122, #13402, #20426, #16637, #9763, #22028, #8051 ),
 .UNSPECIFIED., .F., .F.,
 ( 4, 2, 2, 2, 2, 2, 2, 4 ),
 ( 8.673617379884034509E-19, 0.003169695113379726766, 0.006339390226759453531, 0.007924237783449316480, 0.008716661561794248822, 0.009509085340139179429, 0.01109393289682905105, 0.01267878045351892267 ),
 .UNSPECIFIED. ) ;
#15913=CARTESIAN_POINT ( 'NONE',  ( -11.68090480754633553, 3.765577839755393619, -57.90797000640142045 ) ) ;
#15914=ORIENTED_EDGE ( 'NONE', *, *, #364, .T. ) ;
#15916=EDGE_CURVE ( 'NONE', #12233, #8676, #1719, .T. ) ;
#15918=VECTOR ( 'NONE', #12328, 1000.000000000000000 ) ;
#15919=LINE ( 'NONE', #22611, #18110 ) ;
#15920=EDGE_CURVE ( 'NONE', #19146, #12705, #15954, .T. ) ;
#15924=CARTESIAN_POINT ( 'NONE',  ( -12.24744603029287937, 40.00000000000000000, -54.43639671998464991 ) ) ;
#15926=EDGE_LOOP ( 'NONE', ( #15634, #1772 ) ) ;
#15930=CARTESIAN_POINT ( 'NONE',  ( 9.952189117650862116, 40.00000000000000000, -53.64426396172072486 ) ) ;
#15934=EDGE_LOOP ( 'NONE', ( #1544, #10046, #15346, #3931 ) ) ;
#15935=CIRCLE ( 'NONE', #6078, 2.500000000000002220 ) ;
#15939=ORIENTED_EDGE ( 'NONE', *, *, #7889, .F. ) ;
#15940=CARTESIAN_POINT ( 'NONE',  ( 42.50000000000000711, -9.600000000000001421, -47.50000000000000000 ) ) ;
#15941=CARTESIAN_POINT ( 'NONE',  ( -1.387778780781445676E-14, 20.00000000000000000, 60.00200000000000244 ) ) ;
#15942=EDGE_CURVE ( 'NONE', #8817, #18120, #12244, .T. ) ;
#15943=CARTESIAN_POINT ( 'NONE',  ( 0.7361814224980237631, 39.99998183296705179, -49.30708964234285219 ) ) ;
#15944=CARTESIAN_POINT ( 'NONE',  ( 9.272092376743565012, 39.99999999999999289, 53.43088570351475397 ) ) ;
#15951=CARTESIAN_POINT ( 'NONE',  ( 0.2891450487059649133, -0.01224742503970683433, 48.63032622729384258 ) ) ;
#15953=CARTESIAN_POINT ( 'NONE',  ( 6.102098042870833506E-15, -2.522175986002989312, 47.48283745780745591 ) ) ;
#15954=CIRCLE ( 'NONE', #21088, 2.099999999999997868 ) ;
#15959=CARTESIAN_POINT ( 'NONE',  ( -7.538461658765283957, 38.52939893239184954, 55.92178727523601367 ) ) ;
#15962=CARTESIAN_POINT ( 'NONE',  ( 8.687723243037263288, 39.99999999999999289, -53.22563606164203520 ) ) ;
#15963=CARTESIAN_POINT ( 'NONE',  ( 22.38794582965086022, 21.29119307984318255, 58.65949541090324715 ) ) ;
#15964=CARTESIAN_POINT ( 'NONE',  ( 90.00000000000000000, 40.00000000000000711, 2.524999999999998579 ) ) ;
#15966=B_SPLINE_CURVE_WITH_KNOTS ( 'NONE', 3,
 ( #22155, #6452, #11938, #18714, #17206, #1520 ),
 .UNSPECIFIED., .F., .F.,
 ( 4, 2, 4 ),
 ( 1.748223473168675632E-18, 0.004604358499702457599, 0.009208716999404913464 ),
 .UNSPECIFIED. ) ;
#15973=FACE_OUTER_BOUND ( 'NONE', #7441, .T. ) ;
#15980=DIRECTION ( 'NONE',  ( -0.000000000000000000, -0.000000000000000000, 1.000000000000000000 ) ) ;
#15981=CARTESIAN_POINT ( 'NONE',  ( 0.8008155648455618225, 39.99628551735307980, 49.34729276519122720 ) ) ;
#15985=CARTESIAN_POINT ( 'NONE',  ( 42.50000000000000711, -12.00000000000012434, -47.50000000000000000 ) ) ;
#15986=FACE_OUTER_BOUND ( 'NONE', #5651, .T. ) ;
#15987=DIRECTION ( 'NONE',  ( 1.000000000000000000, 0.000000000000000000, 0.000000000000000000 ) ) ;
#15988=CIRCLE ( 'NONE', #6127, 2.525000000000110489 ) ;
#15991=B_SPLINE_CURVE_WITH_KNOTS ( 'NONE', 3,
 ( #19311, #19426, #269, #3726, #12192, #10677, #5438, #9103, #386, #1995, #9206, #17460, #14346, #13901, #12513, #15959, #20917, #12308 ),
 .UNSPECIFIED., .F., .F.,
 ( 4, 2, 2, 2, 2, 2, 2, 2, 4 ),
 ( -3.543127106788223826E-05, 0.0006851204654911835761, 0.001405672202050249533, 0.002846775675168380579, 0.005728982621404643538, 0.007170086094522767212, 0.008611189567640890885, 0.01005229304075901629, 0.01149339651387713823 ),
 .UNSPECIFIED. ) ;
#15992=( BOUNDED_SURFACE ( )  B_SPLINE_SURFACE ( 3, 2, ( 
 ( #12930, #2646, #11222 ),
 ( #6412, #16498, #13378 ),
 ( #9618, #21778, #16611 ),
 ( #917, #13716, #8467 ),
 ( #3433, #5043, #12238 ),
 ( #8242, #8359, #11897 ),
 ( #16944, #15328, #15213 ),
 ( #11781, #22232, #3209 ),
 ( #20735, #6531, #13490 ),
 ( #22348, #18902, #17276 ),
 ( #6637, #20507, #13838 ),
 ( #6752, #12024, #4922 ),
 ( #10175, #19018, #10394 ),
 ( #3329, #4814, #1590 ),
 ( #15674, #13940, #1482 ),
 ( #6870, #18783, #13597 ),
 ( #20609, #10286, #15436 ),
 ( #15552, #8696, #3088 ),
 ( #8579, #1248, #12038 ),
 ( #6984, #19243, #17168 ),
 ( #22580, #20855, #9952 ),
 ( #22458, #5159, #10058 ),
 ( #17057, #20961, #12131 ),
 ( #19127, #17393, #1364 ),
 ( #1712, #5262, #17734 ),
 ( #2161, #15780, #10971 ),
 ( #17963, #12565, #21405 ),
 ( #5584, #4002, #19362 ),
 ( #14048, #16009, #16235 ),
 ( #21523, #10852, #200 ),
 ( #9029, #19576, #7194 ),
 ( #2267, #9250, #12350 ),
 ( #5704, #10510, #19699 ),
 ( #21068, #5824, #19465 ),
 ( #12792, #90, #3885 ),
 ( #3553, #1828, #14164 ),
 ( #12677, #2041, #545 ),
 ( #7541, #14513, #17515 ) ),
 .UNSPECIFIED., .F., .F., .F. ) 
 B_SPLINE_SURFACE_WITH_KNOTS ( ( 4, 2, 2, 2, 2, 2, 2, 2, 2, 2, 2, 2, 2, 2, 2, 2, 2, 2, 4 ),
 ( 3, 3 ),
 ( -1.734723475976807094E-18, 0.005809515383400554699, 0.008714273075100833349, 0.01161903076680111113, 0.01452378845850138891, 0.01742854615020166670, 0.02033330384190194795, 0.02178568268775208511, 0.02323806153360222573, 0.02614281922530250352, 0.02759519807115264414, 0.02904757691700278477, 0.03485709230040334033, 0.03630947114625347749, 0.03776184999210362159, 0.04066660768380389590, 0.04211898652965403306, 0.04357136537550417021, 0.04647612306720445147 ),
 ( 0.000000000000000000, 1.000000000000000000 ),
 .UNSPECIFIED. ) 
 GEOMETRIC_REPRESENTATION_ITEM ( )  RATIONAL_B_SPLINE_SURFACE ( (
 ( 1.000000000000000000, 0.6290213284793358950, 1.000000000000000000),
 ( 1.000000000000000000, 0.6248939334222242126, 1.000000000000000000),
 ( 1.000000000000000000, 0.6231525367047958675, 1.000000000000000000),
 ( 1.000000000000000000, 0.6225790212150504876, 1.000000000000000000),
 ( 1.000000000000000000, 0.6227321005840230628, 1.000000000000000000),
 ( 1.000000000000000000, 0.6234255931483526636, 1.000000000000000000),
 ( 1.000000000000000000, 0.6239617638515310150, 1.000000000000000000),
 ( 1.000000000000000000, 0.6251439415235403585, 1.000000000000000000),
 ( 1.000000000000000000, 0.6257917911443122705, 1.000000000000000000),
 ( 1.000000000000000000, 0.6269741839743763201, 1.000000000000000000),
 ( 1.000000000000000000, 0.6274966600224941571, 1.000000000000000000),
 ( 1.000000000000000000, 0.6282667852389499652, 1.000000000000000000),
 ( 1.000000000000000000, 0.6285148504006200509, 1.000000000000000000),
 ( 1.000000000000000000, 0.6286307432043518606, 1.000000000000000000),
 ( 1.000000000000000000, 0.6286269973793257027, 1.000000000000000000),
 ( 1.000000000000000000, 0.6285335994514142932, 1.000000000000000000),
 ( 1.000000000000000000, 0.6284444584878937645, 1.000000000000000000),
 ( 1.000000000000000000, 0.6280613430733316127, 1.000000000000000000),
 ( 1.000000000000000000, 0.6276496514148416361, 1.000000000000000000),
 ( 1.000000000000000000, 0.6268798492417411161, 1.000000000000000000),
 ( 1.000000000000000000, 0.6265983628751120582, 1.000000000000000000),
 ( 1.000000000000000000, 0.6260058463377161653, 1.000000000000000000),
 ( 1.000000000000000000, 0.6256937179553445638, 1.000000000000000000),
 ( 1.000000000000000000, 0.6241358698944529104, 1.000000000000000000),
 ( 1.000000000000000000, 0.6228888902097833302, 1.000000000000000000),
 ( 1.000000000000000000, 0.6226627606242427504, 1.000000000000000000),
 ( 1.000000000000000000, 0.6226866229701819577, 1.000000000000000000),
 ( 1.000000000000000000, 0.6229108014427029438, 1.000000000000000000),
 ( 1.000000000000000000, 0.6231102808941239024, 1.000000000000000000),
 ( 1.000000000000000000, 0.6240167787609354200, 1.000000000000000000),
 ( 1.000000000000000000, 0.6250322308934098681, 1.000000000000000000),
 ( 1.000000000000000000, 0.6273487183755138696, 1.000000000000000000),
 ( 1.000000000000000000, 0.6282530044593889196, 1.000000000000000000),
 ( 1.000000000000000000, 0.6303541273113951737, 1.000000000000000000),
 ( 1.000000000000000000, 0.6315549423243406180, 1.000000000000000000),
 ( 1.000000000000000000, 0.6356032421438199131, 1.000000000000000000),
 ( 1.000000000000000000, 0.6388921020274636042, 1.000000000000000000),
 ( 1.000000000000000000, 0.6428092274089118874, 1.000000000000000000) ) ) 
 REPRESENTATION_ITEM ( '' )  SURFACE ( )  );
#15993=VECTOR ( 'NONE', #3571, 1000.000000000000000 ) ;
#15994=AXIS2_PLACEMENT_3D ( 'NONE', #15941, #254, #21231 ) ;
#15995=CARTESIAN_POINT ( 'NONE',  ( -1.387778780781445676E-14, 20.00000000000000000, -105.0020000000000095 ) ) ;
#15997=VERTEX_POINT ( 'NONE', #10858 ) ;
#16006=VECTOR ( 'NONE', #18129, 1000.000000000000000 ) ;
#16009=CARTESIAN_POINT ( 'NONE',  ( -15.13173276104699916, 33.09480349269330901, -56.64473394289596797 ) ) ;
#16011=AXIS2_PLACEMENT_3D ( 'NONE', #17056, #13837, #20734 ) ;
#16013=EDGE_LOOP ( 'NONE', ( #20647, #9304, #1327, #420, #1896, #13169 ) ) ;
#16015=AXIS2_PLACEMENT_3D ( 'NONE', #4773, #11631, #6702 ) ;
#16018=CARTESIAN_POINT ( 'NONE',  ( 37.09999999999980957, 28.00000000000000000, 54.99999999999922551 ) ) ;
#16019=ORIENTED_EDGE ( 'NONE', *, *, #16660, .F. ) ;
#16021=PLANE ( 'NONE',  #16332 ) ;
#16024=AXIS2_PLACEMENT_3D ( 'NONE', #18081, #21762, #18421 ) ;
#16029=AXIS2_PLACEMENT_3D ( 'NONE', #5954, #19828, #4130 ) ;
#16031=CARTESIAN_POINT ( 'NONE',  ( 0.2573513720701691709, 39.99960945924427591, -48.93325617798620897 ) ) ;
#16033=CARTESIAN_POINT ( 'NONE',  ( -10.30713387248692037, 2.842164160680662466, 57.27491564205614338 ) ) ;
#16037=EDGE_CURVE ( 'NONE', #5360, #16994, #14286, .T. ) ;
#16038=CARTESIAN_POINT ( 'NONE',  ( -8.687717822783543653, 39.99999999999999289, 53.22563407722359585 ) ) ;
#16040=DIRECTION ( 'NONE',  ( -0.000000000000000000, -1.000000000000000000, -0.000000000000000000 ) ) ;
#16041=CARTESIAN_POINT ( 'NONE',  ( 22.25047517524400931, 22.91581175091616274, -58.62998360803280207 ) ) ;
#16044=CIRCLE ( 'NONE', #6909, 2.525000000000110489 ) ;
#16046=CARTESIAN_POINT ( 'NONE',  ( -9.689843208404443686, 39.33333333333332860, 54.54983754392751649 ) ) ;
#16047=CARTESIAN_POINT ( 'NONE',  ( -34.99999999999980815, 28.00000000000000000, 54.99999999999922551 ) ) ;
#16048=VECTOR ( 'NONE', #8385, 1000.000000000000000 ) ;
#16049=CARTESIAN_POINT ( 'NONE',  ( -4.589694866125703321, 39.86882942939622154, -51.95767931116155580 ) ) ;
#16050=VERTEX_POINT ( 'NONE', #787 ) ;
#16052=CARTESIAN_POINT ( 'NONE',  ( -35.00000000000000000, 0.000000000000000000, 1.387778780781445676E-14 ) ) ;
#16058=EDGE_LOOP ( 'NONE', ( #6154, #4248, #4188, #2425 ) ) ;
#16062=DIRECTION ( 'NONE',  ( -0.000000000000000000, -1.000000000000000000, -0.000000000000000000 ) ) ;
#16065=CARTESIAN_POINT ( 'NONE',  ( 6.975411441287900693, 40.00000000000000000, 52.53649951873629931 ) ) ;
#16068=DIRECTION ( 'NONE',  ( -1.000000000000000000, 0.000000000000000000, 0.000000000000000000 ) ) ;
#16072=CARTESIAN_POINT ( 'NONE',  ( -20.89754528720910898, 28.21939688025628357, -58.32034131438403080 ) ) ;
#16073=DIRECTION ( 'NONE',  ( -0.000000000000000000, 1.000000000000000000, -0.000000000000000000 ) ) ;
#16074=ORIENTED_EDGE ( 'NONE', *, *, #4292, .F. ) ;
#16075=CARTESIAN_POINT ( 'NONE',  ( 1.438414332627902414, -1.268869129817755681, 49.24051559643875464 ) ) ;
#16081=CIRCLE ( 'NONE', #1085, 2.499999999999998668 ) ;
#16082=CARTESIAN_POINT ( 'NONE',  ( 21.32169069720648835, 26.98977702688153357, 58.42023943869689617 ) ) ;
#16083=LINE ( 'NONE', #12976, #5579 ) ;
#16084=FACE_BOUND ( 'NONE', #7674, .T. ) ;
#16085=ORIENTED_EDGE ( 'NONE', *, *, #14483, .F. ) ;
#16089=ORIENTED_EDGE ( 'NONE', *, *, #9396, .T. ) ;
#16091=CARTESIAN_POINT ( 'NONE',  ( -42.50000000000000711, -12.00000000000012434, -47.50000000000000000 ) ) ;
#16096=CARTESIAN_POINT ( 'NONE',  ( 7.505578006071305985, 1.461761173326671104, 55.63523492903841117 ) ) ;
#16099=CYLINDRICAL_SURFACE ( 'NONE', #18516, 2.099999999999990763 ) ;
#16100=CARTESIAN_POINT ( 'NONE',  ( 35.00000000000000000, 39.00000000000000711, 4.258610482196280173E-15 ) ) ;
#16101=CARTESIAN_POINT ( 'NONE',  ( 14.99999999999998579, 20.00000000000000355, -101.0000000000000284 ) ) ;
#16103=ADVANCED_FACE ( 'NONE', ( #11085 ), #21991, .T. ) ;
#16110=ORIENTED_EDGE ( 'NONE', *, *, #14065, .T. ) ;
#16113=AXIS2_PLACEMENT_3D ( 'NONE', #6810, #20790, #12182 ) ;
#16118=DIRECTION ( 'NONE',  ( -0.000000000000000000, -0.000000000000000000, 1.000000000000000000 ) ) ;
#16122=CARTESIAN_POINT ( 'NONE',  ( -5.666159602074104740, 39.18446031140960883, -54.55708815122285671 ) ) ;
#16125=ADVANCED_FACE ( 'NONE', ( #6174 ), #20380, .F. ) ;
#16126=ORIENTED_EDGE ( 'NONE', *, *, #21275, .F. ) ;
#16128=DIRECTION ( 'NONE',  ( 0.000000000000000000, 0.000000000000000000, -1.000000000000000000 ) ) ;
#16129=CARTESIAN_POINT ( 'NONE',  ( -35.00000000000058265, 26.00000000000000355, -57.10000000000076170 ) ) ;
#16130=CARTESIAN_POINT ( 'NONE',  ( 14.30046708970552061, 2.690036953684188159, -56.32185947139154791 ) ) ;
#16131=EDGE_LOOP ( 'NONE', ( #6540, #819, #7949, #6581 ) ) ;
#16134=ADVANCED_FACE ( 'NONE', ( #15076, #1228 ), #10467, .F. ) ;
#16139=CARTESIAN_POINT ( 'NONE',  ( 10.50000000000024514, -2.516660498395250301, 100.0000000000000000 ) ) ;
#16140=CARTESIAN_POINT ( 'NONE',  ( -7.364735830101260206, 40.00000000000001421, 52.70305158486502961 ) ) ;
#16141=ORIENTED_EDGE ( 'NONE', *, *, #16512, .F. ) ;
#16142=LINE ( 'NONE', #16266, #6541 ) ;
#16148=VERTEX_POINT ( 'NONE', #16825 ) ;
#16149=FACE_OUTER_BOUND ( 'NONE', #17838, .T. ) ;
#16151=CARTESIAN_POINT ( 'NONE',  ( -1.943364650768838686, 39.97741567493590509, -50.18563800799666552 ) ) ;
#16152=ORIENTED_EDGE ( 'NONE', *, *, #2893, .F. ) ;
#16159=VERTEX_POINT ( 'NONE', #19200 ) ;
#16162=VERTEX_POINT ( 'NONE', #8120 ) ;
#16163=CARTESIAN_POINT ( 'NONE',  ( 19.99999999999999645, 20.48974789854085543, 60.62177826491085142 ) ) ;
#16164=CARTESIAN_POINT ( 'NONE',  ( 34.99999999999980815, 40.00000000000000711, 54.99999999999922551 ) ) ;
#16167=CARTESIAN_POINT ( 'NONE',  ( 5.398828385724590895, 39.81726480423273529, -52.45277685974432558 ) ) ;
#16170=DIRECTION ( 'NONE',  ( 0.000000000000000000, 0.000000000000000000, -1.000000000000000000 ) ) ;
#16172=ORIENTED_EDGE ( 'NONE', *, *, #6712, .T. ) ;
#16174=ADVANCED_FACE ( 'NONE', ( #2736 ), #2699, .F. ) ;
#16175=CARTESIAN_POINT ( 'NONE',  ( -0.4182360581324739424, -0.02262178349794176369, 49.14752433807508680 ) ) ;
#16176=EDGE_CURVE ( 'NONE', #13273, #18704, #15169, .T. ) ;
#16177=CARTESIAN_POINT ( 'NONE',  ( -22.39119123459440530, 18.77992731964037532, -58.66020055843083014 ) ) ;
#16180=DIRECTION ( 'NONE',  ( 0.000000000000000000, 0.000000000000000000, 1.000000000000000000 ) ) ;
#16184=EDGE_CURVE ( 'NONE', #16203, #5122, #20104, .T. ) ;
#16186=ORIENTED_EDGE ( 'NONE', *, *, #15397, .F. ) ;
#16187=CARTESIAN_POINT ( 'NONE',  ( 9.750126048355683750, 40.00000000000000000, -53.58570024001794962 ) ) ;
#16188=CARTESIAN_POINT ( 'NONE',  ( 19.34774434964850798, 25.08511355156644385, 60.46357625386934842 ) ) ;
#16191=B_SPLINE_CURVE_WITH_KNOTS ( 'NONE', 3,
 ( #7403, #5683, #12658, #11745, #13328, #4775, #13217, #20355, #4877, #1102, #20467, #2941, #13114, #20238, #18739, #3047, #6596, #4545, #18636, #1204, #9915, #13447, #15053, #7980 ),
 .UNSPECIFIED., .F., .F.,
 ( 4, 2, 2, 2, 2, 2, 2, 2, 2, 2, 2, 4 ),
 ( 0.01913044734024341512, 0.02058416378663297658, 0.02203788023302254151, 0.02494531312580167484, 0.02639902957219124671, 0.02785274601858081858, 0.03076017891135996579, 0.03221389535774953072, 0.03366761180413910259, 0.03657504469691824633, 0.03948247758969737620, 0.04238991048247651994 ),
 .UNSPECIFIED. ) ;
#16196=ORIENTED_EDGE ( 'NONE', *, *, #14488, .T. ) ;
#16198=ORIENTED_EDGE ( 'NONE', *, *, #14699, .T. ) ;
#16199=ORIENTED_EDGE ( 'NONE', *, *, #9996, .F. ) ;
#16200=FACE_OUTER_BOUND ( 'NONE', #3485, .T. ) ;
#16201=DIRECTION ( 'NONE',  ( 0.000000000000000000, -1.000000000000000000, 0.000000000000000000 ) ) ;
#16202=DIRECTION ( 'NONE',  ( -0.000000000000000000, 1.000000000000000000, -0.000000000000000000 ) ) ;
#16203=VERTEX_POINT ( 'NONE', #14590 ) ;
#16204=CARTESIAN_POINT ( 'NONE',  ( 35.00000000000000000, 2.142135623730931471, -59.99999999999999289 ) ) ;
#16208=CYLINDRICAL_SURFACE ( 'NONE', #22178, 2.499999999999995115 ) ;
#16209=AXIS2_PLACEMENT_3D ( 'NONE', #9257, #19811, #9151 ) ;
#16211=CARTESIAN_POINT ( 'NONE',  ( -35.00000000000000000, 40.00000000000000000, 1.387778780781445676E-14 ) ) ;
#16215=EDGE_CURVE ( 'NONE', #2243, #4414, #3854, .T. ) ;
#16217=CARTESIAN_POINT ( 'NONE',  ( -34.99999999999980815, 28.00000000000000000, 54.99999999999922551 ) ) ;
#16218=CARTESIAN_POINT ( 'NONE',  ( -5.617777150769229344, 39.81214432327088559, 52.56494788744241475 ) ) ;
#16219=ADVANCED_FACE ( 'NONE', ( #18369, #11152 ), #12862, .F. ) ;
#16220=DIRECTION ( 'NONE',  ( 0.000000000000000000, 0.000000000000000000, -1.000000000000000000 ) ) ;
#16221=EDGE_LOOP ( 'NONE', ( #5618, #9717, #12638, #16085 ) ) ;
#16226=ORIENTED_EDGE ( 'NONE', *, *, #13579, .F. ) ;
#16229=CARTESIAN_POINT ( 'NONE',  ( -28.50000000000001421, 19.99999999999982947, -100.0000000000000000 ) ) ;
#16233=DIRECTION ( 'NONE',  ( 0.000000000000000000, 0.000000000000000000, -1.000000000000000000 ) ) ;
#16234=CARTESIAN_POINT ( 'NONE',  ( -13.76051559511277134, 5.481080969678175485, 58.73291665846262077 ) ) ;
#16235=CARTESIAN_POINT ( 'NONE',  ( -16.86064470394645909, 34.83129639055714932, -57.19330778950705962 ) ) ;
#16237=CIRCLE ( 'NONE', #22475, 2.099999999999997868 ) ;
#16241=CARTESIAN_POINT ( 'NONE',  ( -1.575352350797029954, 39.94051438458651404, -50.55779643183547734 ) ) ;
#16243=FACE_OUTER_BOUND ( 'NONE', #1954, .T. ) ;
#16245=ORIENTED_EDGE ( 'NONE', *, *, #4668, .T. ) ;
#16248=FACE_OUTER_BOUND ( 'NONE', #5870, .T. ) ;
#16249=FACE_OUTER_BOUND ( 'NONE', #14570, .T. ) ;
#16252=AXIS2_PLACEMENT_3D ( 'NONE', #12576, #19589, #6683 ) ;
#16255=LINE ( 'NONE', #564, #10023 ) ;
#16256=FACE_OUTER_BOUND ( 'NONE', #5228, .T. ) ;
#16257=CIRCLE ( 'NONE', #20303, 2.099999999999997868 ) ;
#16260=DIRECTION ( 'NONE',  ( 0.000000000000000000, -0.000000000000000000, -1.000000000000000000 ) ) ;
#16263=DIRECTION ( 'NONE',  ( -0.5840452403773163104, -0.8117211080122302969, 0.000000000000000000 ) ) ;
#16264=CARTESIAN_POINT ( 'NONE',  ( -13.56354382738803466, 2.142135623730932803, -56.03997097393685323 ) ) ;
#16265=EDGE_LOOP ( 'NONE', ( #5173, #21213, #10359, #19795 ) ) ;
#16266=CARTESIAN_POINT ( 'NONE',  ( 28.49999999999998224, 19.99999999999999645, 60.00099999999999767 ) ) ;
#16268=DIRECTION ( 'NONE',  ( -1.000000000000000000, 0.000000000000000000, 0.000000000000000000 ) ) ;
#16269=DIRECTION ( 'NONE',  ( -0.000000000000000000, -0.000000000000000000, -1.000000000000000000 ) ) ;
#16272=AXIS2_PLACEMENT_3D ( 'NONE', #4688, #13361, #1350 ) ;
#16274=CARTESIAN_POINT ( 'NONE',  ( -0.2542263435710383490, 39.99961927927021321, -48.93085139008606888 ) ) ;
#16277=CARTESIAN_POINT ( 'NONE',  ( 7.505578006071305097, 1.461761173326674434, 55.63523492903841117 ) ) ;
#16279=CARTESIAN_POINT ( 'NONE',  ( -1.387778780781445676E-14, 20.00000000000000000, -98.00000000000000000 ) ) ;
#16286=ORIENTED_EDGE ( 'NONE', *, *, #22109, .T. ) ;
#16290=DIRECTION ( 'NONE',  ( 0.000000000000000000, 0.000000000000000000, 1.000000000000000000 ) ) ;
#16295=ORIENTED_EDGE ( 'NONE', *, *, #10561, .F. ) ;
#16296=DIRECTION ( 'NONE',  ( -0.000000000000000000, 1.000000000000000000, -0.000000000000000000 ) ) ;
#16301=ORIENTED_EDGE ( 'NONE', *, *, #1258, .F. ) ;
#16302=CARTESIAN_POINT ( 'NONE',  ( 7.464609744079063525, 38.57206862716381579, 54.30635410445871258 ) ) ;
#16304=CARTESIAN_POINT ( 'NONE',  ( 7.505578006071305985, 1.461761173326671104, 55.63523492903841117 ) ) ;
#16307=ORIENTED_EDGE ( 'NONE', *, *, #6467, .F. ) ;
#16310=CARTESIAN_POINT ( 'NONE',  ( 13.83098800442548004, 37.66187182509651876, 56.14292165594093831 ) ) ;
#16311=AXIS2_PLACEMENT_3D ( 'NONE', #7763, #7423, #21406 ) ;
#16312=TOROIDAL_SURFACE ( 'NONE', #12282, 18.00000000000000355, 4.000000000000000000 ) ;
#16313=CARTESIAN_POINT ( 'NONE',  ( -42.50000000000000711, -12.00000000000000000, -47.50000000000000000 ) ) ;
#16314=EDGE_CURVE ( 'NONE', #22397, #10118, #6680, .T. ) ;
#16315=EDGE_CURVE ( 'NONE', #18097, #21198, #9349, .T. ) ;
#16321=CIRCLE ( 'NONE', #6454, 2.499999999999995115 ) ;
#16322=AXIS2_PLACEMENT_3D ( 'NONE', #21323, #14199, #21214 ) ;
#16323=ORIENTED_EDGE ( 'NONE', *, *, #10704, .T. ) ;
#16327=CARTESIAN_POINT ( 'NONE',  ( 8.256135806682694422, -0.3920627093389359996, -55.63523492904086254 ) ) ;
#16328=EDGE_CURVE ( 'NONE', #8737, #6835, #17319, .T. ) ;
#16331=CARTESIAN_POINT ( 'NONE',  ( -6.699391982050521221, -4.821764332415714449, 49.69317737456928796 ) ) ;
#16332=AXIS2_PLACEMENT_3D ( 'NONE', #17975, #7326, #12692 ) ;
#16334=DIRECTION ( 'NONE',  ( -0.000000000000000000, -1.000000000000000000, -0.000000000000000000 ) ) ;
#16338=DIRECTION ( 'NONE',  ( 0.000000000000000000, 0.000000000000000000, 1.000000000000000000 ) ) ;
#16343=ORIENTED_EDGE ( 'NONE', *, *, #22508, .F. ) ;
#16348=DIRECTION ( 'NONE',  ( -0.000000000000000000, 1.000000000000000000, -0.000000000000000000 ) ) ;
#16350=FACE_OUTER_BOUND ( 'NONE', #12615, .T. ) ;
#16352=EDGE_CURVE ( 'NONE', #8568, #8737, #11548, .T. ) ;
#16353=CARTESIAN_POINT ( 'NONE',  ( 19.99999999999998579, 20.00000000000000000, -105.0020000000000095 ) ) ;
#16356=CARTESIAN_POINT ( 'NONE',  ( 35.00000000000000000, 40.00000000000000000, 4.258610482196280173E-15 ) ) ;
#16358=ORIENTED_EDGE ( 'NONE', *, *, #9608, .T. ) ;
#16362=VERTEX_POINT ( 'NONE', #8401 ) ;
#16365=DIRECTION ( 'NONE',  ( 1.000000000000000000, 0.000000000000000000, 0.000000000000000000 ) ) ;
#16372=AXIS2_PLACEMENT_3D ( 'NONE', #18346, #2896, #6317 ) ;
#16375=CARTESIAN_POINT ( 'NONE',  ( 0.2763232317742203015, 39.99954927670500382, -48.94786180895853533 ) ) ;
#16380=EDGE_LOOP ( 'NONE', ( #1511, #14129, #20322 ) ) ;
#16381=LINE ( 'NONE', #14869, #21682 ) ;
#16382=DIRECTION ( 'NONE',  ( -0.000000000000000000, -0.000000000000000000, 1.000000000000000000 ) ) ;
#16384=CARTESIAN_POINT ( 'NONE',  ( -90.00000000000000000, 26.00000000000000355, 2.099999999999989875 ) ) ;
#16385=AXIS2_PLACEMENT_3D ( 'NONE', #7309, #21287, #5578 ) ;
#16386=CARTESIAN_POINT ( 'NONE',  ( 12.59807286780800517, 38.55590838447054836, -55.66678043528290232 ) ) ;
#16389=CARTESIAN_POINT ( 'NONE',  ( 14.99999999999998579, 20.00000000000000000, 45.82575694955838230 ) ) ;
#16390=DIRECTION ( 'NONE',  ( 0.000000000000000000, 0.000000000000000000, 1.000000000000000000 ) ) ;
#16391=DIRECTION ( 'NONE',  ( 0.000000000000000000, 0.000000000000000000, -1.000000000000000000 ) ) ;
#16392=EDGE_CURVE ( 'NONE', #8904, #3548, #20656, .T. ) ;
#16399=B_SPLINE_CURVE_WITH_KNOTS ( 'NONE', 3,
 ( #17248, #13682, #20696, #6953 ),
 .UNSPECIFIED., .F., .F.,
 ( 4, 4 ),
 ( 0.000000000000000000, 1.000000000000000000 ),
 .UNSPECIFIED. ) ;
#16402=ORIENTED_EDGE ( 'NONE', *, *, #1668, .F. ) ;
#16403=VERTEX_POINT ( 'NONE', #15481 ) ;
#16404=ORIENTED_EDGE ( 'NONE', *, *, #5039, .T. ) ;
#16406=FACE_OUTER_BOUND ( 'NONE', #18563, .T. ) ;
#16408=VECTOR ( 'NONE', #4412, 1000.000000000000000 ) ;
#16410=EDGE_LOOP ( 'NONE', ( #14448, #19090 ) ) ;
#16412=DIRECTION ( 'NONE',  ( 0.000000000000000000, 0.000000000000000000, -1.000000000000000000 ) ) ;
#16417=CIRCLE ( 'NONE', #10550, 2.000000000000001776 ) ;
#16419=ORIENTED_EDGE ( 'NONE', *, *, #17725, .F. ) ;
#16420=LINE ( 'NONE', #12541, #11981 ) ;
#16422=ORIENTED_EDGE ( 'NONE', *, *, #3298, .F. ) ;
#16423=CARTESIAN_POINT ( 'NONE',  ( 0.6290164960638020553, 40.00000000000000000, 49.48738346577131608 ) ) ;
#16424=EDGE_CURVE ( 'NONE', #9683, #22506, #8289, .T. ) ;
#16428=ORIENTED_EDGE ( 'NONE', *, *, #2148, .T. ) ;
#16434=VECTOR ( 'NONE', #19891, 1000.000000000000000 ) ;
#16436=ORIENTED_EDGE ( 'NONE', *, *, #785, .T. ) ;
#16438=EDGE_LOOP ( 'NONE', ( #12870, #11034, #13141, #22662 ) ) ;
#16440=LINE ( 'NONE', #629, #10686 ) ;
#16443=DIRECTION ( 'NONE',  ( 0.000000000000000000, -1.000000000000000000, 0.000000000000000000 ) ) ;
#16445=ORIENTED_EDGE ( 'NONE', *, *, #20711, .F. ) ;
#16449=ORIENTED_EDGE ( 'NONE', *, *, #22403, .F. ) ;
#16450=CARTESIAN_POINT ( 'NONE',  ( -35.00000000000000000, 39.00000000000000711, 1.387778780781445676E-14 ) ) ;
#16451=LINE ( 'NONE', #523, #9077 ) ;
#16456=DIRECTION ( 'NONE',  ( 0.000000000000000000, 0.000000000000000000, -1.000000000000000000 ) ) ;
#16458=CARTESIAN_POINT ( 'NONE',  ( -4.628075497662138105, 39.46063506869889892, 53.65703709786524200 ) ) ;
#16459=DIRECTION ( 'NONE',  ( -0.000000000000000000, -1.000000000000000000, -0.000000000000000000 ) ) ;
#16467=CARTESIAN_POINT ( 'NONE',  ( -3.125929443366052940, 0.2354807939734264444, -52.75540126681803343 ) ) ;
#16468=CARTESIAN_POINT ( 'NONE',  ( 2.517875701377081388, 0.1458803431931041672, -52.33410116371747733 ) ) ;
#16470=CARTESIAN_POINT ( 'NONE',  ( 9.412328935320623680E-15, -0.02544136969053066924, 50.05036128709051013 ) ) ;
#16471=FACE_OUTER_BOUND ( 'NONE', #21666, .T. ) ;
#16472=CARTESIAN_POINT ( 'NONE',  ( -3.630514520980234749, 39.68566286778591490, -51.94955441408608721 ) ) ;
#16475=DIRECTION ( 'NONE',  ( -1.000000000000000000, 0.000000000000000000, 0.000000000000000000 ) ) ;
#16480=DIRECTION ( 'NONE',  ( 8.659560562354932858E-17, 0.7071067811865474617, -0.7071067811865474617 ) ) ;
#16484=DIRECTION ( 'NONE',  ( -0.000000000000000000, 1.000000000000000000, -0.000000000000000000 ) ) ;
#16491=ORIENTED_EDGE ( 'NONE', *, *, #19281, .T. ) ;
#16492=CARTESIAN_POINT ( 'NONE',  ( 5.724878023121393156, 39.79387150756618752, -52.64592485981327030 ) ) ;
#16493=CARTESIAN_POINT ( 'NONE',  ( 11.15511648635847486, 39.11609166919295433, 55.07420106208768829 ) ) ;
#16495=DIRECTION ( 'NONE',  ( 8.659560562355143632E-17, -0.7071067811865302533, 0.7071067811865647812 ) ) ;
#16496=CONICAL_SURFACE ( 'NONE', #14653, 2.099999999999997868, 1.029744258676652091 ) ;
#16498=CARTESIAN_POINT ( 'NONE',  ( -13.56209497732963953, 5.196600802657145302, -56.07847567635086961 ) ) ;
#16499=DIRECTION ( 'NONE',  ( 8.659560562353731078E-17, 0.7071067811866457165, -0.7071067811864494290 ) ) ;
#16502=ORIENTED_EDGE ( 'NONE', *, *, #1633, .T. ) ;
#16504=CARTESIAN_POINT ( 'NONE',  ( 25.99999999999998579, 19.99999999999999645, -100.0000000000000000 ) ) ;
#16505=CARTESIAN_POINT ( 'NONE',  ( -0.05876574830816937850, 39.99997969038122392, -48.77966625399992040 ) ) ;
#16507=VERTEX_POINT ( 'NONE', #9074 ) ;
#16508=CARTESIAN_POINT ( 'NONE',  ( 8.219889501002811016, 1.750964516533572102, 56.08920281152157372 ) ) ;
#16509=CARTESIAN_POINT ( 'NONE',  ( 9.165151389911692092, 40.00000000000000000, 56.36098470834080842 ) ) ;
#16512=EDGE_CURVE ( 'NONE', #2477, #12153, #4239, .T. ) ;
#16517=EDGE_LOOP ( 'NONE', ( #1193, #9338, #22290, #19037 ) ) ;
#16518=CARTESIAN_POINT ( 'NONE',  ( 13.28791054760747947, 34.95496542652811200, -58.55506233662529780 ) ) ;
#16519=DIRECTION ( 'NONE',  ( 0.000000000000000000, 0.000000000000000000, 1.000000000000000000 ) ) ;
#16520=CYLINDRICAL_SURFACE ( 'NONE', #14271, 2.099999999999997868 ) ;
#16522=DIRECTION ( 'NONE',  ( -0.7071067811865463515, 8.659560562354918067E-17, 0.7071067811865487940 ) ) ;
#16530=AXIS2_PLACEMENT_3D ( 'NONE', #3230, #17189, #3109 ) ;
#16531=CARTESIAN_POINT ( 'NONE',  ( 42.50000000000000711, -12.00000000000000000, -47.50000000000000000 ) ) ;
#16533=FACE_OUTER_BOUND ( 'NONE', #10318, .T. ) ;
#16534=DIRECTION ( 'NONE',  ( 1.000000000000000000, 0.000000000000000000, 0.000000000000000000 ) ) ;
#16535=ORIENTED_EDGE ( 'NONE', *, *, #4145, .T. ) ;
#16536=CARTESIAN_POINT ( 'NONE',  ( 4.750157590145799524, 39.43751370096379816, 52.76321277951888078 ) ) ;
#16539=CARTESIAN_POINT ( 'NONE',  ( -4.664248763237361928, 0.4975022168800966038, -53.81010167002803257 ) ) ;
#16541=CARTESIAN_POINT ( 'NONE',  ( 13.09671971564443105, 38.20119746052611021, 55.86054988736559324 ) ) ;
#16544=CARTESIAN_POINT ( 'NONE',  ( 0.000000000000000000, -5.000000000000000000, 9.068199145005368464E-15 ) ) ;
#16545=ORIENTED_EDGE ( 'NONE', *, *, #5405, .T. ) ;
#16552=DIRECTION ( 'NONE',  ( 0.000000000000000000, 1.000000000000000000, 0.000000000000000000 ) ) ;
#16553=EDGE_LOOP ( 'NONE', ( #11622, #9901, #8861, #9908 ) ) ;
#16556=EDGE_LOOP ( 'NONE', ( #10789, #6348, #10397, #2977 ) ) ;
#16560=CARTESIAN_POINT ( 'NONE',  ( -9.952189117650803496, 40.00000000000000000, 53.64426396172073908 ) ) ;
#16565=CARTESIAN_POINT ( 'NONE',  ( -2.576224933359605451, 39.84426458497861745, 51.65025110504824113 ) ) ;
#16568=ORIENTED_EDGE ( 'NONE', *, *, #7122, .T. ) ;
#16569=ORIENTED_EDGE ( 'NONE', *, *, #12117, .T. ) ;
#16571=EDGE_LOOP ( 'NONE', ( #8658, #21185 ) ) ;
#16572=CARTESIAN_POINT ( 'NONE',  ( -19.88905041090809434, 17.72428093568618479, 58.11830361000903622 ) ) ;
#16580=CARTESIAN_POINT ( 'NONE',  ( -5.905663676014976105, 39.12131202908561534, -53.51378431580162953 ) ) ;
#16583=EDGE_LOOP ( 'NONE', ( #22520, #6130, #979, #283 ) ) ;
#16584=DIRECTION ( 'NONE',  ( -0.000000000000000000, 1.000000000000000000, -0.000000000000000000 ) ) ;
#16585=CARTESIAN_POINT ( 'NONE',  ( 42.50000000000000711, -5.000000000000000000, 47.50000000000000711 ) ) ;
#16587=CARTESIAN_POINT ( 'NONE',  ( -90.00000000000000000, 40.00000000000000711, 2.524999999999998579 ) ) ;
#16599=EDGE_LOOP ( 'NONE', ( #9550, #9237 ) ) ;
#16602=AXIS2_PLACEMENT_3D ( 'NONE', #17353, #14005, #19320 ) ;
#16603=CARTESIAN_POINT ( 'NONE',  ( 42.50000000000000711, -12.00000000000012434, -47.50000000000000000 ) ) ;
#16604=EDGE_LOOP ( 'NONE', ( #7721, #8430 ) ) ;
#16605=CARTESIAN_POINT ( 'NONE',  ( 42.50000000000000711, -9.600000000000001421, -45.00000000000000000 ) ) ;
#16610=CARTESIAN_POINT ( 'NONE',  ( -34.99999999999980815, 40.00000000000000000, 57.09999999999921982 ) ) ;
#16611=CARTESIAN_POINT ( 'NONE',  ( -16.37028666998709880, 4.520534895874758874, -57.04777702420076935 ) ) ;
#16613=CARTESIAN_POINT ( 'NONE',  ( -0.7796821504949128512, 40.00000000000002132, 49.24007756836347482 ) ) ;
#16614=DIRECTION ( 'NONE',  ( -0.4332438415859285463, 0.000000000000000000, -0.9012767464701765263 ) ) ;
#16615=ORIENTED_EDGE ( 'NONE', *, *, #15331, .F. ) ;
#16618=CARTESIAN_POINT ( 'NONE',  ( -42.50000000000000711, -5.000000000000000000, 47.50000000000000711 ) ) ;
#16619=EDGE_LOOP ( 'NONE', ( #2258, #3544, #8298 ) ) ;
#16621=CIRCLE ( 'NONE', #884, 2.500000000000002220 ) ;
#16622=CARTESIAN_POINT ( 'NONE',  ( -14.40375226887235982, 24.20453657423044902, 45.56106839101557426 ) ) ;
#16626=AXIS2_PLACEMENT_3D ( 'NONE', #14462, #21474, #19870 ) ;
#16632=FACE_OUTER_BOUND ( 'NONE', #4575, .T. ) ;
#16633=DIRECTION ( 'NONE',  ( 0.000000000000000000, 0.000000000000000000, 1.000000000000000000 ) ) ;
#16636=FACE_OUTER_BOUND ( 'NONE', #4947, .T. ) ;
#16637=CARTESIAN_POINT ( 'NONE',  ( 4.076028284553002479, 5.556537143872661844, -39.58813741008490439 ) ) ;
#16638=VERTEX_POINT ( 'NONE', #7922 ) ;
#16640=CARTESIAN_POINT ( 'NONE',  ( -42.50000000000000711, -9.600000000000001421, -45.00000000000000000 ) ) ;
#16642=CARTESIAN_POINT ( 'NONE',  ( 5.833333333333329485, 0.000000000000000000, -40.61164310337066041 ) ) ;
#16644=CARTESIAN_POINT ( 'NONE',  ( 19.60425726290408122, 16.02072691545760463, -60.52684394361300235 ) ) ;
#16645=EDGE_LOOP ( 'NONE', ( #12917, #1473, #16491, #10358 ) ) ;
#16646=CARTESIAN_POINT ( 'NONE',  ( -1.570150081433425937, 40.00000000000000000, -49.72616478525270622 ) ) ;
#16647=CARTESIAN_POINT ( 'NONE',  ( 0.6233897118003356441, 39.99089506582289744, -49.47139888151590270 ) ) ;
#16649=EDGE_LOOP ( 'NONE', ( #9780, #2231, #799 ) ) ;
#16653=CARTESIAN_POINT ( 'NONE',  ( 10.79594548525664699, 39.62239930148019340, 54.90840750699845074 ) ) ;
#16657=CARTESIAN_POINT ( 'NONE',  ( 22.40268525210799311, 21.30540434957255513, -58.66274428449842304 ) ) ;
#16660=EDGE_CURVE ( 'NONE', #5679, #1150, #16669, .T. ) ;
#16661=ORIENTED_EDGE ( 'NONE', *, *, #20797, .F. ) ;
#16664=DIRECTION ( 'NONE',  ( 0.000000000000000000, 0.000000000000000000, -1.000000000000000000 ) ) ;
#16666=CARTESIAN_POINT ( 'NONE',  ( -90.00000000000000000, 39.97500000000000142, -9.108981535246192915E-16 ) ) ;
#16667=CARTESIAN_POINT ( 'NONE',  ( 35.00000000000000000, 40.00000000000000000, -58.99999999999993605 ) ) ;
#16669=CIRCLE ( 'NONE', #6794, 2.499999999999998668 ) ;
#16676=DIRECTION ( 'NONE',  ( 0.000000000000000000, 0.000000000000000000, 1.000000000000000000 ) ) ;
#16678=EDGE_CURVE ( 'NONE', #6038, #22156, #19593, .T. ) ;
#16679=CARTESIAN_POINT ( 'NONE',  ( -7.017626609043913000, 6.725442770851620899, 41.44244536674935375 ) ) ;
#16681=CIRCLE ( 'NONE', #13728, 2.500000000000002220 ) ;
#16684=EDGE_CURVE ( 'NONE', #10389, #19954, #20880, .T. ) ;
#16689=CARTESIAN_POINT ( 'NONE',  ( -19.23518390577171999, 25.54875756131827558, 60.43569366689264655 ) ) ;
#16693=CARTESIAN_POINT ( 'NONE',  ( 1.438414332626293479, -1.268869129819692798, -49.24051559643684328 ) ) ;
#16694=FACE_BOUND ( 'NONE', #15837, .T. ) ;
#16695=EDGE_CURVE ( 'NONE', #10325, #19599, #15189, .T. ) ;
#16696=CARTESIAN_POINT ( 'NONE',  ( 34.99999999999980815, 40.00000000000000000, 54.99999999999922551 ) ) ;
#16697=LINE ( 'NONE', #16353, #4998 ) ;
#16698=CARTESIAN_POINT ( 'NONE',  ( 42.50000000000000711, -5.000000000000000000, -47.50000000000000000 ) ) ;
#16699=AXIS2_PLACEMENT_3D ( 'NONE', #10884, #15806, #21319 ) ;
#16700=CARTESIAN_POINT ( 'NONE',  ( -0.7060534721732323327, 40.00000000000297007, -49.41655051369872353 ) ) ;
#16701=DIRECTION ( 'NONE',  ( 0.000000000000000000, 0.000000000000000000, -1.000000000000000000 ) ) ;
#16703=ORIENTED_EDGE ( 'NONE', *, *, #22394, .F. ) ;
#16704=DIRECTION ( 'NONE',  ( -1.000000000000000000, 0.000000000000000000, 0.000000000000000000 ) ) ;
#16706=DIRECTION ( 'NONE',  ( 0.000000000000000000, -1.000000000000000000, 0.000000000000000000 ) ) ;
#16711=ORIENTED_EDGE ( 'NONE', *, *, #3309, .F. ) ;
#16712=CARTESIAN_POINT ( 'NONE',  ( -4.084299015953638090, -4.682619376883241813, -48.27507093818995543 ) ) ;
#16714=EDGE_CURVE ( 'NONE', #11218, #18097, #3340, .T. ) ;
#16716=CARTESIAN_POINT ( 'NONE',  ( -20.00000000000001421, 20.00000000000000000, -98.00000000000000000 ) ) ;
#16718=ORIENTED_EDGE ( 'NONE', *, *, #5407, .T. ) ;
#16719=CARTESIAN_POINT ( 'NONE',  ( 1.952251977614869904, 39.97720309756248014, -50.19198521789787293 ) ) ;
#16720=CARTESIAN_POINT ( 'NONE',  ( 10.72803533575908119, 39.99999999999999289, 53.87712872072329162 ) ) ;
#16723=CARTESIAN_POINT ( 'NONE',  ( -4.873423496009598566, 40.00000000000000000, 51.54632858871904233 ) ) ;
#16724=CARTESIAN_POINT ( 'NONE',  ( 11.17438353485539615, 39.11312751370834206, -55.08132212994122767 ) ) ;
#16725=CARTESIAN_POINT ( 'NONE',  ( -5.833333333333341919, 33.81926995981417150, -40.61164310337066041 ) ) ;
#16727=VERTEX_POINT ( 'NONE', #13501 ) ;
#16731=DIRECTION ( 'NONE',  ( -0.000000000000000000, -0.000000000000000000, 1.000000000000000000 ) ) ;
#16734=DIRECTION ( 'NONE',  ( -1.000000000000000000, 0.000000000000000000, 0.000000000000000000 ) ) ;
#16736=ORIENTED_EDGE ( 'NONE', *, *, #4990, .F. ) ;
#16741=CONICAL_SURFACE ( 'NONE', #11614, 2.524999999999999467, 0.7853981633973095011 ) ;
#16742=CIRCLE ( 'NONE', #17840, 2.000000000000001776 ) ;
#16748=CARTESIAN_POINT ( 'NONE',  ( 19.85669122310594759, 22.43861522864551006, 60.58781117059878341 ) ) ;
#16749=CARTESIAN_POINT ( 'NONE',  ( 10.49999999999994138, 42.51666049839543149, 100.0000000000000000 ) ) ;
#16750=CARTESIAN_POINT ( 'NONE',  ( -30.00000000000001421, 20.00000000000000711, -105.0000000000000142 ) ) ;
#16751=CARTESIAN_POINT ( 'NONE',  ( 35.00000000000000711, 39.00000000000000711, 49.99999999999999289 ) ) ;
#16753=CARTESIAN_POINT ( 'NONE',  ( 1.054992083789042301, 5.028051073338380306, -38.77590480715000609 ) ) ;
#16755=DIRECTION ( 'NONE',  ( -0.000000000000000000, 1.000000000000000000, -0.000000000000000000 ) ) ;
#16757=ORIENTED_EDGE ( 'NONE', *, *, #17016, .F. ) ;
#16758=CARTESIAN_POINT ( 'NONE',  ( -8.759110511859024228, 7.803016162472655282, -42.56552456877078328 ) ) ;
#16759=DIRECTION ( 'NONE',  ( 0.000000000000000000, 0.000000000000000000, 1.000000000000000000 ) ) ;
#16760=LINE ( 'NONE', #20541, #2400 ) ;
#16762=EDGE_LOOP ( 'NONE', ( #13891, #16286, #16186, #9812 ) ) ;
#16766=EDGE_LOOP ( 'NONE', ( #12808, #4780, #21476, #21494 ) ) ;
#16768=FACE_OUTER_BOUND ( 'NONE', #19633, .T. ) ;
#16770=CONICAL_SURFACE ( 'NONE', #7261, 58.99999999999994316, 0.7853981633974725929 ) ;
#16773=CARTESIAN_POINT ( 'NONE',  ( 11.87139216507892847, 36.11857111619715255, 55.37976054165663697 ) ) ;
#16774=DIRECTION ( 'NONE',  ( -0.000000000000000000, -1.000000000000000000, -0.000000000000000000 ) ) ;
#16776=EDGE_CURVE ( 'NONE', #11978, #15147, #3152, .T. ) ;
#16777=EDGE_CURVE ( 'NONE', #2480, #17245, #3221, .T. ) ;
#16778=CARTESIAN_POINT ( 'NONE',  ( 20.01704759191777683, 20.30656121191836405, -60.62580324356297012 ) ) ;
#16783=EDGE_LOOP ( 'NONE', ( #1920, #15376, #2348, #18607 ) ) ;
#16784=ORIENTED_EDGE ( 'NONE', *, *, #2201, .F. ) ;
#16785=CARTESIAN_POINT ( 'NONE',  ( 11.69583326050833172, 39.02781355202390756, 55.28967510510689465 ) ) ;
#16787=TOROIDAL_SURFACE ( 'NONE', #9096, 22.00000000000000000, 2.000000000000000000 ) ;
#16790=DIRECTION ( 'NONE',  ( -0.000000000000000000, 1.000000000000000000, -0.000000000000000000 ) ) ;
#16793=DIRECTION ( 'NONE',  ( -0.000000000000000000, 1.000000000000000000, -0.000000000000000000 ) ) ;
#16796=DIRECTION ( 'NONE',  ( -0.000000000000000000, -1.000000000000000000, -0.000000000000000000 ) ) ;
#16797=CARTESIAN_POINT ( 'NONE',  ( -42.50000000000000711, -9.600000000000001421, -47.50000000000000000 ) ) ;
#16798=CARTESIAN_POINT ( 'NONE',  ( -0.2573524306472053103, 39.99960945630349585, 48.93325698110795230 ) ) ;
#16803=VERTEX_POINT ( 'NONE', #22128 ) ;
#16804=VERTEX_POINT ( 'NONE', #2381 ) ;
#16806=ORIENTED_EDGE ( 'NONE', *, *, #13890, .T. ) ;
#16807=CARTESIAN_POINT ( 'NONE',  ( -18.09042992579668052, 28.57522027848806800, 57.61279183055282971 ) ) ;
#16808=CARTESIAN_POINT ( 'NONE',  ( -30.00000000000001421, 20.00000000000000355, 100.0000000000000000 ) ) ;
#16809=VECTOR ( 'NONE', #95, 1000.000000000000000 ) ;
#16817=CARTESIAN_POINT ( 'NONE',  ( -6.803227178531130903, 38.81166136533656896, -55.43135129401765226 ) ) ;
#16818=CARTESIAN_POINT ( 'NONE',  ( 35.00000000000058265, 28.00000000000000000, -55.00000000000076028 ) ) ;
#16820=ADVANCED_FACE ( 'NONE', ( #19573 ), #18879, .F. ) ;
#16823=DIRECTION ( 'NONE',  ( 0.000000000000000000, -1.000000000000000000, 0.000000000000000000 ) ) ;
#16824=CARTESIAN_POINT ( 'NONE',  ( -10.48823472894017073, 39.21814192245744124, 54.82890001996310048 ) ) ;
#16825=CARTESIAN_POINT ( 'NONE',  ( 42.50000000000000711, -5.000000000000000000, -54.00000000000000000 ) ) ;
#16834=CARTESIAN_POINT ( 'NONE',  ( -0.6808133077283172740, -3.155657370482437329, 47.81204852682553508 ) ) ;
#16835=AXIS2_PLACEMENT_3D ( 'NONE', #22257, #12044, #13738 ) ;
#16842=CARTESIAN_POINT ( 'NONE',  ( -1.582598045080424232, 40.00000000000000000, 49.73344078919016198 ) ) ;
#16843=CARTESIAN_POINT ( 'NONE',  ( 10.35284963817699300, 39.23826485918397822, -54.78050591800258218 ) ) ;
#16848=DIRECTION ( 'NONE',  ( 0.000000000000000000, 0.000000000000000000, -1.000000000000000000 ) ) ;
#16849=LINE ( 'NONE', #13163, #876 ) ;
#16851=DIRECTION ( 'NONE',  ( 0.000000000000000000, -1.000000000000000000, 0.000000000000000000 ) ) ;
#16861=CARTESIAN_POINT ( 'NONE',  ( 14.32898074910538710, 33.98521869245691107, 58.94425321795622352 ) ) ;
#16864=DIRECTION ( 'NONE',  ( -0.000000000000000000, -0.000000000000000000, 1.000000000000000000 ) ) ;
#16865=CARTESIAN_POINT ( 'NONE',  ( 16.97759837164270280, 9.398593820328089876, 59.81443117571823365 ) ) ;
#16866=CARTESIAN_POINT ( 'NONE',  ( -5.833333333333337478, 6.180730040185833829, -40.61164310337066041 ) ) ;
#16874=DIRECTION ( 'NONE',  ( -0.000000000000000000, 1.000000000000000000, -0.000000000000000000 ) ) ;
#16875=ORIENTED_EDGE ( 'NONE', *, *, #14724, .F. ) ;
#16876=CARTESIAN_POINT ( 'NONE',  ( -2.080482199426275746E-16, 39.99999999999997158, -48.73397172404480671 ) ) ;
#16877=CARTESIAN_POINT ( 'NONE',  ( 4.240361389880744625, 39.54844917561619866, -53.29842195655537296 ) ) ;
#16880=CARTESIAN_POINT ( 'NONE',  ( 0.3444338182180646801, -0.009360450408019541091, -50.24963102686507455 ) ) ;
#16883=DIRECTION ( 'NONE',  ( 0.000000000000000000, 0.000000000000000000, -1.000000000000000000 ) ) ;
#16885=CARTESIAN_POINT ( 'NONE',  ( 19.35294509712666766, 31.41613210955675228, -57.92571537617268973 ) ) ;
#16886=EDGE_CURVE ( 'NONE', #4414, #18864, #2040, .T. ) ;
#16894=EDGE_LOOP ( 'NONE', ( #14979, #4416, #13200, #21006 ) ) ;
#16896=CARTESIAN_POINT ( 'NONE',  ( -3.309563215937974423, -3.140776953258733517, -49.61090469809253278 ) ) ;
#16903=CARTESIAN_POINT ( 'NONE',  ( -35.00000000000058265, 39.97500000000000142, -55.00000000000076028 ) ) ;
#16906=CIRCLE ( 'NONE', #7026, 2.499999999999998668 ) ;
#16907=DIRECTION ( 'NONE',  ( 0.000000000000000000, 0.000000000000000000, -1.000000000000000000 ) ) ;
#16908=ORIENTED_EDGE ( 'NONE', *, *, #20055, .T. ) ;
#16909=VERTEX_POINT ( 'NONE', #2617 ) ;
#16910=B_SPLINE_CURVE_WITH_KNOTS ( 'NONE', 3,
 ( #5797, #12770, #19783, #4086, #11054, #18043, #16331, #9348, #2814, #10009 ),
 .UNSPECIFIED., .F., .F.,
 ( 4, 2, 2, 2, 4 ),
 ( 5.485454109350892508E-19, 0.002975785561748033829, 0.005951571123496067657, 0.008927356685244100185, 0.01190314224699213705 ),
 .UNSPECIFIED. ) ;
#16912=CARTESIAN_POINT ( 'NONE',  ( -19.98510692294888713, 21.15566478733060762, 58.14357129518347733 ) ) ;
#16913=CARTESIAN_POINT ( 'NONE',  ( 12.99999999999993960, 42.51666049839543149, -100.0000000000000000 ) ) ;
#16919=ADVANCED_FACE ( 'NONE', ( #16694, #4560 ), #11539, .F. ) ;
#16922=FACE_OUTER_BOUND ( 'NONE', #521, .T. ) ;
#16924=DIRECTION ( 'NONE',  ( -0.000000000000000000, 1.000000000000000000, -0.000000000000000000 ) ) ;
#16925=ORIENTED_EDGE ( 'NONE', *, *, #10715, .F. ) ;
#16929=ORIENTED_EDGE ( 'NONE', *, *, #22522, .F. ) ;
#16931=DIRECTION ( 'NONE',  ( 0.000000000000000000, 1.000000000000000000, 0.000000000000000000 ) ) ;
#16938=ADVANCED_FACE ( 'NONE', ( #7484 ), #1879, .F. ) ;
#16939=DIRECTION ( 'NONE',  ( 0.000000000000000000, 0.000000000000000000, -1.000000000000000000 ) ) ;
#16942=CARTESIAN_POINT ( 'NONE',  ( -1.054992083788969470, 34.97194892666163213, -38.77590480714997767 ) ) ;
#16943=FACE_OUTER_BOUND ( 'NONE', #10184, .T. ) ;
#16944=CARTESIAN_POINT ( 'NONE',  ( -17.83677152930542675, 10.91058841726865403, -60.06362461869091618 ) ) ;
#16947=CARTESIAN_POINT ( 'NONE',  ( 14.17374118098243763, 24.92453540474833673, 45.45638825402599537 ) ) ;
#16954=FACE_OUTER_BOUND ( 'NONE', #47, .T. ) ;
#16959=ORIENTED_EDGE ( 'NONE', *, *, #12120, .F. ) ;
#16964=CARTESIAN_POINT ( 'NONE',  ( 9.327259721468506015, -2.742977016014770175, 53.40697688051272962 ) ) ;
#16967=LINE ( 'NONE', #20638, #690 ) ;
#16968=ORIENTED_EDGE ( 'NONE', *, *, #21678, .F. ) ;
#16969=DIRECTION ( 'NONE',  ( 0.000000000000000000, 0.000000000000000000, 1.000000000000000000 ) ) ;
#16973=CARTESIAN_POINT ( 'NONE',  ( 6.041077103370438905, -0.8288449397156273379, -52.13906252460637347 ) ) ;
#16975=CIRCLE ( 'NONE', #18065, 2.000000000000002665 ) ;
#16976=CARTESIAN_POINT ( 'NONE',  ( 6.631891271510764518, 39.71688159335408130, 53.15285333858339101 ) ) ;
#16978=CARTESIAN_POINT ( 'NONE',  ( -90.00000000000000000, 40.00000000000000711, -9.108981535246192915E-16 ) ) ;
#16988=CARTESIAN_POINT ( 'NONE',  ( 19.48215071167051704, 15.15508441932860606, -58.00945324419101468 ) ) ;
#16989=ORIENTED_EDGE ( 'NONE', *, *, #15752, .T. ) ;
#16990=ORIENTED_EDGE ( 'NONE', *, *, #9652, .T. ) ;
#16992=ORIENTED_EDGE ( 'NONE', *, *, #13764, .T. ) ;
#16993=DIRECTION ( 'NONE',  ( 1.000000000000000000, 0.000000000000000000, 0.000000000000000000 ) ) ;
#16994=VERTEX_POINT ( 'NONE', #3497 ) ;
#16999=DIRECTION ( 'NONE',  ( 0.000000000000000000, 0.000000000000000000, 1.000000000000000000 ) ) ;
#17000=CARTESIAN_POINT ( 'NONE',  ( -7.480086125713259371, -0.2526605362823695633, -53.02285530597750807 ) ) ;
#17003=EDGE_CURVE ( 'NONE', #4421, #21115, #21161, .T. ) ;
#17004=ORIENTED_EDGE ( 'NONE', *, *, #3060, .F. ) ;
#17006=CARTESIAN_POINT ( 'NONE',  ( 35.00000000000000000, -9.000000000000001776, -13.99999999999999645 ) ) ;
#17007=CARTESIAN_POINT ( 'NONE',  ( -5.450915183833553575E-14, -3.671184582167058341, -46.55282949880530907 ) ) ;
#17008=DIRECTION ( 'NONE',  ( 0.000000000000000000, 0.000000000000000000, -1.000000000000000000 ) ) ;
#17009=VECTOR ( 'NONE', #16484, 1000.000000000000000 ) ;
#17012=CONICAL_SURFACE ( 'NONE', #6783, 49.99999999999998579, 0.7853981633974691512 ) ;
#17013=CARTESIAN_POINT ( 'NONE',  ( -10.38220159744133042, 9.149172668433816824, 43.52345836121337896 ) ) ;
#17014=VERTEX_POINT ( 'NONE', #19306 ) ;
#17016=EDGE_CURVE ( 'NONE', #1538, #14638, #2579, .T. ) ;
#17017=ORIENTED_EDGE ( 'NONE', *, *, #3728, .T. ) ;
#17020=CARTESIAN_POINT ( 'NONE',  ( -22.20813536596353188, 23.24072130216429599, 58.62062866457846866 ) ) ;
#17023=DIRECTION ( 'NONE',  ( 0.000000000000000000, 0.000000000000000000, -1.000000000000000000 ) ) ;
#17024=CARTESIAN_POINT ( 'NONE',  ( -26.00000000000001421, 19.99999999999982947, -105.0010000000000048 ) ) ;
#17025=AXIS2_PLACEMENT_3D ( 'NONE', #18412, #12901, #16701 ) ;
#17028=CARTESIAN_POINT ( 'NONE',  ( -15.00000000000001421, 20.00000000000000355, 45.82575694955841072 ) ) ;
#17029=DIRECTION ( 'NONE',  ( 0.000000000000000000, 0.000000000000000000, -1.000000000000000000 ) ) ;
#17031=CARTESIAN_POINT ( 'NONE',  ( 11.15511648636531739, 39.11609166919075165, -55.07420106209022492 ) ) ;
#17043=B_SPLINE_CURVE_WITH_KNOTS ( 'NONE', 3,
 ( #4286, #13411, #18477, #5992, #14688, #16644, #11257, #834, #22036, #6226, #949, #9436, #7714, #18255, #13185, #2566, #20434, #11490, #4625, #9547 ),
 .UNSPECIFIED., .F., .F.,
 ( 4, 2, 2, 2, 2, 2, 2, 2, 2, 4 ),
 ( 0.02328883130680912614, 0.02567687977621935236, 0.02687090401092445680, 0.02806492824562956817, 0.03284102518444999980, 0.03522907365386021561, 0.03761712212327043836, 0.03881114635797554280, 0.04000517059268065417, 0.04239321906209086999 ),
 .UNSPECIFIED. ) ;
#17044=AXIS2_PLACEMENT_3D ( 'NONE', #12009, #6622, #9940 ) ;
#17047=CARTESIAN_POINT ( 'NONE',  ( 0.05615509895247599442, -4.650464140362338128, 45.38761122811000348 ) ) ;
#17049=DIRECTION ( 'NONE',  ( -0.000000000000000000, -1.000000000000000000, -0.000000000000000000 ) ) ;
#17050=AXIS2_PLACEMENT_3D ( 'NONE', #2885, #20744, #15107 ) ;
#17051=CIRCLE ( 'NONE', #6830, 2.500000000000002220 ) ;
#17052=AXIS2_PLACEMENT_3D ( 'NONE', #5511, #8733, #3586 ) ;
#17053=ORIENTED_EDGE ( 'NONE', *, *, #22158, .T. ) ;
#17054=CARTESIAN_POINT ( 'NONE',  ( 13.25963002225072884, 12.97669314386523176, 45.02656532858659943 ) ) ;
#17055=CARTESIAN_POINT ( 'NONE',  ( -4.076028284552909220, 34.44346285612737546, -39.58813741008486886 ) ) ;
#17056=CARTESIAN_POINT ( 'NONE',  ( 35.00000000000000000, 2.142135623730931471, -49.99999999999999289 ) ) ;
#17057=CARTESIAN_POINT ( 'NONE',  ( -18.82278182890058460, 26.77493817624126038, -60.32982055024027801 ) ) ;
#17058=CARTESIAN_POINT ( 'NONE',  ( -4.198142121831033968, 39.89210073658759370, 51.71386687473788868 ) ) ;
#17060=ORIENTED_EDGE ( 'NONE', *, *, #6366, .F. ) ;
#17061=CARTESIAN_POINT ( 'NONE',  ( 11.84374239103369497, 29.21200678190359667, 44.31542800769556578 ) ) ;
#17063=CARTESIAN_POINT ( 'NONE',  ( 11.00126833636921830, 3.276569432483688704, -57.62199738645433200 ) ) ;
#17065=VERTEX_POINT ( 'NONE', #16642 ) ;
#17066=CARTESIAN_POINT ( 'NONE',  ( 5.249999999999981348, 40.00000000000000000, 41.42387596543812123 ) ) ;
#17071=ORIENTED_EDGE ( 'NONE', *, *, #2211, .T. ) ;
#17073=ORIENTED_EDGE ( 'NONE', *, *, #21981, .T. ) ;
#17074=DIRECTION ( 'NONE',  ( 0.000000000000000000, 0.000000000000000000, 1.000000000000000000 ) ) ;
#17077=CARTESIAN_POINT ( 'NONE',  ( 16.07406985629799578, 8.092854060485286993, 59.53272467997607720 ) ) ;
#17080=ORIENTED_EDGE ( 'NONE', *, *, #3080, .F. ) ;
#17083=ORIENTED_EDGE ( 'NONE', *, *, #21587, .F. ) ;
#17086=EDGE_CURVE ( 'NONE', #10900, #18746, #1070, .T. ) ;
#17087=CARTESIAN_POINT ( 'NONE',  ( 7.577104390338814888, -0.4826542685309015424, -53.01683071947938686 ) ) ;
#17089=CARTESIAN_POINT ( 'NONE',  ( 4.196817044553720066, 39.89217751381926291, 51.71303682859505102 ) ) ;
#17091=CARTESIAN_POINT ( 'NONE',  ( 13.08927703801863807, 27.36553638769442998, -44.94509734929665967 ) ) ;
#17092=ORIENTED_EDGE ( 'NONE', *, *, #5691, .T. ) ;
#17093=DIRECTION ( 'NONE',  ( -0.000000000000000000, -0.000000000000000000, -1.000000000000000000 ) ) ;
#17094=CARTESIAN_POINT ( 'NONE',  ( -22.42598460344824218, 19.26775710289567201, 58.66769746720327561 ) ) ;
#17095=VERTEX_POINT ( 'NONE', #4167 ) ;
#17096=CARTESIAN_POINT ( 'NONE',  ( 5.833333333333329485, 40.00000000000000000, -40.61164310337066041 ) ) ;
#17097=ADVANCED_FACE ( 'NONE', ( #2565 ), #14796, .F. ) ;
#17100=VECTOR ( 'NONE', #9877, 1000.000000000000000 ) ;
#17101=CARTESIAN_POINT ( 'NONE',  ( 20.32373648405300770, 10.46972314276608884, -58.17772014969877148 ) ) ;
#17103=ORIENTED_EDGE ( 'NONE', *, *, #8149, .F. ) ;
#17108=DIRECTION ( 'NONE',  ( 0.000000000000000000, 0.000000000000000000, -1.000000000000000000 ) ) ;
#17109=DIRECTION ( 'NONE',  ( 1.000000000000000000, 0.000000000000000000, 0.000000000000000000 ) ) ;
#17114=ORIENTED_EDGE ( 'NONE', *, *, #1151, .T. ) ;
#17116=ORIENTED_EDGE ( 'NONE', *, *, #2880, .T. ) ;
#17119=CARTESIAN_POINT ( 'NONE',  ( 42.50000000000000711, -12.00000000000000000, 54.00000000000000711 ) ) ;
#17121=CIRCLE ( 'NONE', #21155, 2.499999999999998668 ) ;
#17124=CARTESIAN_POINT ( 'NONE',  ( 7.505578006075174891, 1.461761173328240071, -55.63523492904086254 ) ) ;
#17125=CIRCLE ( 'NONE', #7983, 2.099999999999997868 ) ;
#17127=CIRCLE ( 'NONE', #1409, 49.99999999999998579 ) ;
#17131=EDGE_LOOP ( 'NONE', ( #19933, #4255, #10024 ) ) ;
#17136=CARTESIAN_POINT ( 'NONE',  ( 2.232799048558932853, 39.96997190553584289, -50.39091384480168756 ) ) ;
#17137=CARTESIAN_POINT ( 'NONE',  ( -17.38288706075493906, 10.07729229769342538, -59.93358289200955369 ) ) ;
#17140=EDGE_CURVE ( 'NONE', #16507, #5122, #16681, .T. ) ;
#17143=CARTESIAN_POINT ( 'NONE',  ( -8.743619476591407036, 40.00000000000000000, -53.24632774931270518 ) ) ;
#17146=DIRECTION ( 'NONE',  ( -1.000000000000000000, 0.000000000000000000, -0.000000000000000000 ) ) ;
#17147=ORIENTED_EDGE ( 'NONE', *, *, #903, .F. ) ;
#17148=EDGE_CURVE ( 'NONE', #20269, #10746, #3884, .T. ) ;
#17154=DIRECTION ( 'NONE',  ( 1.000000000000000000, 0.000000000000000000, 0.000000000000000000 ) ) ;
#17158=AXIS2_PLACEMENT_3D ( 'NONE', #4431, #17008, #4660 ) ;
#17159=AXIS2_PLACEMENT_3D ( 'NONE', #11025, #5763, #14682 ) ;
#17160=ORIENTED_EDGE ( 'NONE', *, *, #18855, .T. ) ;
#17161=FACE_OUTER_BOUND ( 'NONE', #16013, .T. ) ;
#17165=CARTESIAN_POINT ( 'NONE',  ( 8.199064559763613147, 7.360541284256825634, 42.22991907770642683 ) ) ;
#17166=CARTESIAN_POINT ( 'NONE',  ( -3.601266574137734100, 34.57013445913566585, -39.39030536259064519 ) ) ;
#17168=CARTESIAN_POINT ( 'NONE',  ( -21.72501817863217966, 25.59362490671916746, -58.51313831023544765 ) ) ;
#17169=EDGE_CURVE ( 'NONE', #4759, #21174, #369, .T. ) ;
#17170=DIRECTION ( 'NONE',  ( 1.000000000000000000, 0.000000000000000000, 0.000000000000000000 ) ) ;
#17171=CARTESIAN_POINT ( 'NONE',  ( -13.10473755708775201, 38.28578281281269113, 55.88243319223045091 ) ) ;
#17174=CARTESIAN_POINT ( 'NONE',  ( 14.92530643917652711, 21.54450079162174703, 45.79309713780077118 ) ) ;
#17175=CARTESIAN_POINT ( 'NONE',  ( -1.387778780781445518E-14, 20.00000000000000355, 105.0000000000000142 ) ) ;
#17178=CYLINDRICAL_SURFACE ( 'NONE', #7804, 2.500000000000002220 ) ;
#17179=VERTEX_POINT ( 'NONE', #15018 ) ;
#17181=ADVANCED_FACE ( 'NONE', ( #1282, #12053 ), #20317, .F. ) ;
#17185=VERTEX_POINT ( 'NONE', #11931 ) ;
#17189=DIRECTION ( 'NONE',  ( 0.000000000000000000, -1.000000000000000000, 0.000000000000000000 ) ) ;
#17190=CARTESIAN_POINT ( 'NONE',  ( -0.6864184775319864817, -1.216838870810144080, 47.75834167804403307 ) ) ;
#17194=ORIENTED_EDGE ( 'NONE', *, *, #15397, .T. ) ;
#17195=CARTESIAN_POINT ( 'NONE',  ( -35.00000000000000000, -9.000000000000001776, 1.387778780781445676E-14 ) ) ;
#17196=DIRECTION ( 'NONE',  ( 0.000000000000000000, 0.000000000000000000, 1.000000000000000000 ) ) ;
#17197=ORIENTED_EDGE ( 'NONE', *, *, #10353, .T. ) ;
#17202=CARTESIAN_POINT ( 'NONE',  ( 9.506747383188477230, 40.00000000000000711, 53.50938557514125193 ) ) ;
#17204=CARTESIAN_POINT ( 'NONE',  ( 12.06668108811418705, 28.91809087000033784, -44.43106897542662637 ) ) ;
#17206=CARTESIAN_POINT ( 'NONE',  ( 1.243967489023766193, -3.588031564569214659E-15, -51.43875557960451061 ) ) ;
#17220=EDGE_LOOP ( 'NONE', ( #14722, #8482, #140, #558 ) ) ;
#17222=CARTESIAN_POINT ( 'NONE',  ( 14.71244060472245252, 36.96434927850640406, 56.47085971327723541 ) ) ;
#17227=CARTESIAN_POINT ( 'NONE',  ( 1.564319729173993423, -1.162775034690379128, -47.08282483555583298 ) ) ;
#17228=EDGE_LOOP ( 'NONE', ( #5235, #19522, #8955, #9281 ) ) ;
#17229=CARTESIAN_POINT ( 'NONE',  ( -6.093892532912075666, 0.8902119804445677298, 54.73806350723837966 ) ) ;
#17234=CARTESIAN_POINT ( 'NONE',  ( -0.5261157918504695274, 39.99836265446453609, 49.13909455355741329 ) ) ;
#17238=ORIENTED_EDGE ( 'NONE', *, *, #1765, .T. ) ;
#17239=CIRCLE ( 'NONE', #20924, 18.00000000000000355 ) ;
#17241=PRODUCT_DEFINITION ( 'UNKNOWN', '', #21568, #409 ) ;
#17245=VERTEX_POINT ( 'NONE', #22380 ) ;
#17246=DIRECTION ( 'NONE',  ( 0.000000000000000000, 0.000000000000000000, 1.000000000000000000 ) ) ;
#17248=CARTESIAN_POINT ( 'NONE',  ( -11.86180952234344588, 38.99999999999292299, 55.35904751185378103 ) ) ;
#17250=CARTESIAN_POINT ( 'NONE',  ( -12.92329681834244681, 4.659497110088497429, -58.43073491095716321 ) ) ;
#17251=CARTESIAN_POINT ( 'NONE',  ( 0.2640866558584379353, 39.99958921855358795, 48.93844575723053936 ) ) ;
#17252=EDGE_LOOP ( 'NONE', ( #4079, #3053, #12398, #19917 ) ) ;
#17253=FACE_OUTER_BOUND ( 'NONE', #20361, .T. ) ;
#17254=CARTESIAN_POINT ( 'NONE',  ( -9.100109617798446848, 40.00000000000000000, -53.37249913072469099 ) ) ;
#17264=CARTESIAN_POINT ( 'NONE',  ( 34.99999999999980815, 40.00000000000000711, 54.99999999999922551 ) ) ;
#17266=EDGE_CURVE ( 'NONE', #9068, #105, #9009, .T. ) ;
#17267=ORIENTED_EDGE ( 'NONE', *, *, #356, .F. ) ;
#17269=CARTESIAN_POINT ( 'NONE',  ( 9.079900084793775861, 0.2952492082908232396, -53.92155889450892658 ) ) ;
#17271=DIRECTION ( 'NONE',  ( 1.000000000000000000, 0.000000000000000000, -1.224646799147353207E-16 ) ) ;
#17273=CARTESIAN_POINT ( 'NONE',  ( 10.38193264731104115, 9.167449762519604306, 43.52061562521062399 ) ) ;
#17276=CARTESIAN_POINT ( 'NONE',  ( -21.77460018174987155, 14.53841458819381316, -58.52494103856261631 ) ) ;
#17278=ADVANCED_FACE ( 'NONE', ( #8941 ), #19160, .T. ) ;
#17279=VERTEX_POINT ( 'NONE', #21101 ) ;
#17281=DIRECTION ( 'NONE',  ( 0.000000000000000000, 0.000000000000000000, 1.000000000000000000 ) ) ;
#17282=CARTESIAN_POINT ( 'NONE',  ( -42.50000000000000711, -12.00000000000012434, 44.97499999999989484 ) ) ;
#17288=DIRECTION ( 'NONE',  ( 0.000000000000000000, -1.000000000000000000, 0.000000000000000000 ) ) ;
#17289=LINE ( 'NONE', #22472, #16408 ) ;
#17290=EDGE_CURVE ( 'NONE', #10462, #17245, #20727, .T. ) ;
#17298=CYLINDRICAL_SURFACE ( 'NONE', #21277, 6.499999999999999112 ) ;
#17305=CARTESIAN_POINT ( 'NONE',  ( -11.86180952234070674, 38.99999999999457145, 55.35904751185264416 ) ) ;
#17307=DIRECTION ( 'NONE',  ( -0.000000000000000000, -0.000000000000000000, -1.000000000000000000 ) ) ;
#17308=AXIS2_PLACEMENT_3D ( 'NONE', #15374, #10437, #6681 ) ;
#17310=CARTESIAN_POINT ( 'NONE',  ( -9.165151389911724067, 39.99999999999999289, -56.36098470834080132 ) ) ;
#17311=CARTESIAN_POINT ( 'NONE',  ( 3.019668934335359545, 39.94555832490831193, 50.93804378708211544 ) ) ;
#17312=CARTESIAN_POINT ( 'NONE',  ( 8.188149873056865147, 32.58630821608367256, -42.20917188641860207 ) ) ;
#17313=ORIENTED_EDGE ( 'NONE', *, *, #17534, .F. ) ;
#17314=CARTESIAN_POINT ( 'NONE',  ( 6.696867368503558448E-15, 40.00000000000000000, 48.73397172404481381 ) ) ;
#17317=FACE_OUTER_BOUND ( 'NONE', #16762, .T. ) ;
#17319=LINE ( 'NONE', #8617, #21056 ) ;
#17321=AXIS2_PLACEMENT_3D ( 'NONE', #3971, #5456, #18040 ) ;
#17323=AXIS2_PLACEMENT_3D ( 'NONE', #2765, #1042, #16734 ) ;
#17325=ORIENTED_EDGE ( 'NONE', *, *, #7936, .F. ) ;
#17326=EDGE_CURVE ( 'NONE', #15060, #13151, #5248, .T. ) ;
#17332=EDGE_LOOP ( 'NONE', ( #18765, #11334, #19055, #9898 ) ) ;
#17334=CARTESIAN_POINT ( 'NONE',  ( 19.90501858586606332, 9.588439829449720619, 58.07150046051953041 ) ) ;
#17335=AXIS2_PLACEMENT_3D ( 'NONE', #10713, #17608, #307 ) ;
#17336=CYLINDRICAL_SURFACE ( 'NONE', #21267, 2.499999999999995115 ) ;
#17337=CARTESIAN_POINT ( 'NONE',  ( 5.345263474800246328, 40.00000000000000711, 51.78208639683223424 ) ) ;
#17340=DIRECTION ( 'NONE',  ( 0.000000000000000000, 0.000000000000000000, 1.000000000000000000 ) ) ;
#17341=CARTESIAN_POINT ( 'NONE',  ( -5.833333333333327708, 6.180730040185831164, 40.61164310337068173 ) ) ;
#17342=ORIENTED_EDGE ( 'NONE', *, *, #14281, .F. ) ;
#17349=CARTESIAN_POINT ( 'NONE',  ( -1.080479714573465255, 39.99305457876869951, 49.55623352467100773 ) ) ;
#17351=CARTESIAN_POINT ( 'NONE',  ( 16.71858216490069893, 8.984148545337202307, 57.18548413420058552 ) ) ;
#17353=CARTESIAN_POINT ( 'NONE',  ( 12.99999999999993960, 42.51666049839543149, 105.0000000000000142 ) ) ;
#17357=ORIENTED_EDGE ( 'NONE', *, *, #21284, .F. ) ;
#17359=ORIENTED_EDGE ( 'NONE', *, *, #12635, .T. ) ;
#17360=DIRECTION ( 'NONE',  ( 0.000000000000000000, 0.000000000000000000, 1.000000000000000000 ) ) ;
#17363=CARTESIAN_POINT ( 'NONE',  ( 0.6551139140931220295, 39.99751804686117396, 49.23721919104350775 ) ) ;
#17366=CARTESIAN_POINT ( 'NONE',  ( -5.967611715581248255, 40.00000000000000711, -52.07955728799370831 ) ) ;
#17367=DIRECTION ( 'NONE',  ( -0.000000000000000000, -0.000000000000000000, 1.000000000000000000 ) ) ;
#17377=CYLINDRICAL_SURFACE ( 'NONE', #8557, 49.99999999999998579 ) ;
#17378=CARTESIAN_POINT ( 'NONE',  ( -1.387778780781445518E-14, 20.00000000000000355, -102.0000000000000142 ) ) ;
#17380=ORIENTED_EDGE ( 'NONE', *, *, #6689, .F. ) ;
#17383=AXIS2_PLACEMENT_3D ( 'NONE', #5401, #12382, #15809 ) ;
#17384=DIRECTION ( 'NONE',  ( 0.000000000000000000, 0.000000000000000000, 1.000000000000000000 ) ) ;
#17385=EDGE_CURVE ( 'NONE', #10749, #19781, #4251, .T. ) ;
#17389=CARTESIAN_POINT ( 'NONE',  ( -42.50000000000000711, -5.000000000000000000, 49.60000000000000853 ) ) ;
#17390=CARTESIAN_POINT ( 'NONE',  ( 90.00000000000000000, 28.00000000000000000, -2.099999999999991651 ) ) ;
#17392=EDGE_CURVE ( 'NONE', #8509, #10027, #14822, .T. ) ;
#17393=CARTESIAN_POINT ( 'NONE',  ( -18.14075711706056993, 28.59859666634928743, -57.62969612438654110 ) ) ;
#17398=CARTESIAN_POINT ( 'NONE',  ( 17.00000000000000000, 20.00000000000000711, -102.0000000000000142 ) ) ;
#17400=CARTESIAN_POINT ( 'NONE',  ( -7.505578006075205089, 1.461761173328240515, 55.63523492904089096 ) ) ;
#17405=LINE ( 'NONE', #10628, #14091 ) ;
#17407=VERTEX_POINT ( 'NONE', #7454 ) ;
#17408=EDGE_CURVE ( 'NONE', #14094, #2582, #19733, .T. ) ;
#17412=CIRCLE ( 'NONE', #13381, 2.500000000000002220 ) ;
#17415=DIRECTION ( 'NONE',  ( 0.000000000000000000, 0.5150380749100562650, 0.8571673007021111124 ) ) ;
#17418=DIRECTION ( 'NONE',  ( 0.000000000000000000, -0.7071067811865352493, -0.7071067811865597852 ) ) ;
#17422=CARTESIAN_POINT ( 'NONE',  ( 35.00000000000000000, 38.99999999999999289, 4.258610482196280173E-15 ) ) ;
#17423=ADVANCED_FACE ( 'NONE', ( #13040 ), #5264, .T. ) ;
#17424=CARTESIAN_POINT ( 'NONE',  ( 21.07599011712227011, 12.09199673218656024, -58.36745205258138469 ) ) ;
#17425=LINE ( 'NONE', #8728, #10049 ) ;
#17427=CARTESIAN_POINT ( 'NONE',  ( -3.019669046279628510, 39.94555832068629542, -50.93804386297323106 ) ) ;
#17430=CARTESIAN_POINT ( 'NONE',  ( -20.15166188517206791, 29.89072699358926499, 58.13409936646347376 ) ) ;
#17431=VECTOR ( 'NONE', #6571, 1000.000000000000000 ) ;
#17432=ORIENTED_EDGE ( 'NONE', *, *, #12013, .F. ) ;
#17433=FACE_OUTER_BOUND ( 'NONE', #16221, .T. ) ;
#17435=ADVANCED_FACE ( 'NONE', ( #1143 ), #2026, .F. ) ;
#17436=LINE ( 'NONE', #10106, #10710 ) ;
#17439=ORIENTED_EDGE ( 'NONE', *, *, #18959, .F. ) ;
#17440=ORIENTED_EDGE ( 'NONE', *, *, #20711, .T. ) ;
#17444=CIRCLE ( 'NONE', #12313, 2.099999999999997868 ) ;
#17445=ORIENTED_EDGE ( 'NONE', *, *, #14778, .T. ) ;
#17447=CARTESIAN_POINT ( 'NONE',  ( 16.62266455332486714, 35.11598757108757951, 57.12012504743141506 ) ) ;
#17449=CARTESIAN_POINT ( 'NONE',  ( 8.448970453231776645, 40.00000000000000000, 53.13698759631014923 ) ) ;
#17452=CARTESIAN_POINT ( 'NONE',  ( -4.078319513017746090, 5.557204472854577304, 39.58919430873140755 ) ) ;
#17453=ORIENTED_EDGE ( 'NONE', *, *, #14623, .F. ) ;
#17456=EDGE_LOOP ( 'NONE', ( #6440, #10575 ) ) ;
#17460=CARTESIAN_POINT ( 'NONE',  ( -5.302679949206207333, 39.28774282260670248, 54.25155191766013019 ) ) ;
#17462=EDGE_CURVE ( 'NONE', #14484, #21816, #11572, .T. ) ;
#17465=CARTESIAN_POINT ( 'NONE',  ( 22.05221796475640161, 24.18157222985895061, 58.58672997743932598 ) ) ;
#17466=DIRECTION ( 'NONE',  ( 0.000000000000000000, 1.000000000000000000, 0.000000000000000000 ) ) ;
#17469=ADVANCED_FACE ( 'NONE', ( #5044 ), #9738, .F. ) ;
#17470=B_SPLINE_CURVE_WITH_KNOTS ( 'NONE', 3,
 ( #13865, #8725, #8494, #3466, #20879, #10424, #20986, #17543, #15468, #5183 ),
 .UNSPECIFIED., .F., .F.,
 ( 4, 2, 2, 2, 4 ),
 ( 1.181610135877042463E-17, 0.002975785561748149188, 0.005951571123496287100, 0.008927356685244424578, 0.01190314224699256206 ),
 .UNSPECIFIED. ) ;
#17474=ORIENTED_EDGE ( 'NONE', *, *, #11126, .F. ) ;
#17475=ORIENTED_EDGE ( 'NONE', *, *, #10054, .T. ) ;
#17476=DIRECTION ( 'NONE',  ( 0.000000000000000000, 0.000000000000000000, -1.000000000000000000 ) ) ;
#17477=DIRECTION ( 'NONE',  ( 0.000000000000000000, 0.000000000000000000, -1.000000000000000000 ) ) ;
#17478=AXIS2_PLACEMENT_3D ( 'NONE', #13157, #2532, #4706 ) ;
#17482=CARTESIAN_POINT ( 'NONE',  ( 0.05877019086828588756, 39.99997968727448949, 48.77966970436191474 ) ) ;
#17483=CIRCLE ( 'NONE', #276, 10.00000000000000178 ) ;
#17484=ORIENTED_EDGE ( 'NONE', *, *, #18258, .F. ) ;
#17486=DIRECTION ( 'NONE',  ( 0.000000000000000000, 1.000000000000000000, 0.000000000000000000 ) ) ;
#17487=DIRECTION ( 'NONE',  ( 0.7752116086454784449, 0.5577761202038514776, -0.2965345874457622211 ) ) ;
#17488=FACE_OUTER_BOUND ( 'NONE', #13768, .T. ) ;
#17493=CARTESIAN_POINT ( 'NONE',  ( -19.62614308895802750, 23.87978888144413858, 60.53224704373671727 ) ) ;
#17495=AXIS2_PLACEMENT_3D ( 'NONE', #16698, #15071, #13349 ) ;
#17496=CARTESIAN_POINT ( 'NONE',  ( -8.957612896613865061, 39.56965375125236051, 54.21301076066360736 ) ) ;
#17499=AXIS2_PLACEMENT_3D ( 'NONE', #17603, #17711, #5464 ) ;
#17501=VECTOR ( 'NONE', #18130, 1000.000000000000000 ) ;
#17503=ORIENTED_EDGE ( 'NONE', *, *, #785, .F. ) ;
#17504=EDGE_CURVE ( 'NONE', #16050, #6428, #13340, .T. ) ;
#17506=CARTESIAN_POINT ( 'NONE',  ( 90.00000000000000000, 39.97500000000000142, -9.108981535246192915E-16 ) ) ;
#17507=CIRCLE ( 'NONE', #10543, 9.000000000000003553 ) ;
#17511=EDGE_CURVE ( 'NONE', #1471, #22647, #4591, .T. ) ;
#17515=CARTESIAN_POINT ( 'NONE',  ( -9.998533603140344894, 40.00000000000000000, -54.54288842742649734 ) ) ;
#17520=DIRECTION ( 'NONE',  ( 0.000000000000000000, 0.000000000000000000, -1.000000000000000000 ) ) ;
#17522=CYLINDRICAL_SURFACE ( 'NONE', #19261, 2.099999999999990763 ) ;
#17525=CIRCLE ( 'NONE', #3641, 4.000000000000000000 ) ;
#17526=B_SPLINE_CURVE_WITH_KNOTS ( 'NONE', 3,
 ( #9222, #9461, #14601, #12767, #14480, #5791, #19881, #9118, #3969, #7393, #10939, #4082, #19777 ),
 .UNSPECIFIED., .F., .F.,
 ( 4, 2, 1, 1, 1, 2, 2, 4 ),
 ( 0.000000000000000000, 0.2499999999999938383, 0.3749999999999902300, 0.4374999999999883982, 0.4687499999999868439, 0.4843749999999850675, 0.4999999999999832911, 1.000000000000000000 ),
 .UNSPECIFIED. ) ;
#17528=DIRECTION ( 'NONE',  ( 0.000000000000000000, 0.000000000000000000, 1.000000000000000000 ) ) ;
#17531=ORIENTED_EDGE ( 'NONE', *, *, #7174, .T. ) ;
#17532=EDGE_LOOP ( 'NONE', ( #2934, #14359, #21217 ) ) ;
#17534=EDGE_CURVE ( 'NONE', #10705, #17179, #11003, .T. ) ;
#17542=ORIENTED_EDGE ( 'NONE', *, *, #18574, .T. ) ;
#17543=CARTESIAN_POINT ( 'NONE',  ( 8.479740367039916293, -4.901256658985767345, -50.57596245086818243 ) ) ;
#17544=CARTESIAN_POINT ( 'NONE',  ( 14.68518659845079100, 36.96998281527655195, -56.45735093204005040 ) ) ;
#17546=CARTESIAN_POINT ( 'NONE',  ( -9.728382627765713053, 39.99999999999997868, -53.57939893134117426 ) ) ;
#17548=CARTESIAN_POINT ( 'NONE',  ( -9.952189117650803496, 40.00000000000000000, 53.64426396172073908 ) ) ;
#17549=CARTESIAN_POINT ( 'NONE',  ( -22.15746142094444338, 16.52917608750725975, 58.60949679988863892 ) ) ;
#17554=DIRECTION ( 'NONE',  ( 0.000000000000000000, 0.000000000000000000, -1.000000000000000000 ) ) ;
#17555=CIRCLE ( 'NONE', #15345, 14.00000000000000000 ) ;
#17563=CARTESIAN_POINT ( 'NONE',  ( 19.47136665037375636, 8.793048248091398733, 57.95785196855348431 ) ) ;
#17564=CIRCLE ( 'NONE', #6225, 2.499999999999995115 ) ;
#17565=FACE_OUTER_BOUND ( 'NONE', #16619, .T. ) ;
#17567=ORIENTED_EDGE ( 'NONE', *, *, #4066, .F. ) ;
#17568=DIRECTION ( 'NONE',  ( -0.000000000000000000, 1.000000000000000000, -0.000000000000000000 ) ) ;
#17569=CARTESIAN_POINT ( 'NONE',  ( -4.986731981817630555, 5.845158537422243228, 40.05110651909059527 ) ) ;
#17571=CARTESIAN_POINT ( 'NONE',  ( -4.663248442268214333, 0.4972264943030605400, 53.80945059829245736 ) ) ;
#17572=CARTESIAN_POINT ( 'NONE',  ( -14.71244060472248272, 36.96434927850638985, -56.47085971327719989 ) ) ;
#17573=FACE_OUTER_BOUND ( 'NONE', #12003, .T. ) ;
#17576=FACE_OUTER_BOUND ( 'NONE', #20222, .T. ) ;
#17579=DIRECTION ( 'NONE',  ( -0.000000000000000000, -1.000000000000000000, -0.000000000000000000 ) ) ;
#17580=CARTESIAN_POINT ( 'NONE',  ( -0.6620359884758859614, 39.99747031435470745, 49.24247971419962511 ) ) ;
#17582=CARTESIAN_POINT ( 'NONE',  ( 21.16618710811372139, 27.45243199383212840, 58.38369730662807910 ) ) ;
#17585=CARTESIAN_POINT ( 'NONE',  ( 35.00000000000000000, 40.00000000000000000, 51.00000000000002842 ) ) ;
#17587=EDGE_CURVE ( 'NONE', #14484, #7482, #19128, .T. ) ;
#17588=EDGE_LOOP ( 'NONE', ( #3456, #10344, #3308, #19971, #10228, #2527, #5669, #8260, #18722 ) ) ;
#17597=DIRECTION ( 'NONE',  ( -0.000000000000000000, -0.000000000000000000, 1.000000000000000000 ) ) ;
#17598=CARTESIAN_POINT ( 'NONE',  ( 1.321838024766639252, 39.98984255672822741, 49.73540085867594485 ) ) ;
#17602=DIRECTION ( 'NONE',  ( 0.000000000000000000, 0.000000000000000000, 1.000000000000000000 ) ) ;
#17603=CARTESIAN_POINT ( 'NONE',  ( -42.50000000000000711, -12.00000000000000000, 47.50000000000000711 ) ) ;
#17606=LINE ( 'NONE', #1913, #10960 ) ;
#17608=DIRECTION ( 'NONE',  ( -0.000000000000000000, -0.000000000000000000, 1.000000000000000000 ) ) ;
#17612=ORIENTED_EDGE ( 'NONE', *, *, #17003, .T. ) ;
#17615=CARTESIAN_POINT ( 'NONE',  ( 8.460114887491986480, -4.900635315005658299, -50.56657553898721602 ) ) ;
#17617=CARTESIAN_POINT ( 'NONE',  ( 11.73108507413468971, 40.00000000000000000, -54.23086838360208617 ) ) ;
#17622=CYLINDRICAL_SURFACE ( 'NONE', #15670, 30.00000000000000000 ) ;
#17628=CARTESIAN_POINT ( 'NONE',  ( -35.00000000000000000, -4.928932188134504955, 57.07106781186553235 ) ) ;
#17629=DIRECTION ( 'NONE',  ( -1.000000000000000000, 0.000000000000000000, -0.000000000000000000 ) ) ;
#17630=CARTESIAN_POINT ( 'NONE',  ( 14.99999999999998579, 20.00000000000000355, -45.82575694955836809 ) ) ;
#17634=EDGE_CURVE ( 'NONE', #2582, #15060, #4966, .T. ) ;
#17635=AXIS2_PLACEMENT_3D ( 'NONE', #9740, #9954, #15216 ) ;
#17636=ORIENTED_EDGE ( 'NONE', *, *, #2744, .T. ) ;
#17637=ORIENTED_EDGE ( 'NONE', *, *, #20667, .T. ) ;
#17638=DIRECTION ( 'NONE',  ( 0.000000000000000000, 0.000000000000000000, 1.000000000000000000 ) ) ;
#17640=CARTESIAN_POINT ( 'NONE',  ( -8.916870955515566521, 2.080241304161454252, 56.50845996868352472 ) ) ;
#17643=DIRECTION ( 'NONE',  ( -0.000000000000000000, -1.000000000000000000, -0.000000000000000000 ) ) ;
#17644=CARTESIAN_POINT ( 'NONE',  ( -9.038714882927470384, 40.00000000000001421, 53.35170948314333117 ) ) ;
#17647=CARTESIAN_POINT ( 'NONE',  ( 17.98964431006456977, 6.536084871031931698, -57.54127157382310287 ) ) ;
#17653=CARTESIAN_POINT ( 'NONE',  ( -9.103081159019538404, 0.03030367950604238858, 53.87333532811888404 ) ) ;
#17661=ORIENTED_EDGE ( 'NONE', *, *, #19291, .F. ) ;
#17663=ORIENTED_EDGE ( 'NONE', *, *, #6617, .F. ) ;
#17670=CARTESIAN_POINT ( 'NONE',  ( 4.719078569232699749, 39.99999999999999289, 51.46810808308088525 ) ) ;
#17672=ORIENTED_EDGE ( 'NONE', *, *, #11678, .F. ) ;
#17673=DIRECTION ( 'NONE',  ( -0.000000000000000000, -0.000000000000000000, -1.000000000000000000 ) ) ;
#17674=CARTESIAN_POINT ( 'NONE',  ( -0.6683989176636820906, -3.155640224527792359, -47.80307817979882401 ) ) ;
#17680=CARTESIAN_POINT ( 'NONE',  ( 6.002321937219792680, -0.8366808808196497527, 52.11647083208005427 ) ) ;
#17681=ORIENTED_EDGE ( 'NONE', *, *, #21833, .F. ) ;
#17682=CARTESIAN_POINT ( 'NONE',  ( 0.7060561200947481630, 40.00000000000296296, -49.41654807903094593 ) ) ;
#17683=EDGE_CURVE ( 'NONE', #6172, #4131, #21750, .T. ) ;
#17684=FACE_OUTER_BOUND ( 'NONE', #20925, .T. ) ;
#17687=TOROIDAL_SURFACE ( 'NONE', #497, 18.00000000000000355, 4.000000000000000000 ) ;
#17688=CARTESIAN_POINT ( 'NONE',  ( 19.94270148199750281, 21.57319560958842430, 58.13234078200308375 ) ) ;
#17690=CIRCLE ( 'NONE', #11107, 6.499999999999999112 ) ;
#17695=VERTEX_POINT ( 'NONE', #9380 ) ;
#17699=LINE ( 'NONE', #20930, #13259 ) ;
#17704=DIRECTION ( 'NONE',  ( 0.000000000000000000, 0.000000000000000000, -1.000000000000000000 ) ) ;
#17706=CARTESIAN_POINT ( 'NONE',  ( 4.585174426381384727, 39.86909732867421496, 51.95486263624831480 ) ) ;
#17710=CARTESIAN_POINT ( 'NONE',  ( 13.00000000000024336, -2.516660498395250745, 100.0000000000000000 ) ) ;
#17711=DIRECTION ( 'NONE',  ( -0.000000000000000000, 1.000000000000000000, -0.000000000000000000 ) ) ;
#17714=ADVANCED_FACE ( 'NONE', ( #546 ), #11195, .F. ) ;
#17715=AXIS2_PLACEMENT_3D ( 'NONE', #21103, #8835, #13749 ) ;
#17719=DIRECTION ( 'NONE',  ( 1.000000000000000000, 0.000000000000000000, 0.000000000000000000 ) ) ;
#17721=MANIFOLD_SOLID_BREP ( 'Chamfer3', #7857 ) ;
#17724=ORIENTED_EDGE ( 'NONE', *, *, #12562, .F. ) ;
#17725=EDGE_CURVE ( 'NONE', #11729, #21259, #19104, .T. ) ;
#17726=ORIENTED_EDGE ( 'NONE', *, *, #7371, .T. ) ;
#17727=CARTESIAN_POINT ( 'NONE',  ( 8.523345606290934739, -2.856915207368400988, -52.89411661619065086 ) ) ;
#17730=CONICAL_SURFACE ( 'NONE', #6766, 2.524999999999999467, 0.7853981633974482790 ) ;
#17731=FACE_OUTER_BOUND ( 'NONE', #18591, .T. ) ;
#17734=CARTESIAN_POINT ( 'NONE',  ( -19.42347305479418296, 31.41593231561366650, -57.95407386126544225 ) ) ;
#17741=FACE_BOUND ( 'NONE', #6356, .T. ) ;
#17743=VERTEX_POINT ( 'NONE', #178 ) ;
#17745=AXIS2_PLACEMENT_3D ( 'NONE', #18513, #6483, #6370 ) ;
#17747=DIRECTION ( 'NONE',  ( 0.000000000000000000, 0.000000000000000000, -1.000000000000000000 ) ) ;
#17748=CARTESIAN_POINT ( 'NONE',  ( 13.56354382738798137, 2.142135623730915928, -56.03997097393683902 ) ) ;
#17754=ORIENTED_EDGE ( 'NONE', *, *, #13510, .F. ) ;
#17755=CARTESIAN_POINT ( 'NONE',  ( 0.1964561668385597371, 39.99977788401218959, -48.88630801547629545 ) ) ;
#17757=DIRECTION ( 'NONE',  ( -0.000000000000000000, -1.000000000000000000, -0.000000000000000000 ) ) ;
#17761=CARTESIAN_POINT ( 'NONE',  ( -7.392691288592804000, 39.99999999999999289, 52.71482085253978056 ) ) ;
#17765=CARTESIAN_POINT ( 'NONE',  ( 22.43696576003031851, 20.17999529786815671, -58.67002796852975166 ) ) ;
#17770=CARTESIAN_POINT ( 'NONE',  ( -11.86180952233172725, 39.00000000000000000, -55.35904751184885697 ) ) ;
#17771=CARTESIAN_POINT ( 'NONE',  ( -1.038203980847386187, 39.99359456186276418, -49.52478356376864355 ) ) ;
#17772=EDGE_CURVE ( 'NONE', #4267, #20199, #10701, .T. ) ;
#17776=VECTOR ( 'NONE', #14686, 1000.000000000000000 ) ;
#17786=FACE_OUTER_BOUND ( 'NONE', #7221, .T. ) ;
#17790=ORIENTED_EDGE ( 'NONE', *, *, #4077, .T. ) ;
#17792=DIRECTION ( 'NONE',  ( -0.000000000000000000, -1.000000000000000000, -0.000000000000000000 ) ) ;
#17794=AXIS2_PLACEMENT_3D ( 'NONE', #14078, #22610, #2071 ) ;
#17796=CARTESIAN_POINT ( 'NONE',  ( -1.799800578957587716, 0.06826247860514957078, 51.82705267766674950 ) ) ;
#17798=CARTESIAN_POINT ( 'NONE',  ( -12.23364788621111643, 38.77571842908470501, -55.51446324382121134 ) ) ;
#17799=AXIS2_PLACEMENT_3D ( 'NONE', #6538, #11688, #2989 ) ;
#17803=CARTESIAN_POINT ( 'NONE',  ( 1.061447036142194600, 34.97146889883303800, 38.77662560222201904 ) ) ;
#17808=CARTESIAN_POINT ( 'NONE',  ( 6.263166516349132351, 0.9587459495540682219, 54.84564255054416293 ) ) ;
#17810=CARTESIAN_POINT ( 'NONE',  ( 19.59396665412829464, 15.89499847339836691, 60.52448832957817615 ) ) ;
#17814=EDGE_LOOP ( 'NONE', ( #7768, #9430, #6713, #10934 ) ) ;
#17816=EDGE_CURVE ( 'NONE', #18632, #17095, #1804, .T. ) ;
#17818=CARTESIAN_POINT ( 'NONE',  ( 35.00000000000000000, -5.000000000000000000, 57.00000000000002842 ) ) ;
#17826=CARTESIAN_POINT ( 'NONE',  ( 12.09218358684860917, 1.291952833854519422, -55.42846997241216656 ) ) ;
#17829=CIRCLE ( 'NONE', #22609, 2.099999999999997868 ) ;
#17831=CARTESIAN_POINT ( 'NONE',  ( -35.00000000000058265, 26.00000000000000355, -52.90000000000076597 ) ) ;
#17833=FACE_OUTER_BOUND ( 'NONE', #19377, .T. ) ;
#17836=AXIS2_PLACEMENT_3D ( 'NONE', #4733, #8154, #15008 ) ;
#17837=DIRECTION ( 'NONE',  ( -0.000000000000000000, -0.000000000000000000, 1.000000000000000000 ) ) ;
#17838=EDGE_LOOP ( 'NONE', ( #4424, #7378, #1423, #13538, #536, #3264, #13533, #7450, #418 ) ) ;
#17839=VERTEX_POINT ( 'NONE', #18286 ) ;
#17840=AXIS2_PLACEMENT_3D ( 'NONE', #12710, #16040, #350 ) ;
#17841=EDGE_CURVE ( 'NONE', #12474, #14756, #17525, .T. ) ;
#17842=CIRCLE ( 'NONE', #13060, 57.07106781186551103 ) ;
#17843=ORIENTED_EDGE ( 'NONE', *, *, #21280, .F. ) ;
#17844=CARTESIAN_POINT ( 'NONE',  ( -1.564319729173966111, -1.162775034690410214, -47.08282483555584008 ) ) ;
#17846=DIRECTION ( 'NONE',  ( 0.000000000000000000, -0.000000000000000000, 1.000000000000000000 ) ) ;
#17852=FACE_OUTER_BOUND ( 'NONE', #22404, .T. ) ;
#17854=AXIS2_PLACEMENT_3D ( 'NONE', #3432, #8466, #13851 ) ;
#17855=ORIENTED_EDGE ( 'NONE', *, *, #5392, .T. ) ;
#17856=CARTESIAN_POINT ( 'NONE',  ( 90.00000000000000000, 40.00000000000000000, 2.500000000000001332 ) ) ;
#17859=EDGE_CURVE ( 'NONE', #14794, #10996, #412, .T. ) ;
#17861=CARTESIAN_POINT ( 'NONE',  ( 10.38193264731109977, 9.167449762519654044, -43.52061562521063109 ) ) ;
#17863=VERTEX_POINT ( 'NONE', #7297 ) ;
#17864=ADVANCED_FACE ( 'NONE', ( #18174 ), #21274, .F. ) ;
#17866=CARTESIAN_POINT ( 'NONE',  ( -9.165151389911720514, 40.00000000000000000, 56.36098470834082264 ) ) ;
#17873=EDGE_CURVE ( 'NONE', #6208, #1794, #16191, .T. ) ;
#17874=ORIENTED_EDGE ( 'NONE', *, *, #7254, .T. ) ;
#17876=DIRECTION ( 'NONE',  ( 1.000000000000000000, 0.000000000000000000, 0.000000000000000000 ) ) ;
#17881=FACE_OUTER_BOUND ( 'NONE', #16553, .T. ) ;
#17883=DIRECTION ( 'NONE',  ( -0.000000000000000000, 1.000000000000000000, -0.000000000000000000 ) ) ;
#17888=ORIENTED_EDGE ( 'NONE', *, *, #7381, .T. ) ;
#17889=FACE_OUTER_BOUND ( 'NONE', #582, .T. ) ;
#17892=CARTESIAN_POINT ( 'NONE',  ( -6.501355175172208511, 39.72712728739963239, -53.07780961191252089 ) ) ;
#17898=EDGE_LOOP ( 'NONE', ( #8877, #9516, #20942, #5179 ) ) ;
#17899=ORIENTED_EDGE ( 'NONE', *, *, #3987, .F. ) ;
#17902=ADVANCED_FACE ( 'NONE', ( #2599 ), #4371, .F. ) ;
#17904=DIRECTION ( 'NONE',  ( 8.659560562351929024E-17, -0.7071067811867928210, 0.7071067811863022134 ) ) ;
#17914=CYLINDRICAL_SURFACE ( 'NONE', #7952, 2.500000000000002220 ) ;
#17915=ORIENTED_EDGE ( 'NONE', *, *, #14528, .T. ) ;
#17920=DIRECTION ( 'NONE',  ( 0.000000000000000000, 0.000000000000000000, -1.000000000000000000 ) ) ;
#17923=CARTESIAN_POINT ( 'NONE',  ( 18.14075711706860616, 28.59859666635273001, 57.62969612438692479 ) ) ;
#17925=DIRECTION ( 'NONE',  ( -0.5002637533272176196, 0.000000000000000000, 0.8658730721687590837 ) ) ;
#17929=ORIENTED_EDGE ( 'NONE', *, *, #19340, .F. ) ;
#17948=CARTESIAN_POINT ( 'NONE',  ( -5.204793789172661889, 39.83796802612397414, 52.32473130827783336 ) ) ;
#17950=ORIENTED_EDGE ( 'NONE', *, *, #12040, .F. ) ;
#17955=CARTESIAN_POINT ( 'NONE',  ( 35.00000000000000000, 40.00000000000000000, 4.258610482196280173E-15 ) ) ;
#17956=AXIS2_PLACEMENT_3D ( 'NONE', #4083, #7510, #4193 ) ;
#17957=CARTESIAN_POINT ( 'NONE',  ( -7.882609639814679786E-15, -9.552912840896525389E-26, -50.50395615645409464 ) ) ;
#17959=DIRECTION ( 'NONE',  ( 0.000000000000000000, 1.000000000000000000, 0.000000000000000000 ) ) ;
#17960=EDGE_CURVE ( 'NONE', #7926, #1702, #9914, .T. ) ;
#17963=CARTESIAN_POINT ( 'NONE',  ( -15.62751878812966133, 32.48885827236730961, -59.38785559521993207 ) ) ;
#17967=CYLINDRICAL_SURFACE ( 'NONE', #21202, 2.499999999999998668 ) ;
#17975=CARTESIAN_POINT ( 'NONE',  ( 92.09999999999999432, 28.00000000000000000, -9.108981535246192915E-16 ) ) ;
#17979=AXIS2_PLACEMENT_3D ( 'NONE', #20976, #11701, #18695 ) ;
#17981=FACE_OUTER_BOUND ( 'NONE', #771, .T. ) ;
#17984=DIRECTION ( 'NONE',  ( 1.000000000000000000, 0.000000000000000000, 0.000000000000000000 ) ) ;
#17987=CARTESIAN_POINT ( 'NONE',  ( -7.434571854303535510, 39.99999999999999289, 52.73242012342949181 ) ) ;
#17990=CYLINDRICAL_SURFACE ( 'NONE', #11973, 2.099999999999990763 ) ;
#17991=DIRECTION ( 'NONE',  ( -0.000000000000000000, -0.000000000000000000, 1.000000000000000000 ) ) ;
#17992=DIRECTION ( 'NONE',  ( -0.000000000000000000, -0.000000000000000000, -1.000000000000000000 ) ) ;
#17994=CARTESIAN_POINT ( 'NONE',  ( -35.00000000000000000, 0.000000000000000000, 9.000000000000015987 ) ) ;
#17998=CARTESIAN_POINT ( 'NONE',  ( -6.069328110416789990, 39.76463894057638271, -52.83839008176153840 ) ) ;
#18000=DIRECTION ( 'NONE',  ( 0.000000000000000000, 0.000000000000000000, -1.000000000000000000 ) ) ;
#18001=AXIS2_PLACEMENT_3D ( 'NONE', #12825, #21436, #5509 ) ;
#18002=CARTESIAN_POINT ( 'NONE',  ( -28.50000000000001421, 19.99999999999982947, 100.0000000000000000 ) ) ;
#18005=ORIENTED_EDGE ( 'NONE', *, *, #17326, .T. ) ;
#18006=ORIENTED_EDGE ( 'NONE', *, *, #7110, .F. ) ;
#18007=VERTEX_POINT ( 'NONE', #12309 ) ;
#18008=DIRECTION ( 'NONE',  ( -1.000000000000000000, 0.000000000000000000, 0.000000000000000000 ) ) ;
#18014=ORIENTED_EDGE ( 'NONE', *, *, #21853, .F. ) ;
#18017=EDGE_CURVE ( 'NONE', #17095, #18632, #7306, .T. ) ;
#18018=DIRECTION ( 'NONE',  ( -0.000000000000000000, -0.000000000000000000, 1.000000000000000000 ) ) ;
#18019=EDGE_LOOP ( 'NONE', ( #1796, #7214, #932, #19457 ) ) ;
#18024=CARTESIAN_POINT ( 'NONE',  ( 2.499203666028194437, 0.1468068017377833490, 52.32025702727163008 ) ) ;
#18025=VERTEX_POINT ( 'NONE', #19427 ) ;
#18027=CARTESIAN_POINT ( 'NONE',  ( 9.998533603140316472, 40.00000000000000000, 54.54288842742651156 ) ) ;
#18029=EDGE_CURVE ( 'NONE', #21858, #599, #13144, .T. ) ;
#18036=ORIENTED_EDGE ( 'NONE', *, *, #4663, .F. ) ;
#18038=DIRECTION ( 'NONE',  ( -1.000000000000000000, 0.000000000000000000, 0.000000000000000000 ) ) ;
#18039=LINE ( 'NONE', #4191, #471 ) ;
#18040=DIRECTION ( 'NONE',  ( -1.000000000000000000, 0.000000000000000000, 0.000000000000000000 ) ) ;
#18042=CARTESIAN_POINT ( 'NONE',  ( -11.86180952233172015, 38.99999999999999289, -55.35904751184885697 ) ) ;
#18043=CARTESIAN_POINT ( 'NONE',  ( -5.816608766684270293, -4.770324936805438121, 49.23968220743370949 ) ) ;
#18045=ORIENTED_EDGE ( 'NONE', *, *, #18426, .T. ) ;
#18046=CARTESIAN_POINT ( 'NONE',  ( -11.68090480754633731, 3.765577839755393619, -57.90797000640141334 ) ) ;
#18048=CARTESIAN_POINT ( 'NONE',  ( -42.50000000000000711, -12.00000000000000000, -54.00000000000000000 ) ) ;
#18049=CARTESIAN_POINT ( 'NONE',  ( -42.50000000000000711, -9.600000000000001421, 47.50000000000000711 ) ) ;
#18050=DIRECTION ( 'NONE',  ( 0.000000000000000000, 0.000000000000000000, -1.000000000000000000 ) ) ;
#18052=CARTESIAN_POINT ( 'NONE',  ( 42.50000000000000711, -9.600000000000001421, 50.00000000000000711 ) ) ;
#18056=AXIS2_PLACEMENT_3D ( 'NONE', #16327, #10696, #12426 ) ;
#18057=ORIENTED_EDGE ( 'NONE', *, *, #15554, .F. ) ;
#18058=CONICAL_SURFACE ( 'NONE', #15115, 2.525000000000110489, 0.7853981633971014453 ) ;
#18059=CONICAL_SURFACE ( 'NONE', #18427, 58.99999999999994316, 0.7853981633974725929 ) ;
#18062=CARTESIAN_POINT ( 'NONE',  ( 35.00000000000000000, 0.000000000000000000, 4.258610482196280173E-15 ) ) ;
#18063=CARTESIAN_POINT ( 'NONE',  ( 2.951378045150416796, -1.204966337757524375, -50.23352299313520319 ) ) ;
#18065=AXIS2_PLACEMENT_3D ( 'NONE', #7837, #19993, #17925 ) ;
#18068=CARTESIAN_POINT ( 'NONE',  ( -3.981144761549149980, 39.90683190540670466, -51.58239934697316897 ) ) ;
#18072=CIRCLE ( 'NONE', #13303, 15.00000000000000000 ) ;
#18073=ORIENTED_EDGE ( 'NONE', *, *, #2880, .F. ) ;
#18075=DIRECTION ( 'NONE',  ( 0.000000000000000000, 0.000000000000000000, 1.000000000000000000 ) ) ;
#18078=CARTESIAN_POINT ( 'NONE',  ( -34.99999999999980815, 40.00000000000000000, 54.99999999999922551 ) ) ;
#18079=CIRCLE ( 'NONE', #1249, 2.499999999999995115 ) ;
#18080=ORIENTED_EDGE ( 'NONE', *, *, #4026, .T. ) ;
#18081=CARTESIAN_POINT ( 'NONE',  ( -35.00000000000000000, -5.000000000000000000, 1.387778780781445676E-14 ) ) ;
#18083=CARTESIAN_POINT ( 'NONE',  ( -26.00000000000001421, 19.99999999999982947, 100.0000000000000000 ) ) ;
#18088=VECTOR ( 'NONE', #9720, 1000.000000000000000 ) ;
#18089=DIRECTION ( 'NONE',  ( 0.000000000000000000, 0.000000000000000000, 1.000000000000000000 ) ) ;
#18091=CARTESIAN_POINT ( 'NONE',  ( 7.364743364090521105, 39.99999999999998579, -52.70305476081712470 ) ) ;
#18092=EDGE_CURVE ( 'NONE', #8965, #16, #2165, .T. ) ;
#18096=CARTESIAN_POINT ( 'NONE',  ( -35.00000000000000000, 39.00000000000000711, 1.387778780781445676E-14 ) ) ;
#18097=VERTEX_POINT ( 'NONE', #10800 ) ;
#18102=CARTESIAN_POINT ( 'NONE',  ( -8.410506002219646504, 40.00000000000000711, 53.12343481204283080 ) ) ;
#18103=ADVANCED_FACE ( 'NONE', ( #12138 ), #10622, .F. ) ;
#18106=DIRECTION ( 'NONE',  ( 1.000000000000000000, 0.000000000000000000, 0.000000000000000000 ) ) ;
#18109=CARTESIAN_POINT ( 'NONE',  ( -2.213007560440093169, 39.97050982720588763, -50.37695298629697049 ) ) ;
#18110=VECTOR ( 'NONE', #5826, 1000.000000000000000 ) ;
#18111=ORIENTED_EDGE ( 'NONE', *, *, #3252, .F. ) ;
#18112=DIRECTION ( 'NONE',  ( -0.000000000000000000, 1.000000000000000000, -0.000000000000000000 ) ) ;
#18113=CARTESIAN_POINT ( 'NONE',  ( 13.00000000000024336, -2.516660498395250745, -105.0000000000000142 ) ) ;
#18120=VERTEX_POINT ( 'NONE', #17628 ) ;
#18122=ADVANCED_FACE ( 'NONE', ( #1933 ), #18281, .F. ) ;
#18123=EDGE_CURVE ( 'NONE', #1794, #19351, #15329, .T. ) ;
#18125=CARTESIAN_POINT ( 'NONE',  ( 19.99999999999998224, 20.97067337953453858, -60.62177826491070221 ) ) ;
#18126=AXIS2_PLACEMENT_3D ( 'NONE', #20486, #9932, #22432 ) ;
#18128=CARTESIAN_POINT ( 'NONE',  ( 6.215609608695158883, 39.75345721999698867, -52.92319077873423794 ) ) ;
#18129=DIRECTION ( 'NONE',  ( -0.000000000000000000, -0.000000000000000000, 1.000000000000000000 ) ) ;
#18130=DIRECTION ( 'NONE',  ( 8.659560562351929024E-17, -0.7071067811867928210, 0.7071067811863022134 ) ) ;
#18131=ORIENTED_EDGE ( 'NONE', *, *, #19732, .F. ) ;
#18133=CYLINDRICAL_SURFACE ( 'NONE', #13802, 10.00000000000000178 ) ;
#18135=CARTESIAN_POINT ( 'NONE',  ( -0.3688098923350720537, -0.009433325537011738246, 50.78496022600280924 ) ) ;
#18142=CARTESIAN_POINT ( 'NONE',  ( 2.881552333950327061, 39.80724601559477094, 51.34430340187066122 ) ) ;
#18143=EDGE_CURVE ( 'NONE', #2375, #7505, #16081, .T. ) ;
#18149=CARTESIAN_POINT ( 'NONE',  ( 44.60000000000000853, -9.600000000000001421, -47.50000000000000000 ) ) ;
#18150=CARTESIAN_POINT ( 'NONE',  ( -10.49999999999980282, -2.516660498395515866, -105.0000000000000142 ) ) ;
#18153=DIRECTION ( 'NONE',  ( 0.000000000000000000, 0.000000000000000000, 1.000000000000000000 ) ) ;
#18156=ORIENTED_EDGE ( 'NONE', *, *, #18143, .T. ) ;
#18157=EDGE_LOOP ( 'NONE', ( #10423, #4058, #14269, #20101 ) ) ;
#18164=TOROIDAL_SURFACE ( 'NONE', #8641, 50.00000000000000000, 10.00000000000000000 ) ;
#18167=DIRECTION ( 'NONE',  ( -0.000000000000000000, -1.000000000000000000, -0.000000000000000000 ) ) ;
#18171=CARTESIAN_POINT ( 'NONE',  ( 12.11890052765070713, 39.66666666666666430, -54.74394698394421965 ) ) ;
#18174=FACE_OUTER_BOUND ( 'NONE', #4970, .T. ) ;
#18176=CARTESIAN_POINT ( 'NONE',  ( 42.50000000000000711, -12.00000000000012434, -50.02500000000011227 ) ) ;
#18178=ORIENTED_EDGE ( 'NONE', *, *, #5649, .T. ) ;
#18184=B_SPLINE_CURVE_WITH_KNOTS ( 'NONE', 3,
 ( #343, #5287, #16033, #17640, #1948, #6897 ),
 .UNSPECIFIED., .F., .F.,
 ( 4, 2, 4 ),
 ( 0.000000000000000000, 0.002641318319677492515, 0.005282636639354985029 ),
 .UNSPECIFIED. ) ;
#18186=AXIS2_PLACEMENT_3D ( 'NONE', #5657, #2338, #14234 ) ;
#18188=CARTESIAN_POINT ( 'NONE',  ( 1.387778780781445676E-14, 40.00000000000000000, 48.73397172404482802 ) ) ;
#18194=VERTEX_POINT ( 'NONE', #13138 ) ;
#18196=ADVANCED_FACE ( 'NONE', ( #21756 ), #17967, .F. ) ;
#18202=CIRCLE ( 'NONE', #9419, 22.00000000000000000 ) ;
#18211=EDGE_CURVE ( 'NONE', #18787, #11321, #3657, .T. ) ;
#18213=CARTESIAN_POINT ( 'NONE',  ( 2.425343827396499563, 40.00000000000000000, -50.22135669491186150 ) ) ;
#18214=EDGE_LOOP ( 'NONE', ( #9111, #3946 ) ) ;
#18215=CARTESIAN_POINT ( 'NONE',  ( 1.814350108393116612, 39.98032087727209216, -50.09305062634004457 ) ) ;
#18218=VERTEX_POINT ( 'NONE', #21875 ) ;
#18228=CARTESIAN_POINT ( 'NONE',  ( 13.33780792069982724, 2.142135623730938132, 45.06383732350703042 ) ) ;
#18229=ORIENTED_EDGE ( 'NONE', *, *, #22331, .T. ) ;
#18232=DIRECTION ( 'NONE',  ( 0.000000000000000000, 0.000000000000000000, -1.000000000000000000 ) ) ;
#18233=EDGE_CURVE ( 'NONE', #6550, #7020, #6942, .T. ) ;
#18237=VECTOR ( 'NONE', #19967, 1000.000000000000000 ) ;
#18238=EDGE_LOOP ( 'NONE', ( #9202, #9748, #8550, #17950 ) ) ;
#18240=EDGE_LOOP ( 'NONE', ( #15542, #3106, #17726, #10475 ) ) ;
#18241=ORIENTED_EDGE ( 'NONE', *, *, #8521, .T. ) ;
#18244=CARTESIAN_POINT ( 'NONE',  ( 17.68684951551751539, 29.34943212427064196, -60.02035230153429524 ) ) ;
#18245=CARTESIAN_POINT ( 'NONE',  ( 9.367793990832153028, -4.928932186883191235, 51.00106331757443456 ) ) ;
#18248=DIRECTION ( 'NONE',  ( 0.000000000000000000, 0.000000000000000000, 1.000000000000000000 ) ) ;
#18249=ORIENTED_EDGE ( 'NONE', *, *, #789, .F. ) ;
#18254=CARTESIAN_POINT ( 'NONE',  ( -13.56354382738803999, 2.142135623730931471, -56.03997097393684612 ) ) ;
#18255=CARTESIAN_POINT ( 'NONE',  ( 14.84934717125626946, 6.596698521592450071, -59.12425370493863142 ) ) ;
#18258=EDGE_CURVE ( 'NONE', #18626, #10068, #12416, .T. ) ;
#18261=CIRCLE ( 'NONE', #16029, 18.00000000000000355 ) ;
#18262=CARTESIAN_POINT ( 'NONE',  ( -5.511187417680089240, 0.6970053750307799723, -52.42166665191985686 ) ) ;
#18264=DIRECTION ( 'NONE',  ( 0.000000000000000000, -1.000000000000000000, 0.000000000000000000 ) ) ;
#18267=CARTESIAN_POINT ( 'NONE',  ( 9.829668860674836139, 37.49547983896071912, -57.11616152308156558 ) ) ;
#18273=AXIS2_PLACEMENT_3D ( 'NONE', #1648, #15491, #16993 ) ;
#18278=CARTESIAN_POINT ( 'NONE',  ( -2.836563456948004695E-15, -1.236374842841498678, -48.24164917503444627 ) ) ;
#18281=TOROIDAL_SURFACE ( 'NONE', #20478, 22.00000000000000000, 2.000000000000000000 ) ;
#18282=EDGE_LOOP ( 'NONE', ( #7456, #1445, #20576, #3532 ) ) ;
#18285=DIRECTION ( 'NONE',  ( -0.000000000000000000, -1.000000000000000000, -0.000000000000000000 ) ) ;
#18286=CARTESIAN_POINT ( 'NONE',  ( -90.00000000000000000, 24.73819270004212356, -9.108981535246192915E-16 ) ) ;
#18288=EDGE_CURVE ( 'NONE', #1702, #9194, #18341, .T. ) ;
#18294=ORIENTED_EDGE ( 'NONE', *, *, #7408, .F. ) ;
#18297=CARTESIAN_POINT ( 'NONE',  ( -21.29213537401196632, 12.67546417994314290, 58.41859095437464333 ) ) ;
#18298=CARTESIAN_POINT ( 'NONE',  ( -35.00000000000000000, 40.00000000000000000, 1.387778780781445676E-14 ) ) ;
#18299=FACE_BOUND ( 'NONE', #20213, .T. ) ;
#18300=CARTESIAN_POINT ( 'NONE',  ( -0.2893420571180744250, -0.01224453477246341404, -48.63018218499168910 ) ) ;
#18302=FACE_OUTER_BOUND ( 'NONE', #4500, .T. ) ;
#18306=CARTESIAN_POINT ( 'NONE',  ( 25.99999999999998579, 19.99999999999999645, 60.00099999999999767 ) ) ;
#18309=DIRECTION ( 'NONE',  ( -1.000000000000000000, 0.000000000000000000, 0.000000000000000000 ) ) ;
#18311=CARTESIAN_POINT ( 'NONE',  ( 90.00000000000000000, 28.00000000000000000, -9.108981535246192915E-16 ) ) ;
#18315=CARTESIAN_POINT ( 'NONE',  ( 29.99999999999998579, 20.00000000000000711, 100.0000000000000000 ) ) ;
#18316=CYLINDRICAL_SURFACE ( 'NONE', #4253, 2.099999999999997868 ) ;
#18319=EDGE_CURVE ( 'NONE', #18025, #12070, #20379, .T. ) ;
#18323=CARTESIAN_POINT ( 'NONE',  ( 5.863462918964529536, 39.99999999999999289, -52.03112467568187327 ) ) ;
#18325=CARTESIAN_POINT ( 'NONE',  ( 1.328666390486187066, 39.98974554208385968, -49.74045989696038816 ) ) ;
#18328=CARTESIAN_POINT ( 'NONE',  ( -3.092934392865752891, 39.99999999999999289, 50.60141176657413098 ) ) ;
#18329=CARTESIAN_POINT ( 'NONE',  ( 10.71765026523584829, 39.18334136350156882, -54.91251049708800025 ) ) ;
#18330=DIRECTION ( 'NONE',  ( -0.000000000000000000, -1.000000000000000000, -0.000000000000000000 ) ) ;
#18331=CIRCLE ( 'NONE', #17956, 2.524999999999999467 ) ;
#18333=VERTEX_POINT ( 'NONE', #22333 ) ;
#18335=DIRECTION ( 'NONE',  ( 0.000000000000000000, 1.000000000000000000, 0.000000000000000000 ) ) ;
#18336=CARTESIAN_POINT ( 'NONE',  ( -0.01944734386466554985, 39.99999780157233431, -48.74910573947852299 ) ) ;
#18341=B_SPLINE_CURVE_WITH_KNOTS ( 'NONE', 3,
 ( #8010, #18764, #1227, #15187, #16824, #21990, #8224, #20265, #22436, #13472, #6282, #10040, #22212 ),
 .UNSPECIFIED., .F., .F.,
 ( 4, 2, 1, 1, 1, 2, 2, 4 ),
 ( 0.000000000000000000, 0.2499999999999900080, 0.3749999999999875100, 0.4374999999999895084, 0.4687499999999898415, 0.4843749999999922839, 0.4999999999999947820, 1.000000000000000000 ),
 .UNSPECIFIED. ) ;
#18345=CARTESIAN_POINT ( 'NONE',  ( 11.03199507241028066, 39.99999999999999289, 53.98106524768372338 ) ) ;
#18346=CARTESIAN_POINT ( 'NONE',  ( -35.00000000000000000, -4.928932188134504955, 1.387778780781445676E-14 ) ) ;
#18348=DIRECTION ( 'NONE',  ( -0.000000000000000000, -1.000000000000000000, -0.000000000000000000 ) ) ;
#18349=CARTESIAN_POINT ( 'NONE',  ( 2.090752864397209532, 5.144172964797016689, -38.95144853163193943 ) ) ;
#18353=VERTEX_POINT ( 'NONE', #18539 ) ;
#18354=CARTESIAN_POINT ( 'NONE',  ( -5.833333333333337478, 6.180730040185833829, -40.61164310337066041 ) ) ;
#18356=CARTESIAN_POINT ( 'NONE',  ( 90.00000000000000000, 39.97500000000000142, -9.108981535246192915E-16 ) ) ;
#18361=CARTESIAN_POINT ( 'NONE',  ( 5.302679949206165588, 39.28774282260669537, -54.25155191766006624 ) ) ;
#18363=DIRECTION ( 'NONE',  ( 0.000000000000000000, -0.5150380749100547106, -0.8571673007021120005 ) ) ;
#18364=CARTESIAN_POINT ( 'NONE',  ( -7.505578006075234399, 1.461761173328252950, -55.63523492904088386 ) ) ;
#18366=ORIENTED_EDGE ( 'NONE', *, *, #7625, .F. ) ;
#18369=FACE_BOUND ( 'NONE', #21654, .T. ) ;
#18370=CARTESIAN_POINT ( 'NONE',  ( -15.00000000000001421, 20.00000000000000355, -105.0020000000000095 ) ) ;
#18372=CARTESIAN_POINT ( 'NONE',  ( 19.81218727895565124, 22.86772234701075490, -58.09777938302214295 ) ) ;
#18375=EDGE_LOOP ( 'NONE', ( #15601, #5258, #4940, #21332 ) ) ;
#18385=EDGE_CURVE ( 'NONE', #20079, #13970, #11697, .T. ) ;
#18392=AXIS2_PLACEMENT_3D ( 'NONE', #4190, #19776, #18038 ) ;
#18396=ORIENTED_EDGE ( 'NONE', *, *, #22395, .F. ) ;
#18400=CARTESIAN_POINT ( 'NONE',  ( -17.41694144196565119, 10.15895996405112456, 59.94253659024146685 ) ) ;
#18405=CARTESIAN_POINT ( 'NONE',  ( 0.4211638912362005716, -0.02267170258719574880, -49.14966933624602774 ) ) ;
#18406=EDGE_CURVE ( 'NONE', #7389, #10163, #3596, .T. ) ;
#18407=CONICAL_SURFACE ( 'NONE', #1940, 8.999999999999973355, 0.7853981633974657095 ) ;
#18409=CARTESIAN_POINT ( 'NONE',  ( 1.591932335265033587E-15, -4.923002280079127832E-27, 50.50395615645412306 ) ) ;
#18410=CARTESIAN_POINT ( 'NONE',  ( 9.689843208404433028, 39.33333333333334991, 54.54983754392749518 ) ) ;
#18411=CARTESIAN_POINT ( 'NONE',  ( -5.340789179572220213, 39.27722415257183286, -54.28402915905239468 ) ) ;
#18412=CARTESIAN_POINT ( 'NONE',  ( -42.50000000000000711, -12.00000000000012434, 47.50000000000000711 ) ) ;
#18416=CARTESIAN_POINT ( 'NONE',  ( -0.6237373291637031691, 39.99088417130654705, -49.47180386667445617 ) ) ;
#18421=DIRECTION ( 'NONE',  ( 0.000000000000000000, 0.000000000000000000, -1.000000000000000000 ) ) ;
#18422=ORIENTED_EDGE ( 'NONE', *, *, #3927, .F. ) ;
#18426=EDGE_CURVE ( 'NONE', #19936, #9264, #17606, .T. ) ;
#18427=AXIS2_PLACEMENT_3D ( 'NONE', #15686, #17288, #15341 ) ;
#18429=EDGE_LOOP ( 'NONE', ( #8262, #8929 ) ) ;
#18430=CARTESIAN_POINT ( 'NONE',  ( 21.99999999999998579, 20.00000000000000355, -98.00000000000000000 ) ) ;
#18431=CIRCLE ( 'NONE', #17745, 30.00000000000000000 ) ;
#18435=CARTESIAN_POINT ( 'NONE',  ( 6.745307376263603771, 39.70676877995263965, -53.21562790720045655 ) ) ;
#18437=AXIS2_PLACEMENT_3D ( 'NONE', #20162, #11336, #18089 ) ;
#18440=CARTESIAN_POINT ( 'NONE',  ( 10.48823472801903200, 39.21814192261259535, -54.82890001962670112 ) ) ;
#18442=EDGE_CURVE ( 'NONE', #20626, #12113, #6236, .T. ) ;
#18448=CARTESIAN_POINT ( 'NONE',  ( -34.99999999999999289, 38.99999999999999289, 60.00000000000001421 ) ) ;
#18450=FACE_OUTER_BOUND ( 'NONE', #11871, .T. ) ;
#18455=CARTESIAN_POINT ( 'NONE',  ( -42.50000000000000711, -11.97499999999999964, -50.00000000000000000 ) ) ;
#18460=EDGE_LOOP ( 'NONE', ( #16307, #14711, #12050 ) ) ;
#18461=CARTESIAN_POINT ( 'NONE',  ( 8.331955809010601399, 38.18181818181818699, 56.36098470834073026 ) ) ;
#18466=CARTESIAN_POINT ( 'NONE',  ( 35.00000000000058265, 26.00000000000000355, -55.00000000000076028 ) ) ;
#18467=ORIENTED_EDGE ( 'NONE', *, *, #22658, .T. ) ;
#18468=DIRECTION ( 'NONE',  ( -0.000000000000000000, -1.000000000000000000, -0.000000000000000000 ) ) ;
#18471=CARTESIAN_POINT ( 'NONE',  ( -14.69988787053504531, 16.91499873015103006, -45.69379240540676790 ) ) ;
#18472=EDGE_CURVE ( 'NONE', #10163, #21119, #10829, .T. ) ;
#18473=CARTESIAN_POINT ( 'NONE',  ( -21.80163436544122746, 14.71892543950344923, -58.53048140122280074 ) ) ;
#18477=CARTESIAN_POINT ( 'NONE',  ( 19.95262135541528892, 18.40707545474674589, -60.61067493606136480 ) ) ;
#18479=CARTESIAN_POINT ( 'NONE',  ( -2.774848922471319757, 40.00000000000000000, -50.42374039355618009 ) ) ;
#18481=EDGE_LOOP ( 'NONE', ( #2269, #17474, #2439, #17325 ) ) ;
#18486=CYLINDRICAL_SURFACE ( 'NONE', #20987, 2.499999999999995115 ) ;
#18489=CARTESIAN_POINT ( 'NONE',  ( 15.99370094303709955, 7.960486082689420151, -59.50964696496923523 ) ) ;
#18495=VERTEX_POINT ( 'NONE', #18052 ) ;
#18498=EDGE_CURVE ( 'NONE', #18984, #19146, #10954, .T. ) ;
#18501=CARTESIAN_POINT ( 'NONE',  ( -8.523345606559670884, -2.856915207742760199, -52.89411661591344682 ) ) ;
#18505=CIRCLE ( 'NONE', #21823, 51.00000000000001421 ) ;
#18509=LINE ( 'NONE', #21497, #12726 ) ;
#18513=CARTESIAN_POINT ( 'NONE',  ( -1.387778780781445518E-14, 20.00000000000000355, 100.0000000000000000 ) ) ;
#18516=AXIS2_PLACEMENT_3D ( 'NONE', #408, #7400, #12774 ) ;
#18517=ORIENTED_EDGE ( 'NONE', *, *, #22265, .F. ) ;
#18518=CIRCLE ( 'NONE', #17799, 57.00000000000002132 ) ;
#18521=CARTESIAN_POINT ( 'NONE',  ( -16.72418712225133675, 8.992692292682194832, 57.18730031742740749 ) ) ;
#18522=EDGE_CURVE ( 'NONE', #12474, #20078, #17555, .T. ) ;
#18526=CARTESIAN_POINT ( 'NONE',  ( -11.12223430625391707, 40.00000000000000711, 54.01173000072970609 ) ) ;
#18527=CARTESIAN_POINT ( 'NONE',  ( -40.40000000000001279, -9.600000000000001421, 47.50000000000000711 ) ) ;
#18529=CARTESIAN_POINT ( 'NONE',  ( -35.00000000000000000, 40.00000000000000000, 1.387778780781445676E-14 ) ) ;
#18533=CARTESIAN_POINT ( 'NONE',  ( 1.583519045122365076, -4.618580011808620434, 46.65783332780151227 ) ) ;
#18535=AXIS2_PLACEMENT_3D ( 'NONE', #5189, #8945, #3698 ) ;
#18539=CARTESIAN_POINT ( 'NONE',  ( -42.50000000000000711, -3.738192700042122674, -47.50000000000000000 ) ) ;
#18540=DIRECTION ( 'NONE',  ( -0.000000000000000000, -1.000000000000000000, -0.000000000000000000 ) ) ;
#18544=CARTESIAN_POINT ( 'NONE',  ( 35.00000000000000000, 39.00000000000000711, 4.258610482196280173E-15 ) ) ;
#18545=FACE_OUTER_BOUND ( 'NONE', #13388, .T. ) ;
#18549=EDGE_CURVE ( 'NONE', #6464, #19292, #6954, .T. ) ;
#18550=TOROIDAL_SURFACE ( 'NONE', #20389, 18.00000000000000355, 4.000000000000000000 ) ;
#18556=EDGE_CURVE ( 'NONE', #10193, #1471, #20135, .T. ) ;
#18557=DIRECTION ( 'NONE',  ( -0.000000000000000000, 1.000000000000000000, -0.000000000000000000 ) ) ;
#18558=CARTESIAN_POINT ( 'NONE',  ( 10.64189282826238170, 39.19489805863617704, -54.88474174631790703 ) ) ;
#18559=CARTESIAN_POINT ( 'NONE',  ( -8.199064559763622029, 32.63945871574319568, -42.22991907770641262 ) ) ;
#18560=CIRCLE ( 'NONE', #1014, 15.99999999999993072 ) ;
#18561=CARTESIAN_POINT ( 'NONE',  ( -15.50000000000011013, 42.51666049839536043, -100.0000000000000000 ) ) ;
#18563=EDGE_LOOP ( 'NONE', ( #22305, #3010, #2674, #11907 ) ) ;
#18565=VECTOR ( 'NONE', #17307, 1000.000000000000000 ) ;
#18566=LINE ( 'NONE', #9860, #14034 ) ;
#18567=CARTESIAN_POINT ( 'NONE',  ( 12.27586057105627582, 4.193657236093733864, -55.54740530681009858 ) ) ;
#18568=CARTESIAN_POINT ( 'NONE',  ( -34.99999999999999289, 39.00000000000000711, 50.00000000000000000 ) ) ;
#18570=ORIENTED_EDGE ( 'NONE', *, *, #22016, .T. ) ;
#18571=CARTESIAN_POINT ( 'NONE',  ( 42.50000000000000711, -12.00000000000000000, -50.00000000000000000 ) ) ;
#18574=EDGE_CURVE ( 'NONE', #13854, #18007, #742, .T. ) ;
#18578=EDGE_CURVE ( 'NONE', #7926, #3138, #12337, .T. ) ;
#18582=ORIENTED_EDGE ( 'NONE', *, *, #6998, .T. ) ;
#18584=CIRCLE ( 'NONE', #19688, 2.500000000000002220 ) ;
#18586=CARTESIAN_POINT ( 'NONE',  ( 11.50056215611667554, 36.46966885432792083, -57.85578624339546394 ) ) ;
#18589=CARTESIAN_POINT ( 'NONE',  ( 16.30820259622263890, 8.415540886845231938, 59.60694662124535625 ) ) ;
#18590=DIRECTION ( 'NONE',  ( 0.000000000000000000, 0.000000000000000000, -1.000000000000000000 ) ) ;
#18591=EDGE_LOOP ( 'NONE', ( #5032, #15678 ) ) ;
#18597=CARTESIAN_POINT ( 'NONE',  ( 35.00000000000000711, 39.00000000000000711, -49.99999999999997868 ) ) ;
#18600=DIRECTION ( 'NONE',  ( -0.000000000000000000, -0.000000000000000000, -1.000000000000000000 ) ) ;
#18603=EDGE_LOOP ( 'NONE', ( #13861, #16198, #5460, #7801 ) ) ;
#18605=CARTESIAN_POINT ( 'NONE',  ( -6.094386425459117795, 0.8904119427534493703, -54.73837739180613227 ) ) ;
#18606=AXIS2_PLACEMENT_3D ( 'NONE', #10569, #7137, #21126 ) ;
#18607=ORIENTED_EDGE ( 'NONE', *, *, #14768, .F. ) ;
#18608=VECTOR ( 'NONE', #21404, 1000.000000000000000 ) ;
#18610=DIRECTION ( 'NONE',  ( -0.000000000000000000, -0.000000000000000000, -1.000000000000000000 ) ) ;
#18611=FACE_OUTER_BOUND ( 'NONE', #653, .T. ) ;
#18613=CARTESIAN_POINT ( 'NONE',  ( 18.97285531159653971, 26.38757670764486463, -60.36948798341702371 ) ) ;
#18622=CARTESIAN_POINT ( 'NONE',  ( 10.50000000000024514, -2.516660498395250745, 60.00099999999999767 ) ) ;
#18626=VERTEX_POINT ( 'NONE', #11365 ) ;
#18628=CARTESIAN_POINT ( 'NONE',  ( -5.748506628232283866, -0.6819283742247831404, -52.01451867725678113 ) ) ;
#18632=VERTEX_POINT ( 'NONE', #9538 ) ;
#18633=CARTESIAN_POINT ( 'NONE',  ( 5.133463079812987218, 39.34078236626471892, -53.02544357726076640 ) ) ;
#18636=CARTESIAN_POINT ( 'NONE',  ( -13.65693838750921607, 34.64075751992690755, -58.69913499740199825 ) ) ;
#18638=VECTOR ( 'NONE', #18468, 1000.000000000000000 ) ;
#18643=VERTEX_POINT ( 'NONE', #11249 ) ;
#18644=ORIENTED_EDGE ( 'NONE', *, *, #15920, .T. ) ;
#18645=CARTESIAN_POINT ( 'NONE',  ( -19.35294509712510092, 31.41613210955674518, 57.92571537617230604 ) ) ;
#18648=CARTESIAN_POINT ( 'NONE',  ( -15.59166974688846707, 7.467814210042477363, -59.37578565761233307 ) ) ;
#18649=CYLINDRICAL_SURFACE ( 'NONE', #1226, 2.500000000000002220 ) ;
#18650=ORIENTED_EDGE ( 'NONE', *, *, #10683, .T. ) ;
#18652=CARTESIAN_POINT ( 'NONE',  ( -1.387778780781445676E-14, 40.00000000000000000, -48.73397172404481381 ) ) ;
#18654=DIRECTION ( 'NONE',  ( 0.000000000000000000, -1.000000000000000000, 0.000000000000000000 ) ) ;
#18655=ADVANCED_FACE ( 'NONE', ( #4277 ), #9645, .F. ) ;
#18658=ORIENTED_EDGE ( 'NONE', *, *, #18472, .T. ) ;
#18663=CARTESIAN_POINT ( 'NONE',  ( -12.84899528830097104, 2.142135623730931471, -57.90797000640141334 ) ) ;
#18670=ADVANCED_FACE ( 'NONE', ( #16636 ), #5869, .T. ) ;
#18671=FACE_OUTER_BOUND ( 'NONE', #186, .T. ) ;
#18679=CARTESIAN_POINT ( 'NONE',  ( -14.05436202270911217, 25.29714423467776996, -45.40204559108963878 ) ) ;
#18680=CARTESIAN_POINT ( 'NONE',  ( 90.00000000000000000, 26.00000000000000355, -9.108981535246192915E-16 ) ) ;
#18681=VERTEX_POINT ( 'NONE', #6216 ) ;
#18684=CARTESIAN_POINT ( 'NONE',  ( 6.696867368503558448E-15, 0.000000000000000000, 38.73397172404480671 ) ) ;
#18685=CARTESIAN_POINT ( 'NONE',  ( 35.00000000000000000, 0.000000000000000000, 4.258610482196280173E-15 ) ) ;
#18688=DIRECTION ( 'NONE',  ( -0.000000000000000000, -1.000000000000000000, -0.000000000000000000 ) ) ;
#18689=FACE_OUTER_BOUND ( 'NONE', #22517, .T. ) ;
#18695=DIRECTION ( 'NONE',  ( 0.000000000000000000, 0.000000000000000000, -1.000000000000000000 ) ) ;
#18696=FACE_OUTER_BOUND ( 'NONE', #4782, .T. ) ;
#18697=CIRCLE ( 'NONE', #21630, 2.499999999999995115 ) ;
#18702=LINE ( 'NONE', #6441, #10204 ) ;
#18704=VERTEX_POINT ( 'NONE', #2670 ) ;
#18706=CARTESIAN_POINT ( 'NONE',  ( -12.70473862104220864, 11.99136930790644229, -44.75655646380167951 ) ) ;
#18710=CARTESIAN_POINT ( 'NONE',  ( 8.776846306732625891, 39.47243301244805025, 54.19537464444116637 ) ) ;
#18712=CARTESIAN_POINT ( 'NONE',  ( -8.847970493949620874, 40.00000000000000711, -53.28481329731337723 ) ) ;
#18713=ORIENTED_EDGE ( 'NONE', *, *, #3658, .F. ) ;
#18714=CARTESIAN_POINT ( 'NONE',  ( 2.496587642955522490, 0.1153990516131240540, -52.32802461649443870 ) ) ;
#18715=CARTESIAN_POINT ( 'NONE',  ( -0.4213896610233284767, -0.02267536297422790767, -49.14983462332308761 ) ) ;
#18718=CARTESIAN_POINT ( 'NONE',  ( 42.50000000000000711, -11.97499999999999964, -47.50000000000000000 ) ) ;
#18720=DIRECTION ( 'NONE',  ( 0.000000000000000000, 0.000000000000000000, -1.000000000000000000 ) ) ;
#18721=CARTESIAN_POINT ( 'NONE',  ( 15.40035801025553752, 32.79675990107260475, -56.74176776513677822 ) ) ;
#18722=ORIENTED_EDGE ( 'NONE', *, *, #2636, .T. ) ;
#18723=ORIENTED_EDGE ( 'NONE', *, *, #1155, .T. ) ;
#18724=ORIENTED_EDGE ( 'NONE', *, *, #2466, .T. ) ;
#18725=CYLINDRICAL_SURFACE ( 'NONE', #4725, 49.99999999999998579 ) ;
#18727=CARTESIAN_POINT ( 'NONE',  ( 11.86180952233169705, 39.00000000000000000, 55.35904751184887118 ) ) ;
#18728=CARTESIAN_POINT ( 'NONE',  ( 42.50000000000000711, -9.600000000000001421, -47.50000000000000000 ) ) ;
#18732=FACE_OUTER_BOUND ( 'NONE', #6603, .T. ) ;
#18736=CARTESIAN_POINT ( 'NONE',  ( 8.331955809010628045, 38.18181818181817277, -56.36098470834072316 ) ) ;
#18739=CARTESIAN_POINT ( 'NONE',  ( -16.16780438139469211, 31.78273399965604540, -59.56292242448184027 ) ) ;
#18743=CARTESIAN_POINT ( 'NONE',  ( -12.06668108811419771, 11.08190912999966038, 44.43106897542665479 ) ) ;
#18744=EDGE_CURVE ( 'NONE', #18953, #6097, #2319, .T. ) ;
#18746=VERTEX_POINT ( 'NONE', #7814 ) ;
#18748=CARTESIAN_POINT ( 'NONE',  ( -19.81218727895213405, 22.86772234701062700, 58.09777938301198219 ) ) ;
#18752=DIRECTION ( 'NONE',  ( 0.000000000000000000, 1.000000000000000000, 0.000000000000000000 ) ) ;
#18754=AXIS2_PLACEMENT_3D ( 'NONE', #9343, #7284, #21486 ) ;
#18756=VERTEX_POINT ( 'NONE', #6101 ) ;
#18757=CARTESIAN_POINT ( 'NONE',  ( -10.49999999999980282, -2.516660498395515866, -100.0000000000000000 ) ) ;
#18758=CARTESIAN_POINT ( 'NONE',  ( -8.578904148414546071, 40.00000000000000711, -53.18551243551740981 ) ) ;
#18760=CARTESIAN_POINT ( 'NONE',  ( 11.86180952234068364, 38.99999999999457145, -55.35904751185260864 ) ) ;
#18763=ORIENTED_EDGE ( 'NONE', *, *, #10974, .F. ) ;
#18764=CARTESIAN_POINT ( 'NONE',  ( -9.886810797454463895, 39.30595911725853142, 54.61697552269315992 ) ) ;
#18765=ORIENTED_EDGE ( 'NONE', *, *, #19133, .F. ) ;
#18769=FACE_BOUND ( 'NONE', #15746, .T. ) ;
#18772=AXIS2_PLACEMENT_3D ( 'NONE', #8662, #14013, #5009 ) ;
#18774=ADVANCED_FACE ( 'NONE', ( #14896 ), #21923, .F. ) ;
#18776=CARTESIAN_POINT ( 'NONE',  ( -8.466980083302928506, -4.900852744035391950, 50.56985808960192230 ) ) ;
#18779=EDGE_CURVE ( 'NONE', #6315, #11727, #11131, .T. ) ;
#18780=CARTESIAN_POINT ( 'NONE',  ( 14.50678847729821896, 16.16560534949676509, 45.60743157421821081 ) ) ;
#18781=CARTESIAN_POINT ( 'NONE',  ( -2.855944605007508574, 34.72779906119552606, -39.14690304189947767 ) ) ;
#18783=CARTESIAN_POINT ( 'NONE',  ( -19.97206123483410423, 21.14267036293994906, -58.14006880918119435 ) ) ;
#18785=AXIS2_PLACEMENT_3D ( 'NONE', #8213, #10138, #13125 ) ;
#18786=CARTESIAN_POINT ( 'NONE',  ( -15.62385314663568714, 32.51590977305111352, 59.38867318806723006 ) ) ;
#18787=VERTEX_POINT ( 'NONE', #2444 ) ;
#18789=DIRECTION ( 'NONE',  ( 0.000000000000000000, 0.000000000000000000, 1.000000000000000000 ) ) ;
#18790=CIRCLE ( 'NONE', #1234, 10.00000000000000000 ) ;
#18791=CARTESIAN_POINT ( 'NONE',  ( -15.49999999999980460, -2.516660498395515866, 105.0000000000000142 ) ) ;
#18792=DIRECTION ( 'NONE',  ( 0.000000000000000000, 1.000000000000000000, 0.000000000000000000 ) ) ;
#18794=ORIENTED_EDGE ( 'NONE', *, *, #7776, .T. ) ;
#18801=ORIENTED_EDGE ( 'NONE', *, *, #22395, .T. ) ;
#18804=CIRCLE ( 'NONE', #15861, 2.524999999999999467 ) ;
#18809=FACE_OUTER_BOUND ( 'NONE', #16058, .T. ) ;
#18810=CARTESIAN_POINT ( 'NONE',  ( 14.06256854266893974, 5.693415384482566566, 58.85512087818932514 ) ) ;
#18817=CARTESIAN_POINT ( 'NONE',  ( -2.836563456948004695E-15, -1.236374842841498678, -48.24164917503444627 ) ) ;
#18818=DIRECTION ( 'NONE',  ( -0.000000000000000000, -0.000000000000000000, 1.000000000000000000 ) ) ;
#18821=DIRECTION ( 'NONE',  ( 0.000000000000000000, 0.000000000000000000, 1.000000000000000000 ) ) ;
#18824=CONICAL_SURFACE ( 'NONE', #8928, 49.99999999999998579, 0.7853981633974657095 ) ;
#18830=FACE_OUTER_BOUND ( 'NONE', #9754, .T. ) ;
#18831=CARTESIAN_POINT ( 'NONE',  ( 22.38366207802858909, 18.39979965017225538, -58.65857802150448919 ) ) ;
#18833=ADVANCED_FACE ( 'NONE', ( #20637 ), #22140, .F. ) ;
#18838=CARTESIAN_POINT ( 'NONE',  ( 35.00000000000000000, 40.00000000000000000, 4.258610482196280173E-15 ) ) ;
#18841=CIRCLE ( 'NONE', #1651, 9.000000000000003553 ) ;
#18844=ORIENTED_EDGE ( 'NONE', *, *, #11357, .F. ) ;
#18846=CARTESIAN_POINT ( 'NONE',  ( -4.026578693514479390, -4.679980696191891276, -48.24134193083673949 ) ) ;
#18850=CARTESIAN_POINT ( 'NONE',  ( 9.786572406442770600, 39.51694226791492781, -54.52237350754640488 ) ) ;
#18853=CARTESIAN_POINT ( 'NONE',  ( 6.696867368503558448E-15, 40.00000000000000000, 48.73397172404481381 ) ) ;
#18854=CARTESIAN_POINT ( 'NONE',  ( -2.180214370012230507, 39.97139195390602140, 50.35379697857760561 ) ) ;
#18855=EDGE_CURVE ( 'NONE', #16994, #21335, #22620, .T. ) ;
#18856=AXIS2_PLACEMENT_3D ( 'NONE', #5358, #12335, #19345 ) ;
#18857=CARTESIAN_POINT ( 'NONE',  ( -13.59841332577231299, 13.65742718326611715, 45.18857684126746221 ) ) ;
#18859=ORIENTED_EDGE ( 'NONE', *, *, #16424, .F. ) ;
#18860=VERTEX_POINT ( 'NONE', #13517 ) ;
#18861=ORIENTED_EDGE ( 'NONE', *, *, #12011, .F. ) ;
#18864=VERTEX_POINT ( 'NONE', #16751 ) ;
#18865=CARTESIAN_POINT ( 'NONE',  ( -11.86180952233172725, 39.00000000000000000, -55.35904751184885697 ) ) ;
#18868=CARTESIAN_POINT ( 'NONE',  ( -16.97759837164273122, 9.398593820328095205, -59.81443117571819812 ) ) ;
#18869=AXIS2_PLACEMENT_3D ( 'NONE', #8061, #19977, #7823 ) ;
#18870=DIRECTION ( 'NONE',  ( 0.000000000000000000, -1.000000000000000000, 0.000000000000000000 ) ) ;
#18872=VERTEX_POINT ( 'NONE', #1058 ) ;
#18879=CONICAL_SURFACE ( 'NONE', #22189, 2.099999999999997868, 1.029744258676652091 ) ;
#18883=CONICAL_SURFACE ( 'NONE', #11916, 58.99999999999994316, 0.7853981633974725929 ) ;
#18885=CARTESIAN_POINT ( 'NONE',  ( 19.99999999999998579, 20.00000000000000000, 60.62177826491070221 ) ) ;
#18886=CARTESIAN_POINT ( 'NONE',  ( -5.010575289839672486, 34.16656919735249431, 40.02075074423078149 ) ) ;
#18888=AXIS2_PLACEMENT_3D ( 'NONE', #1699, #15660, #1352 ) ;
#18889=EDGE_CURVE ( 'NONE', #4040, #14214, #5097, .T. ) ;
#18890=EDGE_LOOP ( 'NONE', ( #4664, #17116, #4427, #19745, #15402, #133, #17567 ) ) ;
#18891=CARTESIAN_POINT ( 'NONE',  ( -1.387778780781445676E-14, 20.00000000000000000, 60.00200000000000244 ) ) ;
#18893=AXIS2_PLACEMENT_3D ( 'NONE', #9881, #10313, #8275 ) ;
#18894=AXIS2_PLACEMENT_3D ( 'NONE', #9708, #21632, #778 ) ;
#18896=ORIENTED_EDGE ( 'NONE', *, *, #21516, .F. ) ;
#18897=VECTOR ( 'NONE', #9600, 1000.000000000000114 ) ;
#18898=CARTESIAN_POINT ( 'NONE',  ( 14.94062893683334003, 18.45609313704556342, 45.79998742252196564 ) ) ;
#18899=EDGE_CURVE ( 'NONE', #20510, #4801, #15121, .T. ) ;
#18900=LINE ( 'NONE', #3207, #3028 ) ;
#18902=CARTESIAN_POINT ( 'NONE',  ( -19.42731605661754202, 15.16896271047879807, -57.99434643146634727 ) ) ;
#18903=CARTESIAN_POINT ( 'NONE',  ( -5.398822262509256120, 39.81726523789954086, 52.45277322177971513 ) ) ;
#18905=CARTESIAN_POINT ( 'NONE',  ( -13.87722263113804644, 34.42803545437053003, 58.77926695580350014 ) ) ;
#18910=CYLINDRICAL_SURFACE ( 'NONE', #15487, 2.499999999999995115 ) ;
#18912=ORIENTED_EDGE ( 'NONE', *, *, #9895, .T. ) ;
#18915=EDGE_CURVE ( 'NONE', #16909, #10389, #5069, .T. ) ;
#18920=FACE_OUTER_BOUND ( 'NONE', #14056, .T. ) ;
#18921=CARTESIAN_POINT ( 'NONE',  ( 3.309563215939714365, -3.140776953262784943, 49.61090469809098380 ) ) ;
#18923=CARTESIAN_POINT ( 'NONE',  ( 19.99999999999998579, 20.00000000000000000, 60.62177826491070221 ) ) ;
#18924=LINE ( 'NONE', #19041, #19363 ) ;
#18927=DIRECTION ( 'NONE',  ( 0.000000000000000000, 0.000000000000000000, -1.000000000000000000 ) ) ;
#18935=CARTESIAN_POINT ( 'NONE',  ( 14.17374118098243940, 24.92453540474835805, -45.45638825402598826 ) ) ;
#18937=CARTESIAN_POINT ( 'NONE',  ( 14.99999999999998579, 20.00000000000000000, -105.0020000000000095 ) ) ;
#18945=DIRECTION ( 'NONE',  ( 0.000000000000000000, 0.000000000000000000, 1.000000000000000000 ) ) ;
#18948=CARTESIAN_POINT ( 'NONE',  ( 12.37316313323383632, 4.263667856435456649, -58.19925355777955644 ) ) ;
#18953=VERTEX_POINT ( 'NONE', #9055 ) ;
#18957=CARTESIAN_POINT ( 'NONE',  ( 21.90353326617355023, 15.16496266307568774, 58.55331524747137451 ) ) ;
#18958=CARTESIAN_POINT ( 'NONE',  ( -35.00000000000058265, 39.97500000000000142, -55.00000000000076028 ) ) ;
#18959=EDGE_CURVE ( 'NONE', #7430, #15875, #18184, .T. ) ;
#18961=VERTEX_POINT ( 'NONE', #13858 ) ;
#18962=FACE_BOUND ( 'NONE', #16604, .T. ) ;
#18967=ORIENTED_EDGE ( 'NONE', *, *, #19838, .T. ) ;
#18969=CIRCLE ( 'NONE', #2131, 57.07106781186551103 ) ;
#18972=CARTESIAN_POINT ( 'NONE',  ( -2.931973760223107522E-15, -2.515546993500582751, -47.48752710978099145 ) ) ;
#18974=CARTESIAN_POINT ( 'NONE',  ( -3.072149649144736649, 39.94358005063767791, 50.97360058146784212 ) ) ;
#18978=CARTESIAN_POINT ( 'NONE',  ( -14.87996495114181350, 18.06670563205965152, 45.77322900830828445 ) ) ;
#18983=EDGE_LOOP ( 'NONE', ( #6285, #10936, #21591, #4466, #22090, #20843, #4241, #14179, #16545 ) ) ;
#18984=VERTEX_POINT ( 'NONE', #5177 ) ;
#18990=DIRECTION ( 'NONE',  ( -0.000000000000000000, -1.000000000000000000, -0.000000000000000000 ) ) ;
#18991=CARTESIAN_POINT ( 'NONE',  ( -9.952189117650803496, 40.00000000000000000, 53.64426396172073908 ) ) ;
#18995=CARTESIAN_POINT ( 'NONE',  ( -7.563456402248210253, 40.00000000000000711, -52.78701496912255919 ) ) ;
#18999=CARTESIAN_POINT ( 'NONE',  ( 42.50000000000000711, -12.00000000000000000, 47.50000000000000711 ) ) ;
#19002=CARTESIAN_POINT ( 'NONE',  ( -8.331955809010628045, 38.18181818181818699, 56.36098470834075158 ) ) ;
#19008=EDGE_CURVE ( 'NONE', #7125, #20382, #10154, .T. ) ;
#19009=VERTEX_POINT ( 'NONE', #12472 ) ;
#19011=VERTEX_POINT ( 'NONE', #7722 ) ;
#19014=ORIENTED_EDGE ( 'NONE', *, *, #20881, .F. ) ;
#19015=CARTESIAN_POINT ( 'NONE',  ( 14.05436202270908375, 14.70285576532224425, 45.40204559108965299 ) ) ;
#19016=DIRECTION ( 'NONE',  ( 0.000000000000000000, 0.000000000000000000, -1.000000000000000000 ) ) ;
#19017=LINE ( 'NONE', #15327, #19329 ) ;
#19018=CARTESIAN_POINT ( 'NONE',  ( -19.96591191797318388, 18.54839033250632241, -58.13845218885094823 ) ) ;
#19022=CYLINDRICAL_SURFACE ( 'NONE', #13425, 2.499999999999998668 ) ;
#19023=FACE_OUTER_BOUND ( 'NONE', #19062, .T. ) ;
#19026=EDGE_CURVE ( 'NONE', #5986, #6323, #13300, .T. ) ;
#19027=ORIENTED_EDGE ( 'NONE', *, *, #20572, .T. ) ;
#19037=ORIENTED_EDGE ( 'NONE', *, *, #13890, .F. ) ;
#19038=CARTESIAN_POINT ( 'NONE',  ( 6.696867368503558448E-15, 39.00000000000000711, 38.73397172404480671 ) ) ;
#19039=CARTESIAN_POINT ( 'NONE',  ( 5.079212789370819436, -3.097595057461635992, 50.74825967503632285 ) ) ;
#19041=CARTESIAN_POINT ( 'NONE',  ( 35.00000000000000000, 25.00000000000000000, 9.000000000000007105 ) ) ;
#19042=EDGE_LOOP ( 'NONE', ( #13552, #7648 ) ) ;
#19043=CARTESIAN_POINT ( 'NONE',  ( 42.50000000000000711, -5.000000000000000000, 47.50000000000000711 ) ) ;
#19051=CARTESIAN_POINT ( 'NONE',  ( 11.13407802442741179, 30.05807871779232343, -43.93745127716449872 ) ) ;
#19054=CARTESIAN_POINT ( 'NONE',  ( -42.50000000000000711, -12.00000000000000000, 50.00000000000000711 ) ) ;
#19055=ORIENTED_EDGE ( 'NONE', *, *, #15054, .F. ) ;
#19059=CARTESIAN_POINT ( 'NONE',  ( 15.23870778339282772, 7.010517948053573534, -56.68442755504732133 ) ) ;
#19061=CIRCLE ( 'NONE', #20530, 18.00000000000000355 ) ;
#19062=EDGE_LOOP ( 'NONE', ( #22388, #8876 ) ) ;
#19063=ORIENTED_EDGE ( 'NONE', *, *, #16424, .T. ) ;
#19064=DIRECTION ( 'NONE',  ( 0.000000000000000000, 0.000000000000000000, -1.000000000000000000 ) ) ;
#19065=EDGE_CURVE ( 'NONE', #17245, #1538, #20412, .T. ) ;
#19066=ORIENTED_EDGE ( 'NONE', *, *, #21587, .T. ) ;
#19068=CARTESIAN_POINT ( 'NONE',  ( 35.00000000000000711, 40.00000000000000000, 49.99999999999999289 ) ) ;
#19069=DIRECTION ( 'NONE',  ( 0.000000000000000000, 0.000000000000000000, -1.000000000000000000 ) ) ;
#19073=DIRECTION ( 'NONE',  ( -0.000000000000000000, -0.000000000000000000, 1.000000000000000000 ) ) ;
#19074=EDGE_LOOP ( 'NONE', ( #19402, #22693 ) ) ;
#19076=EDGE_CURVE ( 'NONE', #7279, #10462, #6574, .T. ) ;
#19077=CARTESIAN_POINT ( 'NONE',  ( -3.591923118226331086E-15, -5.000000000000000000, -44.98888751680799203 ) ) ;
#19079=CARTESIAN_POINT ( 'NONE',  ( 6.450245752248383369, 39.75603576625821489, -53.02615179544272905 ) ) ;
#19083=LINE ( 'NONE', #8872, #10331 ) ;
#19088=AXIS2_PLACEMENT_3D ( 'NONE', #13278, #11477, #9760 ) ;
#19089=ORIENTED_EDGE ( 'NONE', *, *, #18319, .F. ) ;
#19090=ORIENTED_EDGE ( 'NONE', *, *, #2072, .T. ) ;
#19092=ORIENTED_EDGE ( 'NONE', *, *, #6352, .F. ) ;
#19093=DIRECTION ( 'NONE',  ( -1.000000000000000000, -0.000000000000000000, -0.000000000000000000 ) ) ;
#19097=CARTESIAN_POINT ( 'NONE',  ( 1.619910636035357454, 39.98468599264958101, 49.95346646087499920 ) ) ;
#19099=EDGE_LOOP ( 'NONE', ( #14875, #7105, #5968, #5888 ) ) ;
#19100=DIRECTION ( 'NONE',  ( -0.000000000000000000, -1.000000000000000000, -0.000000000000000000 ) ) ;
#19101=DIRECTION ( 'NONE',  ( 0.000000000000000000, 1.000000000000000000, 0.000000000000000000 ) ) ;
#19104=LINE ( 'NONE', #20941, #1059 ) ;
#19111=CARTESIAN_POINT ( 'NONE',  ( -8.234904025113911175, 38.24530784312006659, 54.56725976436211312 ) ) ;
#19113=FACE_OUTER_BOUND ( 'NONE', #2805, .T. ) ;
#19116=VERTEX_POINT ( 'NONE', #13637 ) ;
#19119=CARTESIAN_POINT ( 'NONE',  ( 3.174475770762294591, -4.645331003335221531, -47.72510079650860604 ) ) ;
#19121=CARTESIAN_POINT ( 'NONE',  ( 10.75185716664280555, 39.99999999999999289, -53.88525272612032069 ) ) ;
#19127=CARTESIAN_POINT ( 'NONE',  ( -18.02527238916006525, 28.84533800490841671, -60.11925852859477004 ) ) ;
#19128=LINE ( 'NONE', #6985, #21059 ) ;
#19130=DIRECTION ( 'NONE',  ( 1.000000000000000000, 0.000000000000000000, 0.000000000000000000 ) ) ;
#19131=DIRECTION ( 'NONE',  ( -0.000000000000000000, 1.000000000000000000, -0.000000000000000000 ) ) ;
#19132=DIRECTION ( 'NONE',  ( -0.000000000000000000, -0.000000000000000000, 1.000000000000000000 ) ) ;
#19133=EDGE_CURVE ( 'NONE', #20269, #7645, #5087, .T. ) ;
#19134=DIRECTION ( 'NONE',  ( -0.000000000000000000, -0.000000000000000000, 1.000000000000000000 ) ) ;
#19135=CARTESIAN_POINT ( 'NONE',  ( -34.99999999999980815, 40.00000000000000000, 52.49999999999922551 ) ) ;
#19145=ADVANCED_FACE ( 'NONE', ( #17317 ), #9892, .F. ) ;
#19146=VERTEX_POINT ( 'NONE', #11721 ) ;
#19148=CARTESIAN_POINT ( 'NONE',  ( 3.001573872049483782, -1.099462678413573036, 50.31569927527682040 ) ) ;
#19151=CIRCLE ( 'NONE', #12194, 14.00000000000000000 ) ;
#19153=CARTESIAN_POINT ( 'NONE',  ( -42.50000000000000711, -12.00000000000000000, 41.00000000000000711 ) ) ;
#19157=ORIENTED_EDGE ( 'NONE', *, *, #775, .F. ) ;
#19158=DIRECTION ( 'NONE',  ( -0.000000000000000000, 1.000000000000000000, -0.000000000000000000 ) ) ;
#19159=VECTOR ( 'NONE', #1181, 1000.000000000000000 ) ;
#19160=CYLINDRICAL_SURFACE ( 'NONE', #16699, 10.00000000000000178 ) ;
#19162=DIRECTION ( 'NONE',  ( -0.000000000000000000, -1.000000000000000000, -0.000000000000000000 ) ) ;
#19163=CARTESIAN_POINT ( 'NONE',  ( -9.455104433789056628, 39.37252125230245525, -54.46735621690890383 ) ) ;
#19165=ORIENTED_EDGE ( 'NONE', *, *, #8006, .T. ) ;
#19167=LINE ( 'NONE', #3474, #4574 ) ;
#19168=EDGE_LOOP ( 'NONE', ( #5426, #13706 ) ) ;
#19171=CARTESIAN_POINT ( 'NONE',  ( 35.00000000000000000, 2.142135623730931471, 4.258610482196280173E-15 ) ) ;
#19173=AXIS2_PLACEMENT_3D ( 'NONE', #15898, #5713, #7202 ) ;
#19175=VERTEX_POINT ( 'NONE', #9990 ) ;
#19182=CARTESIAN_POINT ( 'NONE',  ( 22.30616949375635727, 22.91984106672850174, 58.64191913087365293 ) ) ;
#19184=DIRECTION ( 'NONE',  ( -0.000000000000000000, -1.000000000000000000, -0.000000000000000000 ) ) ;
#19185=CARTESIAN_POINT ( 'NONE',  ( 8.616492322300894457, 39.99999999999999289, 53.19943576118269135 ) ) ;
#19186=ORIENTED_EDGE ( 'NONE', *, *, #21793, .F. ) ;
#19190=DIRECTION ( 'NONE',  ( 0.000000000000000000, 0.000000000000000000, -1.000000000000000000 ) ) ;
#19194=EDGE_CURVE ( 'NONE', #1286, #21483, #21145, .T. ) ;
#19197=DIRECTION ( 'NONE',  ( -0.000000000000000000, -0.000000000000000000, 1.000000000000000000 ) ) ;
#19198=CARTESIAN_POINT ( 'NONE',  ( -1.529841668203881122, 39.98623406166607452, 49.88755235896857698 ) ) ;
#19199=CIRCLE ( 'NONE', #5629, 2.499999999999998668 ) ;
#19200=CARTESIAN_POINT ( 'NONE',  ( -3.591923118226331086E-15, -5.000000000000000000, -44.98888751680799203 ) ) ;
#19205=ORIENTED_EDGE ( 'NONE', *, *, #6633, .T. ) ;
#19208=ORIENTED_EDGE ( 'NONE', *, *, #2984, .T. ) ;
#19210=ORIENTED_EDGE ( 'NONE', *, *, #5601, .T. ) ;
#19214=CARTESIAN_POINT ( 'NONE',  ( -34.99999999999980815, 40.00000000000000711, 52.47499999999922693 ) ) ;
#19215=CARTESIAN_POINT ( 'NONE',  ( 6.501355124432292243, 39.72712729196061332, 53.07780958417031769 ) ) ;
#19216=VERTEX_POINT ( 'NONE', #8738 ) ;
#19218=CARTESIAN_POINT ( 'NONE',  ( -35.00000000000000000, 0.000000000000000000, 1.387778780781445676E-14 ) ) ;
#19219=CARTESIAN_POINT ( 'NONE',  ( 13.00000000000024336, -2.516660498395250745, -100.0000000000000000 ) ) ;
#19223=CARTESIAN_POINT ( 'NONE',  ( -16.96028156848957025, 30.61033039275980627, 59.80781543853676396 ) ) ;
#19225=CARTESIAN_POINT ( 'NONE',  ( 28.49999999999998224, 19.99999999999999645, -105.0000000000000142 ) ) ;
#19226=FACE_OUTER_BOUND ( 'NONE', #11979, .T. ) ;
#19227=VECTOR ( 'NONE', #3366, 1000.000000000000000 ) ;
#19228=ORIENTED_EDGE ( 'NONE', *, *, #4145, .F. ) ;
#19231=B_SPLINE_CURVE_WITH_KNOTS ( 'NONE', 3,
 ( #22692, #12558, #1924, #3546, #1706, #17617, #6979, #9140, #194, #15667, #19461, #8907, #13934, #3764, #19121, #7189, #15881 ),
 .UNSPECIFIED., .F., .F.,
 ( 4, 1, 1, 2, 2, 1, 1, 1, 2, 2, 4 ),
 ( 0.000000000000000000, 0.1250000000000120182, 0.1875000000000164313, 0.2187500000000176803, 0.2500000000000188738, 0.3750000000000237588, 0.4375000000000262568, 0.4687500000000264788, 0.4843750000000252021, 0.5000000000000238698, 1.000000000000000000 ),
 .UNSPECIFIED. ) ;
#19232=ORIENTED_EDGE ( 'NONE', *, *, #17504, .F. ) ;
#19235=CARTESIAN_POINT ( 'NONE',  ( 0.2227364088701092593, -1.232651810761194122, -48.42315971483877490 ) ) ;
#19238=PLANE ( 'NONE',  #14997 ) ;
#19239=ADVANCED_FACE ( 'NONE', ( #466 ), #14318, .T. ) ;
#19240=LINE ( 'NONE', #10508, #12301 ) ;
#19243=CARTESIAN_POINT ( 'NONE',  ( -19.38379237384221554, 24.94684328524662575, -57.98195591854480568 ) ) ;
#19244=VECTOR ( 'NONE', #14256, 1000.000000000000114 ) ;
#19251=CARTESIAN_POINT ( 'NONE',  ( -35.00000000000000000, -4.999999999999997335, 57.00000000000003553 ) ) ;
#19253=CARTESIAN_POINT ( 'NONE',  ( 14.05436202270909796, 14.70285576532228511, -45.40204559108964588 ) ) ;
#19254=AXIS2_PLACEMENT_3D ( 'NONE', #12544, #2020, #15987 ) ;
#19255=VERTEX_POINT ( 'NONE', #12277 ) ;
#19258=AXIS2_PLACEMENT_3D ( 'NONE', #5462, #15761, #12326 ) ;
#19259=ORIENTED_EDGE ( 'NONE', *, *, #19705, .T. ) ;
#19261=AXIS2_PLACEMENT_3D ( 'NONE', #8815, #8702, #12139 ) ;
#19262=ORIENTED_EDGE ( 'NONE', *, *, #3060, .T. ) ;
#19265=CARTESIAN_POINT ( 'NONE',  ( 2.419767991120476136, -3.149022461038316845, 49.02154318835460600 ) ) ;
#19267=CARTESIAN_POINT ( 'NONE',  ( -5.833333333333325932, 40.00000000000000000, 40.61164310337068883 ) ) ;
#19268=ADVANCED_FACE ( 'NONE', ( #17433 ), #5624, .F. ) ;
#19275=DIRECTION ( 'NONE',  ( 0.000000000000000000, 0.000000000000000000, 1.000000000000000000 ) ) ;
#19276=CARTESIAN_POINT ( 'NONE',  ( -15.49999999999980282, -2.516660498395516310, -100.0000000000000000 ) ) ;
#19278=CARTESIAN_POINT ( 'NONE',  ( -9.506747391179116491, 40.00000000000000711, -53.50938557766276915 ) ) ;
#19281=EDGE_CURVE ( 'NONE', #11262, #11081, #9073, .T. ) ;
#19283=CARTESIAN_POINT ( 'NONE',  ( -15.92429324705536864, 4.173694850190172723, 56.88791232810483933 ) ) ;
#19284=AXIS2_PLACEMENT_3D ( 'NONE', #9293, #13044, #18106 ) ;
#19289=EDGE_CURVE ( 'NONE', #8759, #3548, #17125, .T. ) ;
#19290=CIRCLE ( 'NONE', #13394, 2.099999999999990763 ) ;
#19291=EDGE_CURVE ( 'NONE', #21584, #10900, #14881, .T. ) ;
#19292=VERTEX_POINT ( 'NONE', #7691 ) ;
#19295=ORIENTED_EDGE ( 'NONE', *, *, #3309, .T. ) ;
#19300=EDGE_LOOP ( 'NONE', ( #16615, #4645, #19729, #21763 ) ) ;
#19303=ORIENTED_EDGE ( 'NONE', *, *, #21280, .T. ) ;
#19304=CARTESIAN_POINT ( 'NONE',  ( -8.349099696861312481, 1.803277857259543593, 53.93591755799874221 ) ) ;
#19306=CARTESIAN_POINT ( 'NONE',  ( -10.27431133777640149, -4.928932188134504955, 51.43682631505699732 ) ) ;
#19307=EDGE_LOOP ( 'NONE', ( #20833, #14588, #1168, #5098 ) ) ;
#19308=DIRECTION ( 'NONE',  ( 1.000000000000000000, 0.000000000000000000, 0.000000000000000000 ) ) ;
#19309=ORIENTED_EDGE ( 'NONE', *, *, #10883, .F. ) ;
#19310=CARTESIAN_POINT ( 'NONE',  ( -2.278855561005702801E-14, 40.00000000000000000, -48.73397172404479250 ) ) ;
#19311=CARTESIAN_POINT ( 'NONE',  ( 1.387778780781445676E-14, 40.00000000000000000, 48.73397172404482802 ) ) ;
#19312=CARTESIAN_POINT ( 'NONE',  ( -0.5525077609812600876, 39.99819305627858057, 49.15917909279997389 ) ) ;
#19313=VECTOR ( 'NONE', #19073, 1000.000000000000000 ) ;
#19315=CARTESIAN_POINT ( 'NONE',  ( 22.38103533145805102, 18.35979201191610244, 58.65801380639354790 ) ) ;
#19317=AXIS2_PLACEMENT_3D ( 'NONE', #7300, #5487, #12456 ) ;
#19319=EDGE_CURVE ( 'NONE', #13976, #18872, #5425, .T. ) ;
#19320=DIRECTION ( 'NONE',  ( -1.000000000000000000, 0.000000000000000000, 0.000000000000000000 ) ) ;
#19321=ORIENTED_EDGE ( 'NONE', *, *, #21221, .F. ) ;
#19322=AXIS2_PLACEMENT_3D ( 'NONE', #20102, #14589, #11151 ) ;
#19326=EDGE_LOOP ( 'NONE', ( #9866, #19063, #12032, #12494 ) ) ;
#19327=DIRECTION ( 'NONE',  ( -0.000000000000000000, 1.000000000000000000, -0.000000000000000000 ) ) ;
#19329=VECTOR ( 'NONE', #89, 1000.000000000000000 ) ;
#19333=CARTESIAN_POINT ( 'NONE',  ( 0.5323810940973144890, 39.99832332085551201, 49.14386465755924149 ) ) ;
#19335=FACE_OUTER_BOUND ( 'NONE', #18460, .T. ) ;
#19340=EDGE_CURVE ( 'NONE', #6067, #4414, #10069, .T. ) ;
#19343=AXIS2_PLACEMENT_3D ( 'NONE', #7036, #8974, #19308 ) ;
#19344=CARTESIAN_POINT ( 'NONE',  ( -6.433485051968491852, 38.94088993357631523, 55.16018527339316080 ) ) ;
#19345=DIRECTION ( 'NONE',  ( 0.000000000000000000, 0.000000000000000000, 1.000000000000000000 ) ) ;
#19348=VECTOR ( 'NONE', #8999, 1000.000000000000000 ) ;
#19351=VERTEX_POINT ( 'NONE', #21879 ) ;
#19354=VECTOR ( 'NONE', #4948, 1000.000000000000000 ) ;
#19355=DIRECTION ( 'NONE',  ( -0.000000000000000000, -1.000000000000000000, -0.000000000000000000 ) ) ;
#19356=EDGE_CURVE ( 'NONE', #14756, #15733, #11277, .T. ) ;
#19361=CARTESIAN_POINT ( 'NONE',  ( 42.50000000000000711, -12.00000000000012434, 50.02500000000011937 ) ) ;
#19362=CARTESIAN_POINT ( 'NONE',  ( -17.16827611621724969, 34.47540479398168856, -57.28984973304980599 ) ) ;
#19363=VECTOR ( 'NONE', #22374, 1000.000000000000000 ) ;
#19366=EDGE_LOOP ( 'NONE', ( #58, #3562 ) ) ;
#19368=LINE ( 'NONE', #2390, #15465 ) ;
#19369=FACE_BOUND ( 'NONE', #15926, .T. ) ;
#19370=CARTESIAN_POINT ( 'NONE',  ( 14.99999999999998579, 19.22713695939443568, -45.82575694955836809 ) ) ;
#19371=VERTEX_POINT ( 'NONE', #12910 ) ;
#19374=CARTESIAN_POINT ( 'NONE',  ( -35.00000000000000000, 2.142135623730931471, 1.387778780781445676E-14 ) ) ;
#19377=EDGE_LOOP ( 'NONE', ( #3990, #5527, #21144, #3656, #8932, #17313, #1225 ) ) ;
#19380=CARTESIAN_POINT ( 'NONE',  ( 0.1620509895534447964, 39.99984822922976946, -48.85971511756937247 ) ) ;
#19381=DIRECTION ( 'NONE',  ( -0.000000000000000000, -1.000000000000000000, -0.000000000000000000 ) ) ;
#19383=CARTESIAN_POINT ( 'NONE',  ( -10.49999999999980282, -2.516660498395516310, 105.0000000000000142 ) ) ;
#19384=ORIENTED_EDGE ( 'NONE', *, *, #15572, .F. ) ;
#19385=CARTESIAN_POINT ( 'NONE',  ( -34.99999999999999289, 40.00000000000000000, -51.00000000000000711 ) ) ;
#19386=CARTESIAN_POINT ( 'NONE',  ( -9.952189117650803496, 40.00000000000000000, 53.64426396172073908 ) ) ;
#19388=DIRECTION ( 'NONE',  ( -0.000000000000000000, -0.000000000000000000, 1.000000000000000000 ) ) ;
#19393=DIRECTION ( 'NONE',  ( 0.000000000000000000, 1.000000000000000000, 0.000000000000000000 ) ) ;
#19395=CARTESIAN_POINT ( 'NONE',  ( -2.244030815477592533, 39.96966515101875217, -50.39883272053734231 ) ) ;
#19397=CARTESIAN_POINT ( 'NONE',  ( 11.68090480754630001, 3.765577839755386957, 57.90797000640142755 ) ) ;
#19398=DIRECTION ( 'NONE',  ( 0.000000000000000000, 0.000000000000000000, 1.000000000000000000 ) ) ;
#19402=ORIENTED_EDGE ( 'NONE', *, *, #4105, .T. ) ;
#19403=ORIENTED_EDGE ( 'NONE', *, *, #2232, .F. ) ;
#19407=ADVANCED_FACE ( 'NONE', ( #11666 ), #7617, .F. ) ;
#19410=CARTESIAN_POINT ( 'NONE',  ( 15.37127427991059392, 36.37761751580015357, 56.70227746889294451 ) ) ;
#19412=CARTESIAN_POINT ( 'NONE',  ( 9.454383690904577975, 39.37264121342599310, -54.46710214104096792 ) ) ;
#19413=CARTESIAN_POINT ( 'NONE',  ( 9.193775052642715551, 40.00000000000000711, 53.40447181116137898 ) ) ;
#19415=CARTESIAN_POINT ( 'NONE',  ( -1.387778780781445518E-14, 20.00000000000000355, 105.0000000000000142 ) ) ;
#19416=CARTESIAN_POINT ( 'NONE',  ( 6.696867368504048330E-15, 5.000000000000000888, 38.73397172404480671 ) ) ;
#19417=ORIENTED_EDGE ( 'NONE', *, *, #10148, .F. ) ;
#19422=CARTESIAN_POINT ( 'NONE',  ( 6.976853941385730451, 1.175947842330679061, 53.23020196600168674 ) ) ;
#19426=CARTESIAN_POINT ( 'NONE',  ( -0.1539325450100966219, 40.00000000000000711, 48.91834387730083478 ) ) ;
#19427=CARTESIAN_POINT ( 'NONE',  ( 42.50000000000000711, -11.97499999999999964, 45.00000000000000711 ) ) ;
#19429=CARTESIAN_POINT ( 'NONE',  ( 19.42731605662046235, 15.16896271047388822, 57.99434643147303348 ) ) ;
#19436=EDGE_LOOP ( 'NONE', ( #3724, #18912, #8415, #14011, #18844, #22020, #15134 ) ) ;
#19442=CARTESIAN_POINT ( 'NONE',  ( 0.01336081163439876984, 39.99999903713349880, 48.74437065933960156 ) ) ;
#19447=CARTESIAN_POINT ( 'NONE',  ( 12.82970538955578022, 1.687462484003134255, -55.75926248610264224 ) ) ;
#19453=AXIS2_PLACEMENT_3D ( 'NONE', #3057, #4673, #6379 ) ;
#19455=DIRECTION ( 'NONE',  ( -0.000000000000000000, -0.000000000000000000, 1.000000000000000000 ) ) ;
#19457=ORIENTED_EDGE ( 'NONE', *, *, #11414, .F. ) ;
#19460=CARTESIAN_POINT ( 'NONE',  ( 0.7217013448888215388, -4.626342591370756985, -46.01887142925446739 ) ) ;
#19461=CARTESIAN_POINT ( 'NONE',  ( 11.19713514086473438, 39.99999999999999289, -54.03748032825708236 ) ) ;
#19464=CARTESIAN_POINT ( 'NONE',  ( -90.00000000000000000, 40.00000000000000000, 2.099999999999989875 ) ) ;
#19465=CARTESIAN_POINT ( 'NONE',  ( -13.09671971564483073, 38.20119746052779419, -55.86054988736573534 ) ) ;
#19469=FACE_OUTER_BOUND ( 'NONE', #7842, .T. ) ;
#19471=FACE_BOUND ( 'NONE', #7869, .T. ) ;
#19472=CARTESIAN_POINT ( 'NONE',  ( 9.579024991657044907, 8.451577327321118105, -43.05667825653225123 ) ) ;
#19477=DIRECTION ( 'NONE',  ( -0.000000000000000000, -1.000000000000000000, -0.000000000000000000 ) ) ;
#19480=ADVANCED_FACE ( 'NONE', ( #1695, #3650 ), #21052, .T. ) ;
#19482=CARTESIAN_POINT ( 'NONE',  ( 0.04635509897966557519, 40.00000000000001421, -48.77005890240622676 ) ) ;
#19484=CARTESIAN_POINT ( 'NONE',  ( 90.00000000000000000, 26.00000000000000355, 2.099999999999989875 ) ) ;
#19488=CARTESIAN_POINT ( 'NONE',  ( -8.421829293842984399, 39.99999999999998579, 53.12761752185808461 ) ) ;
#19491=CARTESIAN_POINT ( 'NONE',  ( 22.15746142094439719, 16.52917608750723488, -58.60949679988861050 ) ) ;
#19492=CIRCLE ( 'NONE', #15807, 2.099999999999997868 ) ;
#19494=CARTESIAN_POINT ( 'NONE',  ( 15.50000000000024336, -2.516660498395250301, -105.0000000000000142 ) ) ;
#19497=CARTESIAN_POINT ( 'NONE',  ( -10.31465995609392827, 2.846668092513518378, 57.27881138849647868 ) ) ;
#19498=CARTESIAN_POINT ( 'NONE',  ( -6.718896912932006416, 39.70714865612620059, -53.19564684132798504 ) ) ;
#19502=DIRECTION ( 'NONE',  ( 0.000000000000000000, -1.000000000000000000, 0.000000000000000000 ) ) ;
#19506=CIRCLE ( 'NONE', #18772, 2.499999999999995115 ) ;
#19508=VERTEX_POINT ( 'NONE', #11177 ) ;
#19509=VECTOR ( 'NONE', #7239, 1000.000000000000000 ) ;
#19510=ORIENTED_EDGE ( 'NONE', *, *, #11211, .F. ) ;
#19512=CARTESIAN_POINT ( 'NONE',  ( -35.00000000000000000, -5.000000000000000000, 1.387778780781445676E-14 ) ) ;
#19516=DIRECTION ( 'NONE',  ( -1.000000000000000000, 0.000000000000000000, 0.000000000000000000 ) ) ;
#19518=ORIENTED_EDGE ( 'NONE', *, *, #4668, .F. ) ;
#19520=CARTESIAN_POINT ( 'NONE',  ( -15.37127427991062056, 36.37761751580014646, -56.70227746889291609 ) ) ;
#19522=ORIENTED_EDGE ( 'NONE', *, *, #10857, .T. ) ;
#19524=FACE_OUTER_BOUND ( 'NONE', #6922, .T. ) ;
#19525=EDGE_LOOP ( 'NONE', ( #16925, #11730, #10445, #15339 ) ) ;
#19532=CARTESIAN_POINT ( 'NONE',  ( 19.67353980729958352, 23.69994786804610953, 58.06093965454051897 ) ) ;
#19538=ORIENTED_EDGE ( 'NONE', *, *, #2720, .F. ) ;
#19540=ORIENTED_EDGE ( 'NONE', *, *, #7770, .T. ) ;
#19545=DIRECTION ( 'NONE',  ( -0.000000000000000000, -1.000000000000000000, -0.000000000000000000 ) ) ;
#19546=DIRECTION ( 'NONE',  ( 0.000000000000000000, 0.000000000000000000, -1.000000000000000000 ) ) ;
#19547=DIRECTION ( 'NONE',  ( -0.000000000000000000, 1.000000000000000000, -0.000000000000000000 ) ) ;
#19550=CARTESIAN_POINT ( 'NONE',  ( 6.687085176834780320, 39.71011800170725792, 53.17853448240479963 ) ) ;
#19554=CARTESIAN_POINT ( 'NONE',  ( 42.50000000000000711, -12.00000000000000000, 47.50000000000000711 ) ) ;
#19555=DIRECTION ( 'NONE',  ( 1.049727191138617217E-16, 0.5150380749100562650, -0.8571673007021111124 ) ) ;
#19557=DIRECTION ( 'NONE',  ( -0.000000000000000000, 1.000000000000000000, -0.000000000000000000 ) ) ;
#19558=CONICAL_SURFACE ( 'NONE', #8217, 2.099999999999997868, 1.029744258676652091 ) ;
#19565=ORIENTED_EDGE ( 'NONE', *, *, #12979, .F. ) ;
#19566=EDGE_CURVE ( 'NONE', #14798, #15385, #9137, .T. ) ;
#19570=CARTESIAN_POINT ( 'NONE',  ( 90.00000000000000000, 40.00000000000000711, -9.108981535246192915E-16 ) ) ;
#19573=FACE_OUTER_BOUND ( 'NONE', #7069, .T. ) ;
#19575=CARTESIAN_POINT ( 'NONE',  ( -12.89955995983995507, 4.696256998628602020, 58.40693116658150785 ) ) ;
#19576=CARTESIAN_POINT ( 'NONE',  ( -13.73196689449470220, 34.57679379660266505, -56.13071196757329062 ) ) ;
#19579=FACE_BOUND ( 'NONE', #465, .T. ) ;
#19580=CARTESIAN_POINT ( 'NONE',  ( -6.775279300855757469, 38.82186504314599773, -55.41168644275258259 ) ) ;
#19582=CARTESIAN_POINT ( 'NONE',  ( 5.833333333333437842, 6.180730040185884455, -40.61164310337073857 ) ) ;
#19586=CARTESIAN_POINT ( 'NONE',  ( -15.49999999999980282, -2.516660498395515866, -105.0010000000000048 ) ) ;
#19589=DIRECTION ( 'NONE',  ( -0.000000000000000000, -0.000000000000000000, 1.000000000000000000 ) ) ;
#19593=CIRCLE ( 'NONE', #3513, 2.000000000000002665 ) ;
#19599=VERTEX_POINT ( 'NONE', #20106 ) ;
#19601=CARTESIAN_POINT ( 'NONE',  ( -8.657949774411953570, 40.00000000000000711, 53.21471414886531193 ) ) ;
#19606=CARTESIAN_POINT ( 'NONE',  ( 15.92429324705532245, 4.173694850190156735, -56.88791232810482512 ) ) ;
#19607=AXIS2_PLACEMENT_3D ( 'NONE', #16356, #6278, #6389 ) ;
#19609=VERTEX_POINT ( 'NONE', #4826 ) ;
#19611=CARTESIAN_POINT ( 'NONE',  ( -1.619914140209613773, 39.98468592336024585, -49.95346900270995150 ) ) ;
#19612=ORIENTED_EDGE ( 'NONE', *, *, #5686, .T. ) ;
#19613=CARTESIAN_POINT ( 'NONE',  ( 12.27586057105636108, 4.193657236093890184, 55.54740530680977884 ) ) ;
#19621=VECTOR ( 'NONE', #11669, 1000.000000000000000 ) ;
#19626=DIRECTION ( 'NONE',  ( 0.000000000000000000, 0.000000000000000000, -1.000000000000000000 ) ) ;
#19628=CARTESIAN_POINT ( 'NONE',  ( 5.233858753929546914, 39.99999999999999289, -51.72875402900091757 ) ) ;
#19629=CARTESIAN_POINT ( 'NONE',  ( 6.286720829167179225, 40.00000000000000711, 52.22859680466056176 ) ) ;
#19632=DIRECTION ( 'NONE',  ( 0.000000000000000000, 0.000000000000000000, -1.000000000000000000 ) ) ;
#19633=EDGE_LOOP ( 'NONE', ( #13312, #19186, #7128, #12306 ) ) ;
#19638=EDGE_CURVE ( 'NONE', #22194, #3413, #17289, .T. ) ;
#19639=CARTESIAN_POINT ( 'NONE',  ( -22.42346072916788557, 20.15694599340442394, -58.66711769948890520 ) ) ;
#19644=CARTESIAN_POINT ( 'NONE',  ( 0.6844983420862013057, -1.267142481716289959, 48.72692999687993876 ) ) ;
#19652=CARTESIAN_POINT ( 'NONE',  ( 18.88991738967228429, 26.58741517403858268, 57.84428223557716819 ) ) ;
#19653=DIRECTION ( 'NONE',  ( 3.525918314278899701E-15, 0.000000000000000000, 1.000000000000000000 ) ) ;
#19654=CARTESIAN_POINT ( 'NONE',  ( 13.10473755708325250, 38.28578281281944129, -55.88243319222879535 ) ) ;
#19655=CIRCLE ( 'NONE', #3186, 6.499999999999999112 ) ;
#19657=ORIENTED_EDGE ( 'NONE', *, *, #2636, .F. ) ;
#19661=CARTESIAN_POINT ( 'NONE',  ( -35.00000000000000000, 40.00000000000000000, 1.387778780781445676E-14 ) ) ;
#19666=CARTESIAN_POINT ( 'NONE',  ( -12.24744603029288292, 40.00000000000000000, -54.43639671998465701 ) ) ;
#19667=FACE_OUTER_BOUND ( 'NONE', #20994, .T. ) ;
#19668=ADVANCED_FACE ( 'NONE', ( #16954 ), #8255, .T. ) ;
#19673=LINE ( 'NONE', #12434, #289 ) ;
#19680=CIRCLE ( 'NONE', #17836, 10.00000000000000000 ) ;
#19686=B_SPLINE_CURVE_WITH_KNOTS ( 'NONE', 3,
 ( #18652, #6846, #2959, #10147, #4898, #8552, #5133, #1459, #8669, #8219, #15181, #4790, #8332, #5015, #6499, #20373, #10035, #13465, #3409, #11995, #17366, #1339, #11761, #15305, #8445, #1687, #15648, #22430, #20484, #22328, #15526, #18995, #3183, #20588, #11874, #3302, #18758, #6612, #13574, #17143, #6726, #17254, #5562, #21697, #3526, #8789, #2018, #6962, #5994 ),
 .UNSPECIFIED., .F., .F.,
 ( 4, 1, 1, 1, 2, 2, 1, 1, 1, 1, 2, 2, 1, 1, 1, 2, 2, 1, 1, 1, 1, 2, 2, 1, 1, 1, 1, 2, 2, 1, 1, 1, 2, 2, 4 ),
 ( 0.000000000000000000, 0.1249999999999849842, 0.1874999999999770184, 0.2187499999999730216, 0.2343749999999715228, 0.2499999999999700240, 0.3749999999999616973, 0.4374999999999579781, 0.4687499999999561462, 0.4843749999999556466, 0.4921874999999552580, 0.4999999999999549249, 0.5624999999999592548, 0.5937499999999615863, 0.6093749999999631406, 0.6171874999999638067, 0.6249999999999645839, 0.6874999999999683586, 0.7187499999999701350, 0.7343749999999714673, 0.7421874999999721334, 0.7460937499999724665, 0.7499999999999726885, 0.8124999999999790168, 0.8437499999999827915, 0.8593749999999849010, 0.8671874999999857891, 0.8710937499999861222, 0.8749999999999865663, 0.9062499999999896749, 0.9218749999999912292, 0.9296874999999918954, 0.9335937499999925615, 0.9374999999999932276, 1.000000000000000000 ),
 .UNSPECIFIED. ) ;
#19688=AXIS2_PLACEMENT_3D ( 'NONE', #2864, #17049, #8130 ) ;
#19696=( BOUNDED_SURFACE ( )  B_SPLINE_SURFACE ( 3, 2, ( 
 ( #15766, #20839, #10379 ),
 ( #5357, #12114, #10494 ),
 ( #17496, #19111, #3416 ),
 ( #76, #7064, #14030 ),
 ( #21053, #12334, #19344 ),
 ( #3651, #20131, #3986 ),
 ( #6150, #21732, #6033 ),
 ( #16218, #10955, #16458 ),
 ( #17948, #14831, #13118 ),
 ( #5808, #4436, #4206 ),
 ( #9235, #14613, #16565 ),
 ( #11409, #14718, #5688 ),
 ( #21854, #869, #11065 ),
 ( #21504, #12779, #7862 ) ),
 .UNSPECIFIED., .F., .F., .T. ) 
 B_SPLINE_SURFACE_WITH_KNOTS ( ( 4, 2, 2, 2, 2, 2, 4 ),
 ( 3, 3 ),
 ( 0.004259382447192460938, 0.005809352080732368973, 0.007359321714272276140, 0.008909291347812183307, 0.01045926098135209134, 0.01355920024843190741, 0.01665913951551172348 ),
 ( 0.1636470045611256030, 1.000000000000000000 ),
 .UNSPECIFIED. ) 
 GEOMETRIC_REPRESENTATION_ITEM ( )  RATIONAL_B_SPLINE_SURFACE ( (
 ( 0.9022249821884000820, 0.7012624274003163016, 1.000000000000000000),
 ( 0.9123788763119136114, 0.7322861975901361342, 1.000000000000000000),
 ( 0.9211843504036706376, 0.7591900633693231537, 1.000000000000000000),
 ( 0.9369236066439512456, 0.8072791080863062074, 1.000000000000000000),
 ( 0.9438541764422034852, 0.8284544721476249096, 1.000000000000000000),
 ( 0.9562659320682393993, 0.8663768149956418974, 1.000000000000000000),
 ( 0.9617548100769197639, 0.8831472961401047872, 1.000000000000000000),
 ( 0.9714485269178145810, 0.9127650605070476431, 1.000000000000000000),
 ( 0.9756421407944039226, 0.9255780474842177918, 1.000000000000000000),
 ( 0.9865759213550759910, 0.9589846490593422201, 1.000000000000000000),
 ( 0.9916869380071704487, 0.9746006289112230103, 1.000000000000000000),
 ( 0.9984050399869064396, 0.9951268279631179103, 1.000000000000000000),
 ( 0.9999940432348444208, 0.9999817999566460447, 1.000000000000000000),
 ( 1.000000000000000000, 1.000000000000000000, 1.000000000000000000) ) ) 
 REPRESENTATION_ITEM ( '' )  SURFACE ( )  );
#19699=CARTESIAN_POINT ( 'NONE',  ( -13.83098800442514253, 37.66187182509482057, -56.14292165594078909 ) ) ;
#19705=EDGE_CURVE ( 'NONE', #10027, #249, #16142, .T. ) ;
#19709=VECTOR ( 'NONE', #1903, 1000.000000000000114 ) ;
#19710=ORIENTED_EDGE ( 'NONE', *, *, #9879, .T. ) ;
#19712=ORIENTED_EDGE ( 'NONE', *, *, #19026, .F. ) ;
#19714=CARTESIAN_POINT ( 'NONE',  ( 25.99999999999998579, 19.99999999999999645, 100.0000000000000000 ) ) ;
#19715=CARTESIAN_POINT ( 'NONE',  ( 12.27586057105635042, 4.193657236093891960, -55.54740530680976462 ) ) ;
#19716=APPLICATION_CONTEXT ( 'automotive_design' ) ;
#19721=CIRCLE ( 'NONE', #15675, 49.99999999999998579 ) ;
#19725=CARTESIAN_POINT ( 'NONE',  ( 35.00000000000000000, -5.000000000000000888, 18.00000000000000711 ) ) ;
#19729=ORIENTED_EDGE ( 'NONE', *, *, #9477, .T. ) ;
#19732=EDGE_CURVE ( 'NONE', #790, #9501, #3260, .T. ) ;
#19733=LINE ( 'NONE', #14425, #7516 ) ;
#19735=CARTESIAN_POINT ( 'NONE',  ( 5.833333333333328596, 33.81926995981416439, -40.61164310337066041 ) ) ;
#19739=CIRCLE ( 'NONE', #5817, 2.525000000000110489 ) ;
#19741=VERTEX_POINT ( 'NONE', #6383 ) ;
#19743=DIRECTION ( 'NONE',  ( -0.000000000000000000, 1.000000000000000000, -0.000000000000000000 ) ) ;
#19744=VERTEX_POINT ( 'NONE', #12821 ) ;
#19745=ORIENTED_EDGE ( 'NONE', *, *, #16684, .T. ) ;
#19751=CARTESIAN_POINT ( 'NONE',  ( 7.471708243917213110, 39.63177981526567351, -53.58785989103921565 ) ) ;
#19757=CARTESIAN_POINT ( 'NONE',  ( 0.05268221300119596551, -1.234065601521194377, 48.20433757654415530 ) ) ;
#19762=CARTESIAN_POINT ( 'NONE',  ( 5.340789179572191792, 39.27722415257183286, 54.28402915905950010 ) ) ;
#19767=CARTESIAN_POINT ( 'NONE',  ( 19.61594976190319528, 16.00511159616338830, 58.04523854797174920 ) ) ;
#19769=DIRECTION ( 'NONE',  ( 0.000000000000000000, -1.000000000000000000, 0.000000000000000000 ) ) ;
#19776=DIRECTION ( 'NONE',  ( 0.000000000000000000, 0.000000000000000000, -1.000000000000000000 ) ) ;
#19777=CARTESIAN_POINT ( 'NONE',  ( -9.689843208404459673, 39.33333333333334991, -54.54983754392748807 ) ) ;
#19778=ADVANCED_FACE ( 'NONE', ( #9707 ), #2958, .F. ) ;
#19779=PLANE ( 'NONE',  #21997 ) ;
#19781=VERTEX_POINT ( 'NONE', #1000 ) ;
#19783=CARTESIAN_POINT ( 'NONE',  ( -1.583519045123022995, -4.618580011808621322, 46.65783332780200254 ) ) ;
#19784=VERTEX_POINT ( 'NONE', #21983 ) ;
#19791=LINE ( 'NONE', #18176, #126 ) ;
#19794=ORIENTED_EDGE ( 'NONE', *, *, #12786, .T. ) ;
#19795=ORIENTED_EDGE ( 'NONE', *, *, #16315, .T. ) ;
#19800=VECTOR ( 'NONE', #10566, 1000.000000000000000 ) ;
#19802=CARTESIAN_POINT ( 'NONE',  ( 3.711307361476188671, -1.139702956418044089, -50.71376883234283639 ) ) ;
#19803=CARTESIAN_POINT ( 'NONE',  ( 0.3107847162787464868, 39.99819769545531756, 49.10452103004165281 ) ) ;
#19805=CARTESIAN_POINT ( 'NONE',  ( 8.479740367036404436, -4.901256658985633230, 50.57596245086651265 ) ) ;
#19809=ORIENTED_EDGE ( 'NONE', *, *, #20783, .F. ) ;
#19810=DIRECTION ( 'NONE',  ( 0.000000000000000000, 0.000000000000000000, 1.000000000000000000 ) ) ;
#19811=DIRECTION ( 'NONE',  ( 0.000000000000000000, 0.000000000000000000, 1.000000000000000000 ) ) ;
#19814=DIRECTION ( 'NONE',  ( 0.000000000000000000, 0.000000000000000000, 1.000000000000000000 ) ) ;
#19818=DIRECTION ( 'NONE',  ( 0.000000000000000000, 0.000000000000000000, 1.000000000000000000 ) ) ;
#19821=CARTESIAN_POINT ( 'NONE',  ( 23.49999999999998579, 19.99999999999999645, 100.0000000000000000 ) ) ;
#19826=CARTESIAN_POINT ( 'NONE',  ( 4.592961669381029566, 39.86863535336818387, -51.95971364930980485 ) ) ;
#19828=DIRECTION ( 'NONE',  ( -0.000000000000000000, 1.000000000000000000, -0.000000000000000000 ) ) ;
#19831=EDGE_CURVE ( 'NONE', #19175, #15847, #16044, .T. ) ;
#19832=CARTESIAN_POINT ( 'NONE',  ( -9.952189117650803496, 40.00000000000000000, 53.64426396172073908 ) ) ;
#19836=CARTESIAN_POINT ( 'NONE',  ( -7.763906758555455312, 40.00000000000000711, 52.86922912568341104 ) ) ;
#19837=LINE ( 'NONE', #11006, #11508 ) ;
#19838=EDGE_CURVE ( 'NONE', #21010, #14794, #17507, .T. ) ;
#19840=CARTESIAN_POINT ( 'NONE',  ( 10.27431133777207961, -4.928932188134511172, 51.43682631505490832 ) ) ;
#19841=CARTESIAN_POINT ( 'NONE',  ( -5.249999999999978684, 40.00000000000000000, 41.42387596543811412 ) ) ;
#19842=CARTESIAN_POINT ( 'NONE',  ( -6.877234595577741416, 39.69228527894571812, -53.28061377157573020 ) ) ;
#19844=DIRECTION ( 'NONE',  ( -1.000000000000000000, 0.000000000000000000, 0.000000000000000000 ) ) ;
#19845=AXIS2_PLACEMENT_3D ( 'NONE', #9066, #14661, #14196 ) ;
#19846=DIRECTION ( 'NONE',  ( 0.000000000000000000, 0.000000000000000000, -1.000000000000000000 ) ) ;
#19854=CYLINDRICAL_SURFACE ( 'NONE', #14885, 2.499999999999995115 ) ;
#19858=CARTESIAN_POINT ( 'NONE',  ( -20.00000000000001421, 20.00000000000000000, -60.62177826491068799 ) ) ;
#19859=ORIENTED_EDGE ( 'NONE', *, *, #10237, .T. ) ;
#19862=ORIENTED_EDGE ( 'NONE', *, *, #8149, .T. ) ;
#19867=CARTESIAN_POINT ( 'NONE',  ( 3.711307361474756927, -1.139702956417446567, 50.71376883234223953 ) ) ;
#19869=CARTESIAN_POINT ( 'NONE',  ( 8.234867195337331580, 38.24532286050943952, 54.56733378486904229 ) ) ;
#19870=DIRECTION ( 'NONE',  ( -1.000000000000000000, 0.000000000000000000, 0.000000000000000000 ) ) ;
#19873=CYLINDRICAL_SURFACE ( 'NONE', #15822, 2.499999999999998668 ) ;
#19874=FACE_BOUND ( 'NONE', #284, .T. ) ;
#19878=ORIENTED_EDGE ( 'NONE', *, *, #18092, .F. ) ;
#19879=VERTEX_POINT ( 'NONE', #11994 ) ;
#19881=CARTESIAN_POINT ( 'NONE',  ( -10.87562399016030135, 39.15903841217814829, -54.97094722855624127 ) ) ;
#19886=CONICAL_SURFACE ( 'NONE', #18785, 2.099999999999990763, 1.029744258676652091 ) ;
#19888=CARTESIAN_POINT ( 'NONE',  ( 11.86180952234342278, 38.99999999999291589, -55.35904751185374550 ) ) ;
#19890=DIRECTION ( 'NONE',  ( 1.049727191138617217E-16, 0.5150380749100562650, -0.8571673007021111124 ) ) ;
#19891=DIRECTION ( 'NONE',  ( -0.000000000000000000, -1.000000000000000000, -0.000000000000000000 ) ) ;
#19892=CIRCLE ( 'NONE', #15104, 2.099999999999997868 ) ;
#19897=FACE_OUTER_BOUND ( 'NONE', #13121, .T. ) ;
#19899=VERTEX_POINT ( 'NONE', #18757 ) ;
#19900=CIRCLE ( 'NONE', #10363, 2.500000000000002220 ) ;
#19903=TOROIDAL_SURFACE ( 'NONE', #130, 50.00000000000000000, 10.00000000000000000 ) ;
#19906=DIRECTION ( 'NONE',  ( 0.000000000000000000, -1.000000000000000000, 0.000000000000000000 ) ) ;
#19907=CARTESIAN_POINT ( 'NONE',  ( 1.801771875245271604, 0.06844342149321584745, -51.82845797840088409 ) ) ;
#19909=CARTESIAN_POINT ( 'NONE',  ( 6.401904815323814724, 38.95163572918602313, 55.13655742298573870 ) ) ;
#19910=LINE ( 'NONE', #10240, #2144 ) ;
#19911=CARTESIAN_POINT ( 'NONE',  ( -7.555723902514296597, 38.52224445567478028, -55.93227658743224850 ) ) ;
#19914=FACE_OUTER_BOUND ( 'NONE', #1188, .T. ) ;
#19917=ORIENTED_EDGE ( 'NONE', *, *, #18017, .F. ) ;
#19919=CARTESIAN_POINT ( 'NONE',  ( -5.302825731643218354, 39.28770244913256704, -54.25167596405762538 ) ) ;
#19924=CARTESIAN_POINT ( 'NONE',  ( 12.99999999999993960, 42.51666049839543149, 60.00099999999999767 ) ) ;
#19926=DIRECTION ( 'NONE',  ( 0.000000000000000000, 0.000000000000000000, 1.000000000000000000 ) ) ;
#19930=FACE_OUTER_BOUND ( 'NONE', #18890, .T. ) ;
#19933=ORIENTED_EDGE ( 'NONE', *, *, #15340, .F. ) ;
#19934=CARTESIAN_POINT ( 'NONE',  ( 1.529876220499305495, 39.98623341753695115, -49.88757757837743867 ) ) ;
#19936=VERTEX_POINT ( 'NONE', #13687 ) ;
#19938=FACE_OUTER_BOUND ( 'NONE', #2846, .T. ) ;
#19942=CARTESIAN_POINT ( 'NONE',  ( -4.407759405548853593, 40.00000000000000711, 51.31071847168679767 ) ) ;
#19943=DIRECTION ( 'NONE',  ( -0.000000000000000000, -1.000000000000000000, -0.000000000000000000 ) ) ;
#19945=DIRECTION ( 'NONE',  ( -1.000000000000000000, 0.000000000000000000, 0.000000000000000000 ) ) ;
#19946=AXIS2_PLACEMENT_3D ( 'NONE', #18663, #22217, #10272 ) ;
#19947=CARTESIAN_POINT ( 'NONE',  ( -11.00126833636917034, 3.276569432483635413, 57.62199738645403357 ) ) ;
#19954=VERTEX_POINT ( 'NONE', #17028 ) ;
#19955=AXIS2_PLACEMENT_3D ( 'NONE', #15676, #8811, #5263 ) ;
#19957=ADVANCED_FACE ( 'NONE', ( #17253 ), #9109, .F. ) ;
#19958=B_SPLINE_CURVE_WITH_KNOTS ( 'NONE', 3,
 ( #14841, #6043, #12790, #5928, #19909, #6276, #8112, #20256, #11190, #1001, #2729, #13009, #8001, #14960, #21984, #19803, #4215, #18188 ),
 .UNSPECIFIED., .F., .F.,
 ( 4, 2, 2, 2, 2, 2, 2, 2, 4 ),
 ( 0.000000000000000000, 0.001465012583164692446, 0.002930025166329384891, 0.004395037749494077120, 0.005860050332658769782, 0.008790075498988142097, 0.01025508808215282695, 0.01098759437373516244, 0.01172010066531749793 ),
 .UNSPECIFIED. ) ;
#19959=ORIENTED_EDGE ( 'NONE', *, *, #16392, .T. ) ;
#19961=ORIENTED_EDGE ( 'NONE', *, *, #18233, .T. ) ;
#19962=CARTESIAN_POINT ( 'NONE',  ( 19.62614308895799908, 23.87978888144414924, -60.53224704373669596 ) ) ;
#19967=DIRECTION ( 'NONE',  ( -0.000000000000000000, -0.000000000000000000, 1.000000000000000000 ) ) ;
#19971=ORIENTED_EDGE ( 'NONE', *, *, #15348, .T. ) ;
#19974=CARTESIAN_POINT ( 'NONE',  ( -10.38220159744133575, 9.149172668433822153, -43.52345836121335765 ) ) ;
#19976=CARTESIAN_POINT ( 'NONE',  ( -21.56999872847277544, 13.83083564369840701, -58.47776649573036423 ) ) ;
#19977=DIRECTION ( 'NONE',  ( 0.000000000000000000, 0.000000000000000000, 1.000000000000000000 ) ) ;
#19979=CARTESIAN_POINT ( 'NONE',  ( 35.00000000000058265, 28.00000000000000000, -52.90000000000076597 ) ) ;
#19980=CARTESIAN_POINT ( 'NONE',  ( 4.664549341139660577, 0.4975632029829551994, 53.81030450292042389 ) ) ;
#19982=CARTESIAN_POINT ( 'NONE',  ( 3.981142735421731249, 39.90683062736657405, 51.58240146861697184 ) ) ;
#19984=DIRECTION ( 'NONE',  ( -0.000000000000000000, -1.000000000000000000, -0.000000000000000000 ) ) ;
#19985=CARTESIAN_POINT ( 'NONE',  ( -42.50000000000000711, -5.000000000000000000, 45.40000000000001279 ) ) ;
#19986=AXIS2_PLACEMENT_3D ( 'NONE', #11850, #22182, #15160 ) ;
#19989=CARTESIAN_POINT ( 'NONE',  ( 11.57708680448565097, 39.19108614651868550, 55.24531487870351754 ) ) ;
#19992=CIRCLE ( 'NONE', #15215, 2.499999999999998668 ) ;
#19993=DIRECTION ( 'NONE',  ( -0.8171172023792284689, 0.3308262969263051634, -0.4720947350246256224 ) ) ;
#19994=VERTEX_POINT ( 'NONE', #8888 ) ;
#19995=ORIENTED_EDGE ( 'NONE', *, *, #8147, .T. ) ;
#19998=CONICAL_SURFACE ( 'NONE', #3547, 57.00000000000002132, 0.7853981633974437271 ) ;
#19999=ORIENTED_EDGE ( 'NONE', *, *, #9014, .T. ) ;
#20000=CARTESIAN_POINT ( 'NONE',  ( -42.50000000000000711, -5.000000000000000000, -47.50000000000000000 ) ) ;
#20011=CARTESIAN_POINT ( 'NONE',  ( 35.00000000000000000, 40.00000000000000000, 4.258610482196280173E-15 ) ) ;
#20013=ADVANCED_FACE ( 'NONE', ( #7292 ), #12432, .F. ) ;
#20014=DIRECTION ( 'NONE',  ( -0.000000000000000000, -0.000000000000000000, 1.000000000000000000 ) ) ;
#20015=VECTOR ( 'NONE', #21782, 1000.000000000000000 ) ;
#20017=DIRECTION ( 'NONE',  ( 0.000000000000000000, 0.000000000000000000, -1.000000000000000000 ) ) ;
#20018=EDGE_CURVE ( 'NONE', #21174, #15060, #935, .T. ) ;
#20021=CIRCLE ( 'NONE', #3926, 2.099999999999997868 ) ;
#20024=FACE_OUTER_BOUND ( 'NONE', #22507, .T. ) ;
#20026=DIRECTION ( 'NONE',  ( 0.000000000000000000, 1.000000000000000000, 0.000000000000000000 ) ) ;
#20027=CARTESIAN_POINT ( 'NONE',  ( 0.3709469612218444512, -0.009390992346624811235, -50.78654667931662914 ) ) ;
#20033=CARTESIAN_POINT ( 'NONE',  ( -1.387778780781445518E-14, 20.00000000000000355, -102.0000000000000142 ) ) ;
#20038=CARTESIAN_POINT ( 'NONE',  ( -0.3107847162787801265, 39.99819769545531756, -49.10452103004165281 ) ) ;
#20043=DIRECTION ( 'NONE',  ( -0.000000000000000000, -0.000000000000000000, -1.000000000000000000 ) ) ;
#20044=CYLINDRICAL_SURFACE ( 'NONE', #8949, 10.00000000000000178 ) ;
#20047=VECTOR ( 'NONE', #9489, 1000.000000000000114 ) ;
#20050=DIRECTION ( 'NONE',  ( -1.224646799147353207E-16, 1.000000000000000000, 0.000000000000000000 ) ) ;
#20052=DIRECTION ( 'NONE',  ( 0.000000000000000000, 0.000000000000000000, -1.000000000000000000 ) ) ;
#20055=EDGE_CURVE ( 'NONE', #12680, #7125, #5680, .T. ) ;
#20058=CIRCLE ( 'NONE', #16015, 2.099999999999997868 ) ;
#20060=CARTESIAN_POINT ( 'NONE',  ( -4.416367413074144821, 40.00000000000001421, 51.31508042366087352 ) ) ;
#20065=CARTESIAN_POINT ( 'NONE',  ( -42.50000000000000711, -12.00000000000012434, -47.50000000000000000 ) ) ;
#20067=CARTESIAN_POINT ( 'NONE',  ( -0.02632564323144977528, 39.99999593179830981, -48.75445554395042080 ) ) ;
#20069=ADVANCED_FACE ( 'NONE', ( #9124 ), #16099, .F. ) ;
#20071=DIRECTION ( 'NONE',  ( -1.000000000000000000, 0.000000000000000000, 0.000000000000000000 ) ) ;
#20075=CONICAL_SURFACE ( 'NONE', #21170, 2.525000000000110489, 0.7853981633971014453 ) ;
#20078=VERTEX_POINT ( 'NONE', #21383 ) ;
#20079=VERTEX_POINT ( 'NONE', #5801 ) ;
#20082=CARTESIAN_POINT ( 'NONE',  ( 14.64427171882021028, 33.62973864230776400, -59.05294378005808653 ) ) ;
#20084=CARTESIAN_POINT ( 'NONE',  ( -15.50000000000011013, 42.51666049839536043, -105.0010000000000048 ) ) ;
#20087=ORIENTED_EDGE ( 'NONE', *, *, #20522, .F. ) ;
#20088=CARTESIAN_POINT ( 'NONE',  ( 6.696867368503558448E-15, 40.00000000000000000, 38.73397172404480671 ) ) ;
#20090=AXIS2_PLACEMENT_3D ( 'NONE', #17195, #20640, #1509 ) ;
#20091=ORIENTED_EDGE ( 'NONE', *, *, #20750, .F. ) ;
#20092=CARTESIAN_POINT ( 'NONE',  ( -22.29010897948493763, 17.41268129326156355, -58.63841251601397175 ) ) ;
#20093=CARTESIAN_POINT ( 'NONE',  ( 0.7785676492820222672, 40.00000000000002842, 49.23936426806961464 ) ) ;
#20096=DIRECTION ( 'NONE',  ( 0.000000000000000000, 1.000000000000000000, 0.000000000000000000 ) ) ;
#20098=CARTESIAN_POINT ( 'NONE',  ( 1.575018543176820440, 39.98856470501870319, 49.93405373658204383 ) ) ;
#20100=CARTESIAN_POINT ( 'NONE',  ( 7.604730156747764556E-14, -1.031417236136237481, -48.34206739765565430 ) ) ;
#20101=ORIENTED_EDGE ( 'NONE', *, *, #16215, .F. ) ;
#20102=CARTESIAN_POINT ( 'NONE',  ( -35.00000000000000000, 38.99999999999999289, 1.387778780781445676E-14 ) ) ;
#20104=LINE ( 'NONE', #13086, #10772 ) ;
#20105=CYLINDRICAL_SURFACE ( 'NONE', #11444, 18.00000000000000000 ) ;
#20106=CARTESIAN_POINT ( 'NONE',  ( 35.00000000000000000, -9.000000000000001776, 14.00000000000000355 ) ) ;
#20107=CARTESIAN_POINT ( 'NONE',  ( 17.37021972826951455, 10.07190481803176318, -57.39172882205954807 ) ) ;
#20108=ADVANCED_FACE ( 'NONE', ( #10948 ), #16208, .F. ) ;
#20112=ADVANCED_FACE ( 'NONE', ( #5099 ), #18725, .F. ) ;
#20113=ORIENTED_EDGE ( 'NONE', *, *, #6511, .T. ) ;
#20114=CARTESIAN_POINT ( 'NONE',  ( 11.52370268964480005, 39.05614286667413637, 55.22012726439884744 ) ) ;
#20115=CARTESIAN_POINT ( 'NONE',  ( 42.50000000000000711, -12.00000000000000000, 45.00000000000000711 ) ) ;
#20117=ADVANCED_FACE ( 'NONE', ( #19335 ), #22559, .F. ) ;
#20122=AXIS2_PLACEMENT_3D ( 'NONE', #21248, #16731, #14585 ) ;
#20126=CARTESIAN_POINT ( 'NONE',  ( -20.00000000000001421, 20.00000000000000355, 60.62177826491070931 ) ) ;
#20131=CARTESIAN_POINT ( 'NONE',  ( -6.297086633636163278, 38.99689310884462401, 53.73982279751612623 ) ) ;
#20135=CIRCLE ( 'NONE', #1468, 6.499999999999999112 ) ;
#20136=EDGE_CURVE ( 'NONE', #14267, #12579, #9353, .T. ) ;
#20138=CARTESIAN_POINT ( 'NONE',  ( -21.60519577075148590, 26.10363331747822357, 58.48615516158935179 ) ) ;
#20140=EDGE_CURVE ( 'NONE', #19936, #6468, #1312, .T. ) ;
#20144=CIRCLE ( 'NONE', #1855, 2.000000000000000888 ) ;
#20147=DIRECTION ( 'NONE',  ( 0.000000000000000000, 0.000000000000000000, 1.000000000000000000 ) ) ;
#20148=CARTESIAN_POINT ( 'NONE',  ( -5.204760841428789142, 39.83793900407623312, -52.32476308507700224 ) ) ;
#20153=CARTESIAN_POINT ( 'NONE',  ( 19.67606655124947324, 9.154757266467395738, 58.01240525280897486 ) ) ;
#20158=CARTESIAN_POINT ( 'NONE',  ( -35.00000000000000000, 39.00000000000000711, 1.387778780781445676E-14 ) ) ;
#20161=EDGE_CURVE ( 'NONE', #9888, #4759, #9703, .T. ) ;
#20162=CARTESIAN_POINT ( 'NONE',  ( 34.99999999999980815, 40.00000000000000000, 54.99999999999922551 ) ) ;
#20163=CARTESIAN_POINT ( 'NONE',  ( 3.807409362178445278, 39.99999999999999289, -50.99570508274572234 ) ) ;
#20165=CARTESIAN_POINT ( 'NONE',  ( 4.436829441114990225, 39.87775404803028323, -51.86208824299732356 ) ) ;
#20168=CARTESIAN_POINT ( 'NONE',  ( 34.99999999999980815, 26.00000000000000355, 54.99999999999922551 ) ) ;
#20172=CARTESIAN_POINT ( 'NONE',  ( 35.00000000000000711, 40.00000000000000000, 58.99999999999995026 ) ) ;
#20173=ORIENTED_EDGE ( 'NONE', *, *, #18123, .T. ) ;
#20174=CARTESIAN_POINT ( 'NONE',  ( -13.00000000000011546, 42.51666049839536043, -100.0000000000000000 ) ) ;
#20176=CARTESIAN_POINT ( 'NONE',  ( 8.923978417723413159, 2.083761144195372950, -56.51262908347433722 ) ) ;
#20180=CARTESIAN_POINT ( 'NONE',  ( -1.387778780781445518E-14, 20.00000000000000355, -100.0000000000000000 ) ) ;
#20186=ORIENTED_EDGE ( 'NONE', *, *, #22109, .F. ) ;
#20191=CARTESIAN_POINT ( 'NONE',  ( 18.85684496195309023, 26.68267098057082976, 60.33873919100126670 ) ) ;
#20195=FACE_OUTER_BOUND ( 'NONE', #5830, .T. ) ;
#20196=ORIENTED_EDGE ( 'NONE', *, *, #4764, .T. ) ;
#20197=DIRECTION ( 'NONE',  ( 0.000000000000000000, 0.000000000000000000, 1.000000000000000000 ) ) ;
#20199=VERTEX_POINT ( 'NONE', #18046 ) ;
#20201=DIRECTION ( 'NONE',  ( -0.000000000000000000, 1.000000000000000000, -0.000000000000000000 ) ) ;
#20204=DIRECTION ( 'NONE',  ( -0.000000000000000000, -0.000000000000000000, -1.000000000000000000 ) ) ;
#20205=VERTEX_POINT ( 'NONE', #21965 ) ;
#20206=CARTESIAN_POINT ( 'NONE',  ( -42.50000000000000711, -9.600000000000001421, -50.00000000000000000 ) ) ;
#20209=CARTESIAN_POINT ( 'NONE',  ( 90.00000000000000000, 28.00000000000000000, -9.108981535246192915E-16 ) ) ;
#20212=CARTESIAN_POINT ( 'NONE',  ( -9.103081159019540181, 0.03030367950604016467, 53.87333532811888404 ) ) ;
#20213=EDGE_LOOP ( 'NONE', ( #10386, #14535 ) ) ;
#20215=DIRECTION ( 'NONE',  ( 1.000000000000000000, 0.000000000000000000, 0.000000000000000000 ) ) ;
#20216=FACE_OUTER_BOUND ( 'NONE', #5632, .T. ) ;
#20218=CARTESIAN_POINT ( 'NONE',  ( 22.29474960931338856, 17.42887675327984098, -58.63958600108815489 ) ) ;
#20220=CONICAL_SURFACE ( 'NONE', #3392, 15.99999999999993072, 0.7853981633974415066 ) ;
#20222=EDGE_LOOP ( 'NONE', ( #20290, #6567, #17899, #16295 ) ) ;
#20223=ORIENTED_EDGE ( 'NONE', *, *, #7467, .F. ) ;
#20229=CARTESIAN_POINT ( 'NONE',  ( -8.306841138099667177, 0.005341471314548606325, -53.48947974199504074 ) ) ;
#20232=ORIENTED_EDGE ( 'NONE', *, *, #12103, .T. ) ;
#20238=CARTESIAN_POINT ( 'NONE',  ( -16.44544766657918444, 31.39195386311722302, -59.65016313815161197 ) ) ;
#20240=VECTOR ( 'NONE', #15843, 1000.000000000000000 ) ;
#20241=DIRECTION ( 'NONE',  ( -0.000000000000000000, -1.000000000000000000, -0.000000000000000000 ) ) ;
#20243=EDGE_CURVE ( 'NONE', #13151, #2902, #10777, .T. ) ;
#20245=EDGE_LOOP ( 'NONE', ( #9788, #9941 ) ) ;
#20246=ADVANCED_FACE ( 'NONE', ( #2481 ), #20360, .F. ) ;
#20248=CARTESIAN_POINT ( 'NONE',  ( -17.37021972826562077, 10.07190481803563742, 57.39172882205629378 ) ) ;
#20253=CARTESIAN_POINT ( 'NONE',  ( -10.36558328700373011, 39.99999999999999289, 53.76404159467914923 ) ) ;
#20256=CARTESIAN_POINT ( 'NONE',  ( 4.589682443554551128, 39.46972628399738170, 53.62209933471819312 ) ) ;
#20263=ORIENTED_EDGE ( 'NONE', *, *, #7254, .F. ) ;
#20264=CIRCLE ( 'NONE', #4532, 2.499999999999996891 ) ;
#20265=CARTESIAN_POINT ( 'NONE',  ( -10.74988822594902693, 39.17840323696252369, 54.92437902628115864 ) ) ;
#20266=CARTESIAN_POINT ( 'NONE',  ( 11.68090480754629645, 3.765577839755392731, 57.90797000640142045 ) ) ;
#20267=CARTESIAN_POINT ( 'NONE',  ( -90.00000000000000000, 28.00000000000000000, -2.099999999999991651 ) ) ;
#20269=VERTEX_POINT ( 'NONE', #13663 ) ;
#20270=CIRCLE ( 'NONE', #12924, 2.099999999999997868 ) ;
#20271=FACE_OUTER_BOUND ( 'NONE', #18157, .T. ) ;
#20277=FACE_OUTER_BOUND ( 'NONE', #6674, .T. ) ;
#20281=CARTESIAN_POINT ( 'NONE',  ( 0.7619088751511168267, 39.99660921569888217, -49.31788807117369799 ) ) ;
#20286=LINE ( 'NONE', #11345, #654 ) ;
#20290=ORIENTED_EDGE ( 'NONE', *, *, #8578, .T. ) ;
#20292=CARTESIAN_POINT ( 'NONE',  ( 9.103081159015154356, 0.03030367950454006254, 53.87333532811640424 ) ) ;
#20293=CARTESIAN_POINT ( 'NONE',  ( 7.505578006075176667, 1.461761173328237851, -55.63523492904085543 ) ) ;
#20294=DIRECTION ( 'NONE',  ( 0.000000000000000000, -1.000000000000000000, 0.000000000000000000 ) ) ;
#20295=ADVANCED_FACE ( 'NONE', ( #20464 ), #20679, .F. ) ;
#20297=ADVANCED_FACE ( 'NONE', ( #13555, #22306 ), #1662, .T. ) ;
#20299=DIRECTION ( 'NONE',  ( 0.000000000000000000, -1.000000000000000000, 0.000000000000000000 ) ) ;
#20303=AXIS2_PLACEMENT_3D ( 'NONE', #5831, #11083, #18075 ) ;
#20307=CARTESIAN_POINT ( 'NONE',  ( 10.45842016914148509, 40.00000000000000000, 53.79442460303516782 ) ) ;
#20317=PLANE ( 'NONE',  #18893 ) ;
#20319=ADVANCED_FACE ( 'NONE', ( #6478 ), #12642, .F. ) ;
#20321=CARTESIAN_POINT ( 'NONE',  ( 4.406385930812127150, 39.99999999999999289, 51.31001910650969222 ) ) ;
#20322=ORIENTED_EDGE ( 'NONE', *, *, #18123, .F. ) ;
#20324=CARTESIAN_POINT ( 'NONE',  ( 7.928368521050060735, 38.36676511147830126, -56.15748794203490490 ) ) ;
#20325=ORIENTED_EDGE ( 'NONE', *, *, #10402, .F. ) ;
#20326=CARTESIAN_POINT ( 'NONE',  ( -42.50000000000000711, -12.00000000000000000, 49.60000000000000853 ) ) ;
#20328=CARTESIAN_POINT ( 'NONE',  ( 14.19004819996276723, 37.38003124960520296, 56.27686160268850557 ) ) ;
#20329=DIRECTION ( 'NONE',  ( -0.000000000000000000, -0.000000000000000000, -1.000000000000000000 ) ) ;
#20332=CARTESIAN_POINT ( 'NONE',  ( 18.94109686629718681, 13.34133107273948227, -60.36587731981236260 ) ) ;
#20337=ADVANCED_FACE ( 'NONE', ( #3043 ), #5037, .F. ) ;
#20340=DIRECTION ( 'NONE',  ( 0.000000000000000000, 0.000000000000000000, 1.000000000000000000 ) ) ;
#20342=ORIENTED_EDGE ( 'NONE', *, *, #19065, .T. ) ;
#20343=DIRECTION ( 'NONE',  ( -0.000000000000000000, -1.000000000000000000, -0.000000000000000000 ) ) ;
#20344=CARTESIAN_POINT ( 'NONE',  ( -9.367793990838201523, -4.928932186899944057, -51.00106331755883105 ) ) ;
#20349=DIRECTION ( 'NONE',  ( -0.000000000000000000, -1.000000000000000000, -0.000000000000000000 ) ) ;
#20351=CARTESIAN_POINT ( 'NONE',  ( -7.577104390338862849, -0.4826542685308932157, -53.01683071947938686 ) ) ;
#20355=CARTESIAN_POINT ( 'NONE',  ( -19.01465036493458882, 26.21927150370769866, -60.37937655616647703 ) ) ;
#20360=CONICAL_SURFACE ( 'NONE', #10814, 49.99999999999998579, 0.7853981633974657095 ) ;
#20361=EDGE_LOOP ( 'NONE', ( #2672, #14898, #3129, #17681 ) ) ;
#20364=EDGE_LOOP ( 'NONE', ( #9238, #59 ) ) ;
#20365=CARTESIAN_POINT ( 'NONE',  ( -14.89439646620539293, 6.624450698086694622, 59.14252023618892906 ) ) ;
#20368=DIRECTION ( 'NONE',  ( -0.000000000000000000, -1.000000000000000000, -0.000000000000000000 ) ) ;
#20371=ORIENTED_EDGE ( 'NONE', *, *, #14414, .T. ) ;
#20373=CARTESIAN_POINT ( 'NONE',  ( -4.794048179926227782, 40.00000000000000000, -51.50619363643422588 ) ) ;
#20376=FACE_OUTER_BOUND ( 'NONE', #13767, .T. ) ;
#20378=VERTEX_POINT ( 'NONE', #21246 ) ;
#20379=LINE ( 'NONE', #3188, #5146 ) ;
#20380=CYLINDRICAL_SURFACE ( 'NONE', #22527, 2.099999999999997868 ) ;
#20381=VECTOR ( 'NONE', #18018, 1000.000000000000000 ) ;
#20382=VERTEX_POINT ( 'NONE', #268 ) ;
#20389=AXIS2_PLACEMENT_3D ( 'NONE', #9410, #12935, #13162 ) ;
#20390=EDGE_LOOP ( 'NONE', ( #5959, #22288 ) ) ;
#20391=CARTESIAN_POINT ( 'NONE',  ( -9.370858128257053110, -4.928932186902839518, 51.00253624878534708 ) ) ;
#20394=CARTESIAN_POINT ( 'NONE',  ( 14.68506606271058779, 16.91806408329018652, 45.68712064066588141 ) ) ;
#20399=CARTESIAN_POINT ( 'NONE',  ( -13.25963002225075371, 27.02330685613478423, -45.02656532858657812 ) ) ;
#20401=DIRECTION ( 'NONE',  ( 0.000000000000000000, 0.000000000000000000, 1.000000000000000000 ) ) ;
#20402=ORIENTED_EDGE ( 'NONE', *, *, #13168, .T. ) ;
#20403=CARTESIAN_POINT ( 'NONE',  ( 14.69988787053502222, 23.08500126984896639, 45.69379240540679632 ) ) ;
#20405=CARTESIAN_POINT ( 'NONE',  ( 1.485717122675112911, -1.299971956346694490, 49.29290837556793292 ) ) ;
#20406=CARTESIAN_POINT ( 'NONE',  ( 7.505578006075174891, 1.461761173328240071, -55.63523492904086254 ) ) ;
#20407=CARTESIAN_POINT ( 'NONE',  ( -0.1621100730513900801, 39.99984845991361482, -48.85976302750078304 ) ) ;
#20412=CIRCLE ( 'NONE', #19322, 60.00000000000000000 ) ;
#20413=CIRCLE ( 'NONE', #1007, 60.00000000000000000 ) ;
#20415=CIRCLE ( 'NONE', #17478, 2.500000000000002220 ) ;
#20420=ORIENTED_EDGE ( 'NONE', *, *, #19319, .F. ) ;
#20421=CARTESIAN_POINT ( 'NONE',  ( 9.144347024359401388, 37.80953375799288807, 56.77060857467738941 ) ) ;
#20422=CARTESIAN_POINT ( 'NONE',  ( 11.68090480754629112, 3.765577839755377187, -57.90797000640139913 ) ) ;
#20423=CARTESIAN_POINT ( 'NONE',  ( -42.50000000000000711, -12.00000000000012434, -50.02500000000011227 ) ) ;
#20426=CARTESIAN_POINT ( 'NONE',  ( 3.601266574137822474, 5.429865540864382112, -39.39030536259068782 ) ) ;
#20431=CARTESIAN_POINT ( 'NONE',  ( -14.04383866228955746, 14.71638174774082941, -45.39674436955349535 ) ) ;
#20433=PLANE ( 'NONE',  #21049 ) ;
#20434=CARTESIAN_POINT ( 'NONE',  ( 13.76051559511272693, 5.481080969678164827, -58.73291665846257104 ) ) ;
#20435=ORIENTED_EDGE ( 'NONE', *, *, #3104, .F. ) ;
#20436=DIRECTION ( 'NONE',  ( 0.000000000000000000, 0.000000000000000000, 1.000000000000000000 ) ) ;
#20438=ORIENTED_EDGE ( 'NONE', *, *, #2984, .F. ) ;
#20440=CARTESIAN_POINT ( 'NONE',  ( -0.6847309795004193900, -1.267153214277350948, -48.72709510502366470 ) ) ;
#20441=CIRCLE ( 'NONE', #6170, 51.00000000000002132 ) ;
#20448=CARTESIAN_POINT ( 'NONE',  ( 15.91215689494260843, 32.15331685092851188, -56.91770382337011114 ) ) ;
#20449=VERTEX_POINT ( 'NONE', #12307 ) ;
#20451=AXIS2_PLACEMENT_3D ( 'NONE', #16696, #17883, #14959 ) ;
#20455=AXIS2_PLACEMENT_3D ( 'NONE', #21152, #63, #17704 ) ;
#20464=FACE_OUTER_BOUND ( 'NONE', #4830, .T. ) ;
#20465=DIRECTION ( 'NONE',  ( -0.000000000000000000, -1.000000000000000000, -0.000000000000000000 ) ) ;
#20467=CARTESIAN_POINT ( 'NONE',  ( -18.31820558117436448, 28.04217374067966873, -60.19578215372065699 ) ) ;
#20470=CARTESIAN_POINT ( 'NONE',  ( -13.08927703801865405, 12.63446361230554693, 44.94509734929668809 ) ) ;
#20472=ORIENTED_EDGE ( 'NONE', *, *, #17772, .T. ) ;
#20474=ORIENTED_EDGE ( 'NONE', *, *, #8027, .F. ) ;
#20476=CARTESIAN_POINT ( 'NONE',  ( -18.94109686629600731, 13.34133107273681595, 60.36587731981239813 ) ) ;
#20477=DIRECTION ( 'NONE',  ( 0.000000000000000000, -1.000000000000000000, 0.000000000000000000 ) ) ;
#20478=AXIS2_PLACEMENT_3D ( 'NONE', #329, #7320, #14285 ) ;
#20484=CARTESIAN_POINT ( 'NONE',  ( -7.287850675723428040, 40.00000000000000000, -52.67053208787582719 ) ) ;
#20485=CARTESIAN_POINT ( 'NONE',  ( -23.50000000000001066, 19.99999999999982947, 60.00099999999999767 ) ) ;
#20486=CARTESIAN_POINT ( 'NONE',  ( 42.50000000000000711, -9.600000000000001421, -47.50000000000000000 ) ) ;
#20489=ADVANCED_FACE ( 'NONE', ( #10578 ), #1825, .F. ) ;
#20490=ORIENTED_EDGE ( 'NONE', *, *, #3834, .T. ) ;
#20492=VECTOR ( 'NONE', #2487, 1000.000000000000000 ) ;
#20496=EDGE_CURVE ( 'NONE', #18353, #13383, #11378, .T. ) ;
#20498=CARTESIAN_POINT ( 'NONE',  ( -5.095494235770363645, -3.097009620008996045, 50.75850000587684718 ) ) ;
#20500=CARTESIAN_POINT ( 'NONE',  ( 12.99999999999993960, 42.51666049839543149, -105.0010000000000048 ) ) ;
#20502=CARTESIAN_POINT ( 'NONE',  ( 10.63866000424707003, 9.419394561690063838, 43.66469350997158472 ) ) ;
#20505=DIRECTION ( 'NONE',  ( -0.000000000000000000, -1.000000000000000000, -0.000000000000000000 ) ) ;
#20507=CARTESIAN_POINT ( 'NONE',  ( -19.61594976190323081, 16.00511159616170431, -58.04523854797172078 ) ) ;
#20508=CARTESIAN_POINT ( 'NONE',  ( 25.99999999999998579, 19.99999999999999645, 60.00099999999999767 ) ) ;
#20509=CARTESIAN_POINT ( 'NONE',  ( -15.91215689494263330, 32.15331685092852609, 56.91770382337013245 ) ) ;
#20510=VERTEX_POINT ( 'NONE', #9660 ) ;
#20513=CARTESIAN_POINT ( 'NONE',  ( 9.867969867548763929, 0.2954100743914914728, -54.30456930252559289 ) ) ;
#20516=VERTEX_POINT ( 'NONE', #954 ) ;
#20520=LINE ( 'NONE', #20623, #9640 ) ;
#20522=EDGE_CURVE ( 'NONE', #19009, #16203, #3166, .T. ) ;
#20527=ORIENTED_EDGE ( 'NONE', *, *, #7041, .F. ) ;
#20528=DIRECTION ( 'NONE',  ( 0.000000000000000000, 0.000000000000000000, 1.000000000000000000 ) ) ;
#20530=AXIS2_PLACEMENT_3D ( 'NONE', #9223, #16202, #513 ) ;
#20534=DIRECTION ( 'NONE',  ( 0.000000000000000000, 0.000000000000000000, 1.000000000000000000 ) ) ;
#20535=ORIENTED_EDGE ( 'NONE', *, *, #12803, .T. ) ;
#20539=DIRECTION ( 'NONE',  ( 0.000000000000000000, 0.000000000000000000, 1.000000000000000000 ) ) ;
#20541=CARTESIAN_POINT ( 'NONE',  ( 10.50000000000024514, -2.516660498395250301, -105.0010000000000048 ) ) ;
#20548=CARTESIAN_POINT ( 'NONE',  ( -18.35281960068863327, 33.06122318964058593, 57.65236019522518518 ) ) ;
#20550=DIRECTION ( 'NONE',  ( 8.659560562355143632E-17, -0.7071067811865302533, 0.7071067811865647812 ) ) ;
#20554=ADVANCED_FACE ( 'NONE', ( #21592 ), #11718, .T. ) ;
#20555=CARTESIAN_POINT ( 'NONE',  ( 17.57556337526168733, 10.44046169743542052, -57.45538260706032929 ) ) ;
#20561=VECTOR ( 'NONE', #6772, 1000.000000000000114 ) ;
#20562=LINE ( 'NONE', #22298, #19800 ) ;
#20568=CARTESIAN_POINT ( 'NONE',  ( 8.970886036659246443, 37.88902356861865428, -54.67438719140665881 ) ) ;
#20570=DIRECTION ( 'NONE',  ( 0.000000000000000000, -1.000000000000000000, 0.000000000000000000 ) ) ;
#20571=CARTESIAN_POINT ( 'NONE',  ( -0.3359952163700163918, 39.99934595043738028, 48.99376255120481716 ) ) ;
#20572=EDGE_CURVE ( 'NONE', #7317, #3415, #1630, .T. ) ;
#20575=ORIENTED_EDGE ( 'NONE', *, *, #3224, .F. ) ;
#20576=ORIENTED_EDGE ( 'NONE', *, *, #19289, .T. ) ;
#20580=CARTESIAN_POINT ( 'NONE',  ( -22.29474960931412753, 17.42887675328155694, 58.63958600108833252 ) ) ;
#20584=ADVANCED_FACE ( 'NONE', ( #20650 ), #4264, .F. ) ;
#20588=CARTESIAN_POINT ( 'NONE',  ( -8.265432227388908260, 40.00000000000000000, -53.06731920609691855 ) ) ;
#20590=CARTESIAN_POINT ( 'NONE',  ( 11.51194040402256746, 39.05862814753313472, -55.21283662269733838 ) ) ;
#20592=ORIENTED_EDGE ( 'NONE', *, *, #11267, .F. ) ;
#20598=EDGE_LOOP ( 'NONE', ( #1965, #1023, #20490, #4471 ) ) ;
#20601=ORIENTED_EDGE ( 'NONE', *, *, #9671, .T. ) ;
#20602=CARTESIAN_POINT ( 'NONE',  ( 42.50000000000000711, -5.000000000000000000, 45.40000000000001279 ) ) ;
#20604=ORIENTED_EDGE ( 'NONE', *, *, #19008, .T. ) ;
#20609=CARTESIAN_POINT ( 'NONE',  ( -19.93949378746062351, 21.61607484719041850, -60.60748883510625973 ) ) ;
#20610=CARTESIAN_POINT ( 'NONE',  ( -9.852267639826653323, 31.31642578264289156, -43.21671877549178475 ) ) ;
#20613=FACE_OUTER_BOUND ( 'NONE', #9346, .T. ) ;
#20614=ORIENTED_EDGE ( 'NONE', *, *, #21786, .F. ) ;
#20615=CARTESIAN_POINT ( 'NONE',  ( 7.017626609043924546, 33.27455722914837111, 41.44244536674933954 ) ) ;
#20616=LINE ( 'NONE', #15680, #15142 ) ;
#20618=CARTESIAN_POINT ( 'NONE',  ( 9.103081159019511759, 0.03030367950603989405, -53.87333532811885561 ) ) ;
#20623=CARTESIAN_POINT ( 'NONE',  ( 35.00000000000000711, -4.999999999999997335, -57.00000000000001421 ) ) ;
#20625=EDGE_CURVE ( 'NONE', #3760, #22096, #6788, .T. ) ;
#20626=VERTEX_POINT ( 'NONE', #22043 ) ;
#20627=AXIS2_PLACEMENT_3D ( 'NONE', #17955, #772, #9486 ) ;
#20636=DIRECTION ( 'NONE',  ( -1.000000000000000000, 0.000000000000000000, 0.000000000000000000 ) ) ;
#20637=FACE_OUTER_BOUND ( 'NONE', #2749, .T. ) ;
#20638=CARTESIAN_POINT ( 'NONE',  ( -35.00000000000000000, 40.00000000000000000, -49.99999999999997158 ) ) ;
#20640=DIRECTION ( 'NONE',  ( 0.000000000000000000, -1.000000000000000000, 0.000000000000000000 ) ) ;
#20643=LINE ( 'NONE', #15702, #18565 ) ;
#20645=CARTESIAN_POINT ( 'NONE',  ( -35.00000000000000000, -4.928932188134504955, 1.387778780781445676E-14 ) ) ;
#20646=CARTESIAN_POINT ( 'NONE',  ( 7.766910979104990176, 39.99999999999999289, 52.87044925761806269 ) ) ;
#20647=ORIENTED_EDGE ( 'NONE', *, *, #6511, .F. ) ;
#20649=ORIENTED_EDGE ( 'NONE', *, *, #12181, .T. ) ;
#20650=FACE_OUTER_BOUND ( 'NONE', #9455, .T. ) ;
#20651=CIRCLE ( 'NONE', #21387, 6.499999999999999112 ) ;
#20652=CARTESIAN_POINT ( 'NONE',  ( -21.73016838732310774, 25.62687619368171710, 58.51481333197136792 ) ) ;
#20655=AXIS2_PLACEMENT_3D ( 'NONE', #10842, #21742, #6039 ) ;
#20656=LINE ( 'NONE', #4753, #10798 ) ;
#20660=EDGE_CURVE ( 'NONE', #599, #15249, #1176, .T. ) ;
#20663=CONICAL_SURFACE ( 'NONE', #11156, 2.099999999999997868, 1.029744258676652091 ) ;
#20667=EDGE_CURVE ( 'NONE', #15820, #17279, #15966, .T. ) ;
#20671=AXIS2_PLACEMENT_3D ( 'NONE', #4462, #2398, #7894 ) ;
#20672=CARTESIAN_POINT ( 'NONE',  ( 22.41121774633936070, 19.23761757294737151, 58.66449182057562695 ) ) ;
#20673=DIRECTION ( 'NONE',  ( -0.000000000000000000, -1.000000000000000000, -0.000000000000000000 ) ) ;
#20676=DIRECTION ( 'NONE',  ( 0.000000000000000000, 0.000000000000000000, 1.000000000000000000 ) ) ;
#20677=ORIENTED_EDGE ( 'NONE', *, *, #3927, .T. ) ;
#20679=CYLINDRICAL_SURFACE ( 'NONE', #957, 2.099999999999997868 ) ;
#20682=AXIS2_PLACEMENT_3D ( 'NONE', #619, #14919, #20215 ) ;
#20684=CARTESIAN_POINT ( 'NONE',  ( -5.724874953890430440, 39.79387174624774559, 52.64592308926970077 ) ) ;
#20690=ORIENTED_EDGE ( 'NONE', *, *, #4026, .F. ) ;
#20691=( BOUNDED_SURFACE ( )  B_SPLINE_SURFACE ( 3, 2, ( 
 ( #22094, #4450, #14627 ),
 ( #2620, #12900, #9492 ),
 ( #19911, #9829, #6168 ),
 ( #16817, #2844, #6045 ),
 ( #21869, #13235, #21634 ),
 ( #13133, #21986, #7761 ),
 ( #18411, #16580, #14961 ),
 ( #887, #1121, #4217 ),
 ( #8114, #14733, #20148 ),
 ( #11427, #16472, #18068 ),
 ( #2731, #6277, #9710 ),
 ( #11078, #2384, #5930 ),
 ( #15072, #16700, #9377 ),
 ( #7656, #4108, #1003 ) ),
 .UNSPECIFIED., .F., .F., .F. ) 
 B_SPLINE_SURFACE_WITH_KNOTS ( ( 4, 2, 2, 2, 2, 2, 4 ),
 ( 3, 3 ),
 ( 0.004259382447192780127, 0.005809352080732721121, 0.007359321714272661248, 0.008909291347812601375, 0.01045926098135254237, 0.01355920024843242262, 0.01665913951551230288 ),
 ( 0.000000000000000000, 0.8363210495138897471 ),
 .UNSPECIFIED. ) 
 GEOMETRIC_REPRESENTATION_ITEM ( )  RATIONAL_B_SPLINE_SURFACE ( (
 ( 1.000000000000000000, 0.7012738381899416007, 0.9022096307043713237),
 ( 1.000000000000000000, 0.7322964233739771567, 0.9123651190729491489),
 ( 1.000000000000000000, 0.7591992615145440881, 0.9211719756968406170),
 ( 1.000000000000000000, 0.8072864693883526899, 0.9369137031300254215),
 ( 1.000000000000000000, 0.8284610246205110773, 0.9438453610848451802),
 ( 1.000000000000000000, 0.8663819189607202542, 0.9562590654590453765),
 ( 1.000000000000000000, 0.8831517595277805777, 0.9617488052667169107),
 ( 1.000000000000000000, 0.9127683925939877874, 0.9714440441011351624),
 ( 1.000000000000000000, 0.9255808901573298053, 0.9756383164096822380),
 ( 1.000000000000000000, 0.9589862157102829743, 0.9865738136639907729),
 ( 1.000000000000000000, 0.9746015990832553877, 0.9916856327878436073),
 ( 1.000000000000000000, 0.9951270141023534910, 0.9984047895650791649),
 ( 1.000000000000000000, 0.9999818006517211533, 0.9999940422995483580),
 ( 1.000000000000000000, 1.000000000000000000, 1.000000000000000000) ) ) 
 REPRESENTATION_ITEM ( '' )  SURFACE ( )  );
#20696=CARTESIAN_POINT ( 'NONE',  ( -12.11890052765076220, 39.66666666666666430, 54.74394698394426229 ) ) ;
#20700=CARTESIAN_POINT ( 'NONE',  ( -11.73108507413472346, 40.00000000000000000, 54.23086838360213591 ) ) ;
#20705=DIRECTION ( 'NONE',  ( -0.000000000000000000, 1.000000000000000000, -0.000000000000000000 ) ) ;
#20707=PLANE ( 'NONE',  #4612 ) ;
#20711=EDGE_CURVE ( 'NONE', #22326, #15589, #21087, .T. ) ;
#20719=PLANE ( 'NONE',  #17044 ) ;
#20724=CARTESIAN_POINT ( 'NONE',  ( -3.192088256997320350, -4.645848710072370658, 47.73628783182301305 ) ) ;
#20725=EDGE_CURVE ( 'NONE', #4439, #454, #971, .T. ) ;
#20726=CARTESIAN_POINT ( 'NONE',  ( 35.00000000000000000, -9.000000000000001776, -9.000000000000000000 ) ) ;
#20727=CIRCLE ( 'NONE', #10416, 60.00000000000000000 ) ;
#20728=TOROIDAL_SURFACE ( 'NONE', #13011, 50.00000000000000000, 10.00000000000000000 ) ;
#20731=AXIS2_PLACEMENT_3D ( 'NONE', #3620, #19197, #152 ) ;
#20732=CARTESIAN_POINT ( 'NONE',  ( 9.579024991656979182, 8.451577327321064814, 43.05667825653220149 ) ) ;
#20733=CARTESIAN_POINT ( 'NONE',  ( -2.090752864397128707, 34.85582703520299930, -38.95144853163190390 ) ) ;
#20734=DIRECTION ( 'NONE',  ( 0.000000000000000000, 0.000000000000000000, 1.000000000000000000 ) ) ;
#20735=CARTESIAN_POINT ( 'NONE',  ( -18.87679372942798395, 13.33229001579394968, -60.34430474298741842 ) ) ;
#20736=CARTESIAN_POINT ( 'NONE',  ( -6.629162819447105726, 39.71713125805204214, 53.15137286438373820 ) ) ;
#20738=ORIENTED_EDGE ( 'NONE', *, *, #16714, .F. ) ;
#20739=CARTESIAN_POINT ( 'NONE',  ( 14.98515767422208178, 20.77155976913489610, 45.81928800960653803 ) ) ;
#20744=DIRECTION ( 'NONE',  ( 0.000000000000000000, 0.000000000000000000, -1.000000000000000000 ) ) ;
#20747=CIRCLE ( 'NONE', #21852, 57.00000000000002132 ) ;
#20750=EDGE_CURVE ( 'NONE', #5360, #13935, #13755, .T. ) ;
#20752=EDGE_LOOP ( 'NONE', ( #8499, #20342, #10078, #10211 ) ) ;
#20753=FACE_OUTER_BOUND ( 'NONE', #6463, .T. ) ;
#20754=FACE_OUTER_BOUND ( 'NONE', #2567, .T. ) ;
#20755=CARTESIAN_POINT ( 'NONE',  ( 35.00000000000000000, 38.99999999999999289, 4.258610482196280173E-15 ) ) ;
#20760=CARTESIAN_POINT ( 'NONE',  ( -34.99999999999980815, 28.00000000000000000, 54.99999999999922551 ) ) ;
#20762=DIRECTION ( 'NONE',  ( 0.000000000000000000, 0.000000000000000000, 1.000000000000000000 ) ) ;
#20766=CARTESIAN_POINT ( 'NONE',  ( 9.066530173131811310, 39.99999999999999289, 53.36211915552348728 ) ) ;
#20769=ORIENTED_EDGE ( 'NONE', *, *, #10691, .F. ) ;
#20771=CARTESIAN_POINT ( 'NONE',  ( -22.43696576003033982, 20.17999529786816737, 58.67002796852977298 ) ) ;
#20777=DIRECTION ( 'NONE',  ( 1.049727191138617217E-16, 0.5150380749100562650, -0.8571673007021111124 ) ) ;
#20778=ADVANCED_FACE ( 'NONE', ( #17889 ), #19998, .T. ) ;
#20779=DIRECTION ( 'NONE',  ( -1.000000000000000000, 0.000000000000000000, 0.000000000000000000 ) ) ;
#20780=VECTOR ( 'NONE', #16118, 1000.000000000000000 ) ;
#20781=AXIS2_PLACEMENT_3D ( 'NONE', #18062, #20026, #21517 ) ;
#20783=EDGE_CURVE ( 'NONE', #9047, #9571, #13971, .T. ) ;
#20787=ORIENTED_EDGE ( 'NONE', *, *, #15942, .F. ) ;
#20790=DIRECTION ( 'NONE',  ( 0.000000000000000000, 1.000000000000000000, 0.000000000000000000 ) ) ;
#20793=PLANE ( 'NONE',  #1864 ) ;
#20795=CIRCLE ( 'NONE', #17854, 18.00000000000000000 ) ;
#20797=EDGE_CURVE ( 'NONE', #9047, #22397, #5724, .T. ) ;
#20798=CARTESIAN_POINT ( 'NONE',  ( 5.833333333333338366, 33.81926995981415729, 40.61164310337067462 ) ) ;
#20799=ORIENTED_EDGE ( 'NONE', *, *, #9040, .T. ) ;
#20800=CARTESIAN_POINT ( 'NONE',  ( 6.803227178530688590, 38.81166136533672528, -55.43135129401763805 ) ) ;
#20805=CARTESIAN_POINT ( 'NONE',  ( -0.5387139470867652324, 39.99828243297760366, 49.14868387071282996 ) ) ;
#20806=CARTESIAN_POINT ( 'NONE',  ( 18.13678767552818272, 6.731837175187128430, 57.58481432322350457 ) ) ;
#20807=CYLINDRICAL_SURFACE ( 'NONE', #4505, 2.499999999999995115 ) ;
#20817=AXIS2_PLACEMENT_3D ( 'NONE', #1847, #9280, #8827 ) ;
#20819=DIRECTION ( 'NONE',  ( -0.000000000000000000, 1.000000000000000000, -0.000000000000000000 ) ) ;
#20821=EDGE_CURVE ( 'NONE', #6579, #6323, #21464, .T. ) ;
#20823=CARTESIAN_POINT ( 'NONE',  ( 6.069328058468995479, 39.76463894486199990, 52.83839005242463571 ) ) ;
#20828=CARTESIAN_POINT ( 'NONE',  ( -35.00000000000000000, 2.142135623730931471, 1.387778780781445676E-14 ) ) ;
#20831=CARTESIAN_POINT ( 'NONE',  ( 10.06223851446537410, 39.28158160658947651, -54.67678195792276341 ) ) ;
#20833=ORIENTED_EDGE ( 'NONE', *, *, #10630, .F. ) ;
#20835=CARTESIAN_POINT ( 'NONE',  ( -20.00000000000001421, 20.00000000000000355, 60.62177826491070931 ) ) ;
#20837=ORIENTED_EDGE ( 'NONE', *, *, #7245, .F. ) ;
#20839=CARTESIAN_POINT ( 'NONE',  ( -8.970889523128901644, 37.88902197091756818, 54.67437798809974225 ) ) ;
#20843=ORIENTED_EDGE ( 'NONE', *, *, #19319, .T. ) ;
#20849=EDGE_CURVE ( 'NONE', #1702, #10048, #681, .T. ) ;
#20855=CARTESIAN_POINT ( 'NONE',  ( -19.27384183542242369, 25.35969264784100474, -57.95172789105616573 ) ) ;
#20857=ORIENTED_EDGE ( 'NONE', *, *, #14778, .F. ) ;
#20860=FACE_OUTER_BOUND ( 'NONE', #17814, .T. ) ;
#20866=VERTEX_POINT ( 'NONE', #8613 ) ;
#20875=EDGE_LOOP ( 'NONE', ( #17194, #1329 ) ) ;
#20876=FACE_OUTER_BOUND ( 'NONE', #6245, .T. ) ;
#20877=DIRECTION ( 'NONE',  ( -1.000000000000000000, 0.000000000000000000, 0.000000000000000000 ) ) ;
#20879=CARTESIAN_POINT ( 'NONE',  ( 4.084299015953619438, -4.682619376883208950, -48.27507093818998385 ) ) ;
#20880=B_SPLINE_CURVE_WITH_KNOTS ( 'NONE', 3,
 ( #21791, #7577, #21566, #6087, #5867, #2428, #9632, #13051, #4377, #12721, #12830, #711, #11355, #7693, #1045, #16622, #14882, #14670, #929, #21908, #6204, #13166 ),
 .UNSPECIFIED., .F., .F.,
 ( 4, 2, 2, 2, 2, 2, 2, 2, 2, 2, 4 ),
 ( 0.007712149587921343294, 0.01231940472852627484, 0.01347121851367750339, 0.01462303229882873194, 0.01692665986913119425, 0.01807847365428242800, 0.01923028743943366176, 0.02153391500973612233, 0.02268572879488734914, 0.02383754258003857596, 0.02614117015034102959 ),
 .UNSPECIFIED. ) ;
#20881=EDGE_CURVE ( 'NONE', #11692, #8817, #7190, .T. ) ;
#20882=CARTESIAN_POINT ( 'NONE',  ( 20.89512770937650643, 28.22558907592241084, -58.31975796628788089 ) ) ;
#20886=CARTESIAN_POINT ( 'NONE',  ( 5.651049729919324527, 39.99999999999999289, 51.93203805547999963 ) ) ;
#20887=CARTESIAN_POINT ( 'NONE',  ( -7.902600844548947734, 39.58333017843621349, -53.79900150422385252 ) ) ;
#20888=ORIENTED_EDGE ( 'NONE', *, *, #7442, .T. ) ;
#20889=CARTESIAN_POINT ( 'NONE',  ( -42.50000000000000711, -12.00000000000000000, 54.00000000000000711 ) ) ;
#20893=EDGE_CURVE ( 'NONE', #12579, #1894, #11210, .T. ) ;
#20895=CARTESIAN_POINT ( 'NONE',  ( -42.50000000000000711, -5.000000000000000000, -47.50000000000000000 ) ) ;
#20896=FACE_OUTER_BOUND ( 'NONE', #1177, .T. ) ;
#20901=ORIENTED_EDGE ( 'NONE', *, *, #17504, .T. ) ;
#20903=CARTESIAN_POINT ( 'NONE',  ( 22.16820537380700173, 16.50892643625843448, 58.61209530626889830 ) ) ;
#20905=CARTESIAN_POINT ( 'NONE',  ( 4.794048089945632363, 40.00000000000000000, 51.50619359082698878 ) ) ;
#20910=EDGE_CURVE ( 'NONE', #6172, #862, #17444, .T. ) ;
#20911=CARTESIAN_POINT ( 'NONE',  ( -2.516035484449607118, 0.1456407669953184991, 52.33281532376254575 ) ) ;
#20915=EDGE_LOOP ( 'NONE', ( #12316, #21714, #22286 ) ) ;
#20916=CARTESIAN_POINT ( 'NONE',  ( 7.704853968945537979, 39.66343356457746694, -53.66055573870352191 ) ) ;
#20917=CARTESIAN_POINT ( 'NONE',  ( -7.928368521050097151, 38.36676511147829416, 56.15748794203494754 ) ) ;
#20918=CARTESIAN_POINT ( 'NONE',  ( -0.5472028025208371949, 39.99822772478366062, 49.15514354140995579 ) ) ;
#20919=EDGE_CURVE ( 'NONE', #22397, #9047, #19655, .T. ) ;
#20924=AXIS2_PLACEMENT_3D ( 'NONE', #7130, #15824, #21120 ) ;
#20925=EDGE_LOOP ( 'NONE', ( #15693, #16568, #19961 ) ) ;
#20928=ORIENTED_EDGE ( 'NONE', *, *, #17140, .F. ) ;
#20929=FACE_OUTER_BOUND ( 'NONE', #13095, .T. ) ;
#20930=CARTESIAN_POINT ( 'NONE',  ( 42.50000000000000711, -5.000000000000000000, 45.40000000000001279 ) ) ;
#20931=CARTESIAN_POINT ( 'NONE',  ( -11.87329829275383375, 39.99999999999997868, -54.28004929202754170 ) ) ;
#20933=CARTESIAN_POINT ( 'NONE',  ( 0.1155398381881750092, 39.99992209574985225, 48.82370845058371600 ) ) ;
#20938=FACE_OUTER_BOUND ( 'NONE', #2346, .T. ) ;
#20939=DIRECTION ( 'NONE',  ( -1.000000000000000000, 0.000000000000000000, 0.000000000000000000 ) ) ;
#20941=CARTESIAN_POINT ( 'NONE',  ( -23.50000000000001066, 19.99999999999982947, -105.0010000000000048 ) ) ;
#20942=ORIENTED_EDGE ( 'NONE', *, *, #17725, .T. ) ;
#20944=CARTESIAN_POINT ( 'NONE',  ( 42.50000000000000711, -12.00000000000000000, -47.50000000000000000 ) ) ;
#20950=ADVANCED_FACE ( 'NONE', ( #21438 ), #18550, .F. ) ;
#20953=DIRECTION ( 'NONE',  ( -0.000000000000000000, -1.000000000000000000, -0.000000000000000000 ) ) ;
#20954=EDGE_CURVE ( 'NONE', #1383, #3928, #7574, .T. ) ;
#20955=ADVANCED_FACE ( 'NONE', ( #2422 ), #10846, .T. ) ;
#20957=B_SPLINE_CURVE_WITH_KNOTS ( 'NONE', 3,
 ( #19582, #554, #21531, #19472, #7547, #17861, #2167, #12245, #12358, #7093, #3892, #10625, #15786, #8920, #19253, #21077, #21189, #5381, #12459, #10859, #19370, #17630 ),
 .UNSPECIFIED., .F., .F.,
 ( 4, 2, 2, 2, 2, 2, 2, 2, 2, 2, 4 ),
 ( 0.007712149587921488143, 0.01231940472852635984, 0.01347121851367757625, 0.01462303229882878919, 0.01692665986913123241, 0.01807847365428245229, 0.01923028743943366869, 0.02153391500973611192, 0.02268572879488733526, 0.02383754258003855514, 0.02614117015034099489 ),
 .UNSPECIFIED. ) ;
#20961=CARTESIAN_POINT ( 'NONE',  ( -18.88991738967393275, 26.58741517404049048, -57.84428223557713267 ) ) ;
#20962=EDGE_CURVE ( 'NONE', #11090, #13123, #14550, .T. ) ;
#20967=ADVANCED_FACE ( 'NONE', ( #16149 ), #5860, .T. ) ;
#20972=CONICAL_SURFACE ( 'NONE', #9610, 2.099999999999997868, 1.029744258676652091 ) ;
#20973=ORIENTED_EDGE ( 'NONE', *, *, #13080, .F. ) ;
#20976=CARTESIAN_POINT ( 'NONE',  ( -42.50000000000000711, -11.97499999999999964, 47.50000000000000711 ) ) ;
#20982=LINE ( 'NONE', #10086, #16048 ) ;
#20984=CARTESIAN_POINT ( 'NONE',  ( -11.09836907989745569, 40.00000000000000000, -54.00358115607139808 ) ) ;
#20986=CARTESIAN_POINT ( 'NONE',  ( 6.699391982050356020, -4.821764332415713561, -49.69317737456918849 ) ) ;
#20987=AXIS2_PLACEMENT_3D ( 'NONE', #2921, #2802, #9896 ) ;
#20989=CARTESIAN_POINT ( 'NONE',  ( 15.67632863000011056, 36.06985656533340290, -56.80410608597895816 ) ) ;
#20990=DIRECTION ( 'NONE',  ( 0.7071067811865463515, 0.000000000000000000, 0.7071067811865487940 ) ) ;
#20993=CARTESIAN_POINT ( 'NONE',  ( 9.855264211176361755, 31.32970427768389499, -43.22210574525156801 ) ) ;
#20994=EDGE_LOOP ( 'NONE', ( #21243, #4642, #7186, #16990, #10454 ) ) ;
#20995=CARTESIAN_POINT ( 'NONE',  ( -35.00000000000000000, -4.999999999999997335, 1.387778780781445676E-14 ) ) ;
#20996=CARTESIAN_POINT ( 'NONE',  ( -19.90072640592962117, 9.610007367499633801, 58.06946678856481725 ) ) ;
#20998=AXIS2_PLACEMENT_3D ( 'NONE', #21611, #3975, #21844 ) ;
#21004=AXIS2_PLACEMENT_3D ( 'NONE', #2541, #9524, #15445 ) ;
#21005=CIRCLE ( 'NONE', #8549, 2.499999999999995115 ) ;
#21006=ORIENTED_EDGE ( 'NONE', *, *, #17290, .F. ) ;
#21009=SHAPE_REPRESENTATION_RELATIONSHIP ( 'NONE' , 'NONE' ,  #21292, #7741 ) ;
#21010=VERTEX_POINT ( 'NONE', #17994 ) ;
#21012=CARTESIAN_POINT ( 'NONE',  ( 13.32368996328068356, 38.03919112700259575, 55.94897837928601803 ) ) ;
#21017=CARTESIAN_POINT ( 'NONE',  ( -35.00000000000000000, -9.000000000000001776, 1.387778780781445676E-14 ) ) ;
#21018=CARTESIAN_POINT ( 'NONE',  ( 0.6864184775310656628, -1.216838870810526219, -47.75834167803935060 ) ) ;
#21021=AXIS2_PLACEMENT_3D ( 'NONE', #2524, #6062, #7900 ) ;
#21024=VERTEX_POINT ( 'NONE', #19840 ) ;
#21028=AXIS2_PLACEMENT_3D ( 'NONE', #6876, #19131, #17281 ) ;
#21029=CARTESIAN_POINT ( 'NONE',  ( 18.82278182890044604, 26.77493817624154460, 60.32982055024199752 ) ) ;
#21030=DIRECTION ( 'NONE',  ( 1.000000000000000000, 0.000000000000000000, 0.000000000000000000 ) ) ;
#21031=DIRECTION ( 'NONE',  ( -0.000000000000000000, 1.000000000000000000, -0.000000000000000000 ) ) ;
#21032=EDGE_CURVE ( 'NONE', #7317, #20449, #12136, .T. ) ;
#21033=EDGE_LOOP ( 'NONE', ( #3021, #1694 ) ) ;
#21042=CARTESIAN_POINT ( 'NONE',  ( 2.213007027836657148, 39.97050984159520226, 50.37695261049397288 ) ) ;
#21044=DIRECTION ( 'NONE',  ( 0.000000000000000000, 0.000000000000000000, 1.000000000000000000 ) ) ;
#21046=CARTESIAN_POINT ( 'NONE',  ( 28.49999999999998224, 19.99999999999999645, -100.0000000000000000 ) ) ;
#21049=AXIS2_PLACEMENT_3D ( 'NONE', #3242, #11712, #6447 ) ;
#21052=PLANE ( 'NONE',  #1021 ) ;
#21053=CARTESIAN_POINT ( 'NONE',  ( -7.704858207814790916, 39.66343987625801759, 53.66055254569381106 ) ) ;
#21056=VECTOR ( 'NONE', #18610, 1000.000000000000000 ) ;
#21059=VECTOR ( 'NONE', #22581, 1000.000000000000000 ) ;
#21063=CARTESIAN_POINT ( 'NONE',  ( -1.387778780781445676E-14, 20.00000000000000000, -101.0000000000000284 ) ) ;
#21065=CARTESIAN_POINT ( 'NONE',  ( -90.00000000000000000, 28.00000000000000000, -9.108981535246192915E-16 ) ) ;
#21066=CARTESIAN_POINT ( 'NONE',  ( -18.48876241336181536, 12.20729522219679986, 60.24712676880315598 ) ) ;
#21068=CARTESIAN_POINT ( 'NONE',  ( -11.24237306623856014, 36.54654314592846021, -57.72256821685509465 ) ) ;
#21071=VECTOR ( 'NONE', #19890, 1000.000000000000000 ) ;
#21075=CIRCLE ( 'NONE', #15198, 60.00000000000000000 ) ;
#21077=CARTESIAN_POINT ( 'NONE',  ( 14.40375226887234561, 15.79546342576959184, -45.56106839101555295 ) ) ;
#21079=VERTEX_POINT ( 'NONE', #3214 ) ;
#21082=EDGE_CURVE ( 'NONE', #18681, #16159, #20747, .T. ) ;
#21087=CIRCLE ( 'NONE', #7554, 10.00000000000000178 ) ;
#21088=AXIS2_PLACEMENT_3D ( 'NONE', #12458, #2048, #10400 ) ;
#21091=DIRECTION ( 'NONE',  ( -0.000000000000000000, 1.000000000000000000, -0.000000000000000000 ) ) ;
#21094=CARTESIAN_POINT ( 'NONE',  ( -34.99999999999980815, 40.00000000000000711, 54.99999999999922551 ) ) ;
#21095=CARTESIAN_POINT ( 'NONE',  ( -1.387778780781445518E-14, 20.00000000000000355, 103.0000000000000284 ) ) ;
#21096=ORIENTED_EDGE ( 'NONE', *, *, #17859, .T. ) ;
#21101=CARTESIAN_POINT ( 'NONE',  ( -7.882609639814679786E-15, -9.552912840896525389E-26, -50.50395615645409464 ) ) ;
#21103=CARTESIAN_POINT ( 'NONE',  ( -1.387778780781445676E-14, 20.00000000000000000, 60.00200000000000244 ) ) ;
#21106=CARTESIAN_POINT ( 'NONE',  ( -2.665760015255949078, 39.95807811140273458, -50.69599157361079023 ) ) ;
#21108=EDGE_LOOP ( 'NONE', ( #3574, #12455, #21096, #9719 ) ) ;
#21110=LINE ( 'NONE', #2197, #19509 ) ;
#21111=AXIS2_PLACEMENT_3D ( 'NONE', #15995, #19455, #7182 ) ;
#21114=ADVANCED_FACE ( 'NONE', ( #8365 ), #6417, .F. ) ;
#21115=VERTEX_POINT ( 'NONE', #15679 ) ;
#21116=CIRCLE ( 'NONE', #996, 20.00000000000000000 ) ;
#21119=VERTEX_POINT ( 'NONE', #3773 ) ;
#21120=DIRECTION ( 'NONE',  ( 0.000000000000000000, 0.000000000000000000, -1.000000000000000000 ) ) ;
#21121=CARTESIAN_POINT ( 'NONE',  ( 21.99996130922171389, 24.71724789032312586, 58.57718774367118186 ) ) ;
#21123=CARTESIAN_POINT ( 'NONE',  ( 4.465627656007536750, 40.00000000000000000, 51.33835359896442441 ) ) ;
#21126=DIRECTION ( 'NONE',  ( -1.000000000000000000, 0.000000000000000000, -0.000000000000000000 ) ) ;
#21130=DIRECTION ( 'NONE',  ( 0.000000000000000000, 0.000000000000000000, -1.000000000000000000 ) ) ;
#21132=CARTESIAN_POINT ( 'NONE',  ( 9.103081159015337320, 0.03030367950460435486, 53.87333532811651793 ) ) ;
#21134=CARTESIAN_POINT ( 'NONE',  ( 1.575029502094859701, 39.98856664293944618, -49.93404254833944123 ) ) ;
#21135=FACE_OUTER_BOUND ( 'NONE', #16583, .T. ) ;
#21136=CARTESIAN_POINT ( 'NONE',  ( -4.517334468824944160, 39.87309017818895995, 51.91252173886011434 ) ) ;
#21137=CIRCLE ( 'NONE', #15637, 2.499999999999998668 ) ;
#21140=CARTESIAN_POINT ( 'NONE',  ( 19.81381843823947264, 22.85613052104596932, 58.09821304537223341 ) ) ;
#21143=DIRECTION ( 'NONE',  ( -1.000000000000000000, 0.000000000000000000, 0.000000000000000000 ) ) ;
#21144=ORIENTED_EDGE ( 'NONE', *, *, #12206, .F. ) ;
#21145=CIRCLE ( 'NONE', #1771, 58.99999999999994316 ) ;
#21151=AXIS2_PLACEMENT_3D ( 'NONE', #7519, #14939, #5802 ) ;
#21152=CARTESIAN_POINT ( 'NONE',  ( 42.50000000000000711, -5.000000000000000000, 47.50000000000000711 ) ) ;
#21153=DIRECTION ( 'NONE',  ( -0.000000000000000000, 1.000000000000000000, -0.000000000000000000 ) ) ;
#21154=CARTESIAN_POINT ( 'NONE',  ( 1.103251425233469529, 39.99275656736713813, 49.57314630728770766 ) ) ;
#21155=AXIS2_PLACEMENT_3D ( 'NONE', #3404, #15980, #11133 ) ;
#21158=DIRECTION ( 'NONE',  ( 0.000000000000000000, 0.000000000000000000, -1.000000000000000000 ) ) ;
#21161=B_SPLINE_CURVE_WITH_KNOTS ( 'NONE', 3,
 ( #1988, #44, #10458, #15953, #21347, #13991, #14339, #262 ),
 .UNSPECIFIED., .F., .F.,
 ( 4, 2, 2, 4 ),
 ( 0.001329099847188741938, 0.002445656686148434990, 0.003562213525108127825, 0.005795327203027498750 ),
 .UNSPECIFIED. ) ;
#21162=( NAMED_UNIT ( * ) PLANE_ANGLE_UNIT ( ) SI_UNIT ( $, .RADIAN. ) );
#21170=AXIS2_PLACEMENT_3D ( 'NONE', #3279, #16796, #1202 ) ;
#21171=FACE_OUTER_BOUND ( 'NONE', #13741, .T. ) ;
#21172=CIRCLE ( 'NONE', #3634, 2.499999999999996891 ) ;
#21173=ORIENTED_EDGE ( 'NONE', *, *, #15085, .F. ) ;
#21174=VERTEX_POINT ( 'NONE', #15783 ) ;
#21175=EDGE_LOOP ( 'NONE', ( #9758, #14082, #14823 ) ) ;
#21176=CARTESIAN_POINT ( 'NONE',  ( 5.961618526219221614, -3.061744126945400879, -51.29856354178556188 ) ) ;
#21182=EDGE_CURVE ( 'NONE', #2480, #7279, #14123, .T. ) ;
#21184=CARTESIAN_POINT ( 'NONE',  ( -14.94062893683336668, 21.54390686295444368, -45.79998742252194432 ) ) ;
#21185=ORIENTED_EDGE ( 'NONE', *, *, #590, .T. ) ;
#21186=CARTESIAN_POINT ( 'NONE',  ( -26.00000000000001421, 19.99999999999982947, 105.0000000000000142 ) ) ;
#21187=CARTESIAN_POINT ( 'NONE',  ( -8.331955809010631597, 38.18181818181817988, -56.36098470834072316 ) ) ;
#21188=CARTESIAN_POINT ( 'NONE',  ( -28.50000000000001421, 19.99999999999982947, -105.0010000000000048 ) ) ;
#21189=CARTESIAN_POINT ( 'NONE',  ( 14.50678847729822252, 16.16560534949679351, -45.60743157421818950 ) ) ;
#21191=VERTEX_POINT ( 'NONE', #13943 ) ;
#21193=FACE_OUTER_BOUND ( 'NONE', #7399, .T. ) ;
#21198=VERTEX_POINT ( 'NONE', #10515 ) ;
#21202=AXIS2_PLACEMENT_3D ( 'NONE', #21529, #9498, #18309 ) ;
#21204=ORIENTED_EDGE ( 'NONE', *, *, #20725, .T. ) ;
#21206=CARTESIAN_POINT ( 'NONE',  ( -8.732260780949433254, 39.99999999999998579, 53.24192688670174789 ) ) ;
#21210=EDGE_CURVE ( 'NONE', #18495, #10435, #6482, .T. ) ;
#21212=DIRECTION ( 'NONE',  ( 1.000000000000000000, 0.000000000000000000, 0.000000000000000000 ) ) ;
#21213=ORIENTED_EDGE ( 'NONE', *, *, #2118, .F. ) ;
#21214=DIRECTION ( 'NONE',  ( 0.000000000000000000, 0.000000000000000000, 1.000000000000000000 ) ) ;
#21215=CARTESIAN_POINT ( 'NONE',  ( -9.744263423232602861, 2.495070046656082674, 54.63687069583399136 ) ) ;
#21216=CARTESIAN_POINT ( 'NONE',  ( -1.092488160344625037, 39.99289796980131229, -49.56515122593324918 ) ) ;
#21217=ORIENTED_EDGE ( 'NONE', *, *, #12011, .T. ) ;
#21219=AXIS2_PLACEMENT_3D ( 'NONE', #20755, #5068, #13616 ) ;
#21221=EDGE_CURVE ( 'NONE', #16362, #21600, #11230, .T. ) ;
#21222=CARTESIAN_POINT ( 'NONE',  ( -6.696867368503558448E-15, 40.00000000000000000, -48.73397172404479960 ) ) ;
#21224=ADVANCED_FACE ( 'NONE', ( #19469 ), #19022, .F. ) ;
#21229=ORIENTED_EDGE ( 'NONE', *, *, #14262, .F. ) ;
#21231=DIRECTION ( 'NONE',  ( -1.000000000000000000, 0.000000000000000000, 0.000000000000000000 ) ) ;
#21233=CARTESIAN_POINT ( 'NONE',  ( 8.553367002852411360, 39.50246935780211999, -54.09836737755986746 ) ) ;
#21243=ORIENTED_EDGE ( 'NONE', *, *, #1633, .F. ) ;
#21245=VERTEX_POINT ( 'NONE', #3670 ) ;
#21246=CARTESIAN_POINT ( 'NONE',  ( 7.776554266669417956E-15, -4.648749848372173865, -45.43309249825056639 ) ) ;
#21248=CARTESIAN_POINT ( 'NONE',  ( 12.99999999999993960, 42.51666049839543149, -100.0000000000000000 ) ) ;
#21252=CARTESIAN_POINT ( 'NONE',  ( 22.42386962120395566, 19.82082524447363525, 58.66720683610022746 ) ) ;
#21255=VECTOR ( 'NONE', #16864, 1000.000000000000000 ) ;
#21256=LINE ( 'NONE', #5334, #868 ) ;
#21259=VERTEX_POINT ( 'NONE', #10856 ) ;
#21266=CARTESIAN_POINT ( 'NONE',  ( 2.098977200742791815, 39.97352556959325653, 50.29629763963205846 ) ) ;
#21267=AXIS2_PLACEMENT_3D ( 'NONE', #5103, #13547, #17109 ) ;
#21269=CARTESIAN_POINT ( 'NONE',  ( 9.103081159019511759, 0.03030367950604059835, -53.87333532811884851 ) ) ;
#21272=DIRECTION ( 'NONE',  ( 0.000000000000000000, 0.000000000000000000, -1.000000000000000000 ) ) ;
#21274=CYLINDRICAL_SURFACE ( 'NONE', #11311, 9.000000000000003553 ) ;
#21275=EDGE_CURVE ( 'NONE', #19009, #16507, #12681, .T. ) ;
#21277=AXIS2_PLACEMENT_3D ( 'NONE', #10414, #15233, #20528 ) ;
#21279=FACE_OUTER_BOUND ( 'NONE', #695, .T. ) ;
#21280=EDGE_CURVE ( 'NONE', #10118, #9571, #11976, .T. ) ;
#21284=EDGE_CURVE ( 'NONE', #3548, #8759, #17829, .T. ) ;
#21286=CARTESIAN_POINT ( 'NONE',  ( -0.1963897509086758586, -3.154216256251429318, -47.17168727994676658 ) ) ;
#21287=DIRECTION ( 'NONE',  ( -0.000000000000000000, -0.000000000000000000, 1.000000000000000000 ) ) ;
#21292=SHAPE_REPRESENTATION ( 'CASE', ( #18273 ), #10192 ) ;
#21294=CARTESIAN_POINT ( 'NONE',  ( -14.58570206007863135, 6.310259562106216080, 59.03202081059066586 ) ) ;
#21299=CARTESIAN_POINT ( 'NONE',  ( -7.928388824789384337, 38.36675580713608014, -56.15749817958554502 ) ) ;
#21301=DIRECTION ( 'NONE',  ( 0.000000000000000000, 0.000000000000000000, -1.000000000000000000 ) ) ;
#21303=CARTESIAN_POINT ( 'NONE',  ( -35.00000000000000000, 0.000000000000000000, -49.99999999999997158 ) ) ;
#21304=FACE_BOUND ( 'NONE', #15114, .T. ) ;
#21310=ORIENTED_EDGE ( 'NONE', *, *, #6010, .F. ) ;
#21315=CARTESIAN_POINT ( 'NONE',  ( -12.27586057105639838, 4.193657236093905283, -55.54740530680978594 ) ) ;
#21319=DIRECTION ( 'NONE',  ( 0.000000000000000000, 0.000000000000000000, -1.000000000000000000 ) ) ;
#21321=FACE_OUTER_BOUND ( 'NONE', #8375, .T. ) ;
#21323=CARTESIAN_POINT ( 'NONE',  ( 34.99999999999980815, 39.97500000000000142, 54.99999999999922551 ) ) ;
#21324=CARTESIAN_POINT ( 'NONE',  ( -9.867969867547913054, 0.2954100743918419703, 54.30456930252528736 ) ) ;
#21325=CARTESIAN_POINT ( 'NONE',  ( -9.689843208404459673, 39.33333333333334991, -54.54983754392748807 ) ) ;
#21330=CARTESIAN_POINT ( 'NONE',  ( 9.689843208404422370, 39.33333333333334281, -54.54983754392748097 ) ) ;
#21332=ORIENTED_EDGE ( 'NONE', *, *, #14276, .F. ) ;
#21335=VERTEX_POINT ( 'NONE', #14465 ) ;
#21340=CARTESIAN_POINT ( 'NONE',  ( 3.803764550617159124, 39.91204985064339184, -51.45951652639460150 ) ) ;
#21341=CARTESIAN_POINT ( 'NONE',  ( 6.019227058680656661, 40.00000000000001421, 52.10376793666976170 ) ) ;
#21345=EDGE_LOOP ( 'NONE', ( #11700, #10385, #11619, #21623, #1836, #2682, #5429 ) ) ;
#21346=CARTESIAN_POINT ( 'NONE',  ( -2.587870662174074354, 0.1391398518287489672, 50.61865394279453767 ) ) ;
#21347=CARTESIAN_POINT ( 'NONE',  ( 4.664299542270204193E-14, -2.819653587506501857, 47.26169151849854444 ) ) ;
#21352=CARTESIAN_POINT ( 'NONE',  ( 3.171164708323686021, 39.94220383057359669, -51.05051439163197813 ) ) ;
#21356=EDGE_LOOP ( 'NONE', ( #5951, #14397, #2219, #515 ) ) ;
#21357=FACE_OUTER_BOUND ( 'NONE', #7616, .T. ) ;
#21360=CARTESIAN_POINT ( 'NONE',  ( 19.96591191796975551, 18.54839033250521751, 58.13845218884756605 ) ) ;
#21364=DIRECTION ( 'NONE',  ( -1.000000000000000000, 0.000000000000000000, 0.000000000000000000 ) ) ;
#21367=ORIENTED_EDGE ( 'NONE', *, *, #4464, .T. ) ;
#21369=VECTOR ( 'NONE', #14148, 1000.000000000000000 ) ;
#21377=ADVANCED_FACE ( 'NONE', ( #21357 ), #5030, .F. ) ;
#21383=CARTESIAN_POINT ( 'NONE',  ( -35.00000000000000000, -9.000000000000001776, -13.99999999999998579 ) ) ;
#21386=CARTESIAN_POINT ( 'NONE',  ( 13.00000000000024336, -2.516660498395250745, 105.0000000000000142 ) ) ;
#21387=AXIS2_PLACEMENT_3D ( 'NONE', #8508, #337, #15485 ) ;
#21389=CARTESIAN_POINT ( 'NONE',  ( -35.00000000000000000, 40.00000000000000000, 1.387778780781445676E-14 ) ) ;
#21390=CARTESIAN_POINT ( 'NONE',  ( -1.387778780781445518E-14, 20.00000000000000355, -105.0000000000000142 ) ) ;
#21391=VECTOR ( 'NONE', #3361, 1000.000000000000000 ) ;
#21401=CARTESIAN_POINT ( 'NONE',  ( -34.99999999999980815, 26.00000000000000355, 54.99999999999922551 ) ) ;
#21402=EDGE_CURVE ( 'NONE', #2004, #19351, #14000, .T. ) ;
#21404=DIRECTION ( 'NONE',  ( -0.000000000000000000, 1.000000000000000000, -0.000000000000000000 ) ) ;
#21405=CARTESIAN_POINT ( 'NONE',  ( -17.76477806472196974, 33.73774409953113462, -57.47211831788180803 ) ) ;
#21406=DIRECTION ( 'NONE',  ( 0.000000000000000000, 0.000000000000000000, 1.000000000000000000 ) ) ;
#21409=DIRECTION ( 'NONE',  ( -0.000000000000000000, -1.000000000000000000, -0.000000000000000000 ) ) ;
#21414=LINE ( 'NONE', #14407, #5665 ) ;
#21416=CARTESIAN_POINT ( 'NONE',  ( 14.89439646620657953, 6.624450698088172551, -59.14252023619225440 ) ) ;
#21417=CIRCLE ( 'NONE', #5313, 60.00000000000000000 ) ;
#21419=CYLINDRICAL_SURFACE ( 'NONE', #3452, 49.99999999999998579 ) ;
#21425=FACE_BOUND ( 'NONE', #4490, .T. ) ;
#21429=CARTESIAN_POINT ( 'NONE',  ( -9.744263423232260024, 2.495070046662454466, -54.63687069582701383 ) ) ;
#21431=DIRECTION ( 'NONE',  ( 0.000000000000000000, 0.000000000000000000, 1.000000000000000000 ) ) ;
#21434=CARTESIAN_POINT ( 'NONE',  ( -9.952189117650897643, 40.00000000000000000, 53.64426396172076039 ) ) ;
#21436=DIRECTION ( 'NONE',  ( 0.000000000000000000, -1.000000000000000000, 0.000000000000000000 ) ) ;
#21438=FACE_OUTER_BOUND ( 'NONE', #3961, .T. ) ;
#21439=CARTESIAN_POINT ( 'NONE',  ( -7.505578006075202424, 1.461761173328241181, 55.63523492904089096 ) ) ;
#21440=CARTESIAN_POINT ( 'NONE',  ( -0.5103191905027275599, 39.99845979207320568, -49.12706114568621985 ) ) ;
#21444=CARTESIAN_POINT ( 'NONE',  ( 34.99999999999980815, 40.00000000000000000, 52.49999999999922551 ) ) ;
#21452=ORIENTED_EDGE ( 'NONE', *, *, #19281, .F. ) ;
#21456=CARTESIAN_POINT ( 'NONE',  ( -90.00000000000000000, 26.00000000000000355, -9.108981535246192915E-16 ) ) ;
#21460=FACE_OUTER_BOUND ( 'NONE', #7129, .T. ) ;
#21463=CARTESIAN_POINT ( 'NONE',  ( -2.949288349266179665, -1.205118272524452916, 50.23218672884134861 ) ) ;
#21464=CIRCLE ( 'NONE', #17052, 20.00000000000000000 ) ;
#21467=EDGE_LOOP ( 'NONE', ( #9902, #6855, #12421, #12760 ) ) ;
#21468=CARTESIAN_POINT ( 'NONE',  ( 1.145276119296964268, 0.005126887279929492891, 49.65522505680549870 ) ) ;
#21470=CARTESIAN_POINT ( 'NONE',  ( 4.628075497661852999, 39.46063506869896997, 53.65703709785807263 ) ) ;
#21471=ADVANCED_FACE ( 'NONE', ( #21653 ), #4125, .F. ) ;
#21474=DIRECTION ( 'NONE',  ( -0.000000000000000000, -0.000000000000000000, -1.000000000000000000 ) ) ;
#21476=ORIENTED_EDGE ( 'NONE', *, *, #5407, .F. ) ;
#21477=CARTESIAN_POINT ( 'NONE',  ( 18.87679372942819001, 13.33229001579472417, 60.34430474298743263 ) ) ;
#21478=DIRECTION ( 'NONE',  ( -0.000000000000000000, -0.000000000000000000, -1.000000000000000000 ) ) ;
#21479=ADVANCED_FACE ( 'NONE', ( #16256 ), #13048, .F. ) ;
#21480=DIRECTION ( 'NONE',  ( 0.000000000000000000, 1.000000000000000000, 0.000000000000000000 ) ) ;
#21483=VERTEX_POINT ( 'NONE', #9397 ) ;
#21484=ORIENTED_EDGE ( 'NONE', *, *, #18522, .F. ) ;
#21486=DIRECTION ( 'NONE',  ( 0.000000000000000000, 0.000000000000000000, -1.000000000000000000 ) ) ;
#21494=ORIENTED_EDGE ( 'NONE', *, *, #7208, .F. ) ;
#21497=CARTESIAN_POINT ( 'NONE',  ( 29.99999999999998579, 20.00000000000000711, 105.0000000000000142 ) ) ;
#21504=CARTESIAN_POINT ( 'NONE',  ( -1.706267410340174185E-14, 40.00000000000000000, 48.73397172404484223 ) ) ;
#21515=CARTESIAN_POINT ( 'NONE',  ( -35.00000000000058265, 28.00000000000000000, -55.00000000000076028 ) ) ;
#21516=EDGE_CURVE ( 'NONE', #1894, #12579, #15988, .T. ) ;
#21517=DIRECTION ( 'NONE',  ( 0.000000000000000000, 0.000000000000000000, 1.000000000000000000 ) ) ;
#21518=CARTESIAN_POINT ( 'NONE',  ( 42.50000000000000711, -12.00000000000012434, 47.50000000000000711 ) ) ;
#21520=AXIS2_PLACEMENT_3D ( 'NONE', #12389, #125, #12600 ) ;
#21523=CARTESIAN_POINT ( 'NONE',  ( -13.88612301964757201, 34.41939562427583610, -58.78253654025285613 ) ) ;
#21529=CARTESIAN_POINT ( 'NONE',  ( -12.99999999999980282, -2.516660498395516310, 60.00099999999999767 ) ) ;
#21530=CARTESIAN_POINT ( 'NONE',  ( 34.99999999999980815, 40.00000000000000711, 52.47499999999922693 ) ) ;
#21531=CARTESIAN_POINT ( 'NONE',  ( 8.199064559763693083, 7.360541284256873595, -42.22991907770646947 ) ) ;
#21537=DIRECTION ( 'NONE',  ( -0.000000000000000000, -0.000000000000000000, 1.000000000000000000 ) ) ;
#21541=AXIS2_PLACEMENT_3D ( 'NONE', #12475, #17643, #5609 ) ;
#21542=EDGE_LOOP ( 'NONE', ( #15617, #16661, #451, #14651 ) ) ;
#21543=AXIS2_PLACEMENT_3D ( 'NONE', #3403, #1680, #5344 ) ;
#21545=CARTESIAN_POINT ( 'NONE',  ( 7.349642776635462837, 39.99999999999999289, -52.69668487371527732 ) ) ;
#21548=CARTESIAN_POINT ( 'NONE',  ( 4.274780932708218018, 39.88689858671455113, -51.75995564879541888 ) ) ;
#21553=CARTESIAN_POINT ( 'NONE',  ( -6.122940801430958757, 40.00000000000000000, 52.15215292453424922 ) ) ;
#21554=EDGE_LOOP ( 'NONE', ( #14773, #9417 ) ) ;
#21555=DIRECTION ( 'NONE',  ( -0.000000000000000000, -1.000000000000000000, -0.000000000000000000 ) ) ;
#21556=CARTESIAN_POINT ( 'NONE',  ( 42.50000000000000711, -5.000000000000000000, 47.50000000000000711 ) ) ;
#21560=DIRECTION ( 'NONE',  ( 0.000000000000000000, -1.000000000000000000, 0.000000000000000000 ) ) ;
#21562=CIRCLE ( 'NONE', #9488, 2.499999999999995115 ) ;
#21563=CARTESIAN_POINT ( 'NONE',  ( -9.075375600668062148, 39.43595020880619728, -54.33405310382095621 ) ) ;
#21566=CARTESIAN_POINT ( 'NONE',  ( -8.199064559763614923, 32.63945871574321700, 42.22991907770644104 ) ) ;
#21568=PRODUCT_DEFINITION_FORMATION_WITH_SPECIFIED_SOURCE ( 'ANY', '', #891, .NOT_KNOWN. ) ;
#21571=ORIENTED_EDGE ( 'NONE', *, *, #2720, .T. ) ;
#21578=CARTESIAN_POINT ( 'NONE',  ( -4.163336342344415913E-14, 40.00000000000002132, -48.73397172404479250 ) ) ;
#21580=LINE ( 'NONE', #2445, #17501 ) ;
#21581=ORIENTED_EDGE ( 'NONE', *, *, #21711, .F. ) ;
#21583=DIRECTION ( 'NONE',  ( -1.000000000000000000, 0.000000000000000000, 0.000000000000000000 ) ) ;
#21584=VERTEX_POINT ( 'NONE', #13371 ) ;
#21587=EDGE_CURVE ( 'NONE', #8689, #3941, #8328, .T. ) ;
#21588=LINE ( 'NONE', #1990, #20381 ) ;
#21589=ORIENTED_EDGE ( 'NONE', *, *, #17169, .T. ) ;
#21590=CARTESIAN_POINT ( 'NONE',  ( 1.591932335265033587E-15, -4.923002280079127832E-27, 50.50395615645412306 ) ) ;
#21591=ORIENTED_EDGE ( 'NONE', *, *, #11384, .T. ) ;
#21592=FACE_OUTER_BOUND ( 'NONE', #967, .T. ) ;
#21597=CARTESIAN_POINT ( 'NONE',  ( 15.13173276104727094, 33.09480349269512089, 56.64473394289761643 ) ) ;
#21598=CARTESIAN_POINT ( 'NONE',  ( 35.00000000000000000, -4.928932188134504955, 4.258610482196280173E-15 ) ) ;
#21599=CYLINDRICAL_SURFACE ( 'NONE', #1240, 2.099999999999997868 ) ;
#21600=VERTEX_POINT ( 'NONE', #6629 ) ;
#21603=ORIENTED_EDGE ( 'NONE', *, *, #8868, .F. ) ;
#21611=CARTESIAN_POINT ( 'NONE',  ( 35.00000000000000000, -4.999999999999997335, 4.258610482196280173E-15 ) ) ;
#21617=DIRECTION ( 'NONE',  ( 1.000000000000000000, 0.000000000000000000, -1.224646799147353207E-16 ) ) ;
#21623=ORIENTED_EDGE ( 'NONE', *, *, #20572, .F. ) ;
#21626=EDGE_CURVE ( 'NONE', #12299, #14267, #18584, .T. ) ;
#21628=ORIENTED_EDGE ( 'NONE', *, *, #7352, .F. ) ;
#21630=AXIS2_PLACEMENT_3D ( 'NONE', #18958, #6586, #3147 ) ;
#21631=CARTESIAN_POINT ( 'NONE',  ( 15.49999999999993960, 42.51666049839543149, -100.0000000000000000 ) ) ;
#21632=DIRECTION ( 'NONE',  ( 0.000000000000000000, 1.000000000000000000, 0.000000000000000000 ) ) ;
#21633=CARTESIAN_POINT ( 'NONE',  ( -12.09218358684866423, 1.291952833854532079, -55.42846997241218077 ) ) ;
#21634=CARTESIAN_POINT ( 'NONE',  ( -7.704815895020981742, 39.66337687413038537, -53.66058441934326595 ) ) ;
#21635=DIRECTION ( 'NONE',  ( -0.000000000000000000, -0.000000000000000000, -1.000000000000000000 ) ) ;
#21639=CARTESIAN_POINT ( 'NONE',  ( -4.589682443554583102, 39.46972628399738880, -53.62209933471819312 ) ) ;
#21644=VERTEX_POINT ( 'NONE', #20726 ) ;
#21646=CARTESIAN_POINT ( 'NONE',  ( -6.696867368503558448E-15, 40.00000000000000000, -48.73397172404479960 ) ) ;
#21648=EDGE_CURVE ( 'NONE', #19879, #18120, #17483, .T. ) ;
#21651=DIRECTION ( 'NONE',  ( -1.000000000000000000, 0.000000000000000000, 0.000000000000000000 ) ) ;
#21653=FACE_OUTER_BOUND ( 'NONE', #19300, .T. ) ;
#21654=EDGE_LOOP ( 'NONE', ( #6001, #5199 ) ) ;
#21655=CARTESIAN_POINT ( 'NONE',  ( 0.5260908555861737446, 39.99836280959126356, -49.13907560113233330 ) ) ;
#21658=ADVANCED_FACE ( 'NONE', ( #18671 ), #2976, .F. ) ;
#21663=CARTESIAN_POINT ( 'NONE',  ( -42.50000000000000711, -5.000000000000000000, 54.00000000000000711 ) ) ;
#21666=EDGE_LOOP ( 'NONE', ( #15229, #22315, #16569 ) ) ;
#21667=CARTESIAN_POINT ( 'NONE',  ( -42.50000000000000711, -12.00000000000000000, 47.50000000000000711 ) ) ;
#21675=ORIENTED_EDGE ( 'NONE', *, *, #20496, .T. ) ;
#21676=ORIENTED_EDGE ( 'NONE', *, *, #7110, .T. ) ;
#21678=EDGE_CURVE ( 'NONE', #2902, #2004, #19231, .T. ) ;
#21680=CARTESIAN_POINT ( 'NONE',  ( 17.23507576850065348, 30.19164414353179637, 59.89185441256822884 ) ) ;
#21682=VECTOR ( 'NONE', #16495, 1000.000000000000114 ) ;
#21689=CARTESIAN_POINT ( 'NONE',  ( -35.00000000000000000, 40.00000000000000000, 1.387778780781445676E-14 ) ) ;
#21691=ORIENTED_EDGE ( 'NONE', *, *, #10026, .F. ) ;
#21696=ORIENTED_EDGE ( 'NONE', *, *, #1151, .F. ) ;
#21697=CARTESIAN_POINT ( 'NONE',  ( -9.233659704009069102, 40.00000000000000000, -53.41795192421820104 ) ) ;
#21701=CARTESIAN_POINT ( 'NONE',  ( 7.704812602363275253, 39.66337197165110950, 53.66058689971939089 ) ) ;
#21703=ORIENTED_EDGE ( 'NONE', *, *, #18442, .T. ) ;
#21705=CARTESIAN_POINT ( 'NONE',  ( 16.86064470394643067, 34.83129639055714932, 57.19330778950707384 ) ) ;
#21706=CARTESIAN_POINT ( 'NONE',  ( -90.00000000000000000, 39.97500000000000142, 2.500000000000001332 ) ) ;
#21707=AXIS2_PLACEMENT_3D ( 'NONE', #2290, #9282, #16263 ) ;
#21708=CARTESIAN_POINT ( 'NONE',  ( 15.90155957501127304, 35.87083899979363366, -56.88316157031720621 ) ) ;
#21709=B_SPLINE_CURVE_WITH_KNOTS ( 'NONE', 3,
 ( #17957, #11188, #539, #2725, #16467, #9243, #2260, #14508 ),
 .UNSPECIFIED., .F., .F.,
 ( 4, 2, 2, 4 ),
 ( 0.000000000000000000, 0.002331395735520895053, 0.004662791471041790106, 0.009325582942083583682 ),
 .UNSPECIFIED. ) ;
#21710=ORIENTED_EDGE ( 'NONE', *, *, #9179, .T. ) ;
#21711=EDGE_CURVE ( 'NONE', #675, #21024, #17842, .T. ) ;
#21714=ORIENTED_EDGE ( 'NONE', *, *, #15340, .T. ) ;
#21716=CARTESIAN_POINT ( 'NONE',  ( -35.00000000000000000, -9.000000000000001776, 1.387778780781445676E-14 ) ) ;
#21717=B_SPLINE_CURVE_WITH_KNOTS ( 'NONE', 3,
 ( #3934, #16163, #6098, #11476, #16748, #13174, #14785, #720, #20191, #14893, #4611, #21920, #21680, #9871, #939, #4493, #12953, #16861, #21801, #14676, #13062, #22137, #20421, #18461 ),
 .UNSPECIFIED., .F., .F.,
 ( 4, 2, 2, 2, 2, 2, 2, 2, 2, 2, 2, 4 ),
 ( 0.01913044734024342899, 0.02058416378663299393, 0.02203788023302255886, 0.02494531312580169913, 0.02639902957219127447, 0.02785274601858084981, 0.03076017891135999355, 0.03221389535774956542, 0.03366761180413913035, 0.03657504469691827409, 0.03948247758969741089, 0.04238991048247654769 ),
 .UNSPECIFIED. ) ;
#21722=ORIENTED_EDGE ( 'NONE', *, *, #145, .F. ) ;
#21726=CARTESIAN_POINT ( 'NONE',  ( 10.49999999999994316, 42.51666049839543149, -105.0000000000000142 ) ) ;
#21729=DIRECTION ( 'NONE',  ( -0.000000000000000000, 1.000000000000000000, -0.000000000000000000 ) ) ;
#21732=CARTESIAN_POINT ( 'NONE',  ( -5.905688108141349701, 39.12130528552482644, 53.51375100093226678 ) ) ;
#21733=CARTESIAN_POINT ( 'NONE',  ( 35.00000000000000000, 40.00000000000000000, 4.258610482196280173E-15 ) ) ;
#21738=ORIENTED_EDGE ( 'NONE', *, *, #4105, .F. ) ;
#21742=DIRECTION ( 'NONE',  ( -0.000000000000000000, 1.000000000000000000, -0.000000000000000000 ) ) ;
#21743=CARTESIAN_POINT ( 'NONE',  ( -35.00000000000058265, 40.00000000000000711, -52.47500000000076170 ) ) ;
#21745=AXIS2_PLACEMENT_3D ( 'NONE', #13763, #441, #20779 ) ;
#21746=DIRECTION ( 'NONE',  ( -0.000000000000000000, 1.000000000000000000, -0.000000000000000000 ) ) ;
#21748=CARTESIAN_POINT ( 'NONE',  ( 7.325260514639500961E-15, -4.648749848371387827, 45.43309249825157536 ) ) ;
#21750=LINE ( 'NONE', #889, #13703 ) ;
#21753=AXIS2_PLACEMENT_3D ( 'NONE', #21886, #6185, #10990 ) ;
#21756=FACE_OUTER_BOUND ( 'NONE', #14092, .T. ) ;
#21760=AXIS2_PLACEMENT_3D ( 'NONE', #17175, #18789, #22585 ) ;
#21762=DIRECTION ( 'NONE',  ( -0.000000000000000000, 1.000000000000000000, -0.000000000000000000 ) ) ;
#21763=ORIENTED_EDGE ( 'NONE', *, *, #10185, .F. ) ;
#21770=CARTESIAN_POINT ( 'NONE',  ( 1.582593789249429506, 40.00000000000000000, -49.73343818203412070 ) ) ;
#21772=CARTESIAN_POINT ( 'NONE',  ( 9.689843208404422370, 39.33333333333334281, -54.54983754392748097 ) ) ;
#21773=CARTESIAN_POINT ( 'NONE',  ( 11.49398617736656014, 40.00000000000000711, 54.13866599136176916 ) ) ;
#21774=ADVANCED_FACE ( 'NONE', ( #317 ), #8805, .F. ) ;
#21776=CARTESIAN_POINT ( 'NONE',  ( 10.27431133777637484, -4.928932188134504955, -51.43682631505696179 ) ) ;
#21778=CARTESIAN_POINT ( 'NONE',  ( -14.70622169670557078, 6.333487747695555115, -56.50111465619737317 ) ) ;
#21780=DIRECTION ( 'NONE',  ( 0.000000000000000000, 0.000000000000000000, 1.000000000000000000 ) ) ;
#21781=ORIENTED_EDGE ( 'NONE', *, *, #22362, .T. ) ;
#21782=DIRECTION ( 'NONE',  ( 0.000000000000000000, 0.7071067811865352493, 0.7071067811865597852 ) ) ;
#21786=EDGE_CURVE ( 'NONE', #507, #164, #12711, .T. ) ;
#21788=ADVANCED_FACE ( 'NONE', ( #10843 ), #14042, .F. ) ;
#21791=CARTESIAN_POINT ( 'NONE',  ( -5.833333333333328596, 33.81926995981417861, 40.61164310337068173 ) ) ;
#21793=EDGE_CURVE ( 'NONE', #17279, #4267, #21709, .T. ) ;
#21800=VERTEX_POINT ( 'NONE', #773 ) ;
#21801=CARTESIAN_POINT ( 'NONE',  ( 13.65693838750919120, 34.64075751992691465, 58.69913499740202667 ) ) ;
#21802=AXIS2_PLACEMENT_3D ( 'NONE', #13747, #6905, #13967 ) ;
#21803=CARTESIAN_POINT ( 'NONE',  ( 4.842578813362819368, -0.8535550256951374148, 51.47191290771596783 ) ) ;
#21810=CARTESIAN_POINT ( 'NONE',  ( -12.99999999999980282, -2.516660498395516310, 105.0000000000000142 ) ) ;
#21812=CARTESIAN_POINT ( 'NONE',  ( -13.59841332577231832, 13.65742718326612604, -45.18857684126742669 ) ) ;
#21813=CARTESIAN_POINT ( 'NONE',  ( 9.594672135725315573E-15, 39.99999999999997158, 48.73397172404484223 ) ) ;
#21816=VERTEX_POINT ( 'NONE', #10964 ) ;
#21817=CARTESIAN_POINT ( 'NONE',  ( 0.7060532431912704965, 40.00000000000297717, 49.41655072425569983 ) ) ;
#21820=CARTESIAN_POINT ( 'NONE',  ( -7.864084088052238365E-15, -0.02545116923825692726, -50.05029972084987122 ) ) ;
#21823=AXIS2_PLACEMENT_3D ( 'NONE', #14940, #1101, #6145 ) ;
#21830=FACE_BOUND ( 'NONE', #16410, .T. ) ;
#21833=EDGE_CURVE ( 'NONE', #15580, #2477, #14621, .T. ) ;
#21838=ORIENTED_EDGE ( 'NONE', *, *, #8801, .F. ) ;
#21840=CARTESIAN_POINT ( 'NONE',  ( -34.99999999999999289, 40.00000000000000000, 58.99999999999995737 ) ) ;
#21843=CARTESIAN_POINT ( 'NONE',  ( 11.68090480754630178, 3.765577839755386069, 57.90797000640142045 ) ) ;
#21844=DIRECTION ( 'NONE',  ( 0.000000000000000000, 0.000000000000000000, 1.000000000000000000 ) ) ;
#21845=ORIENTED_EDGE ( 'NONE', *, *, #19705, .F. ) ;
#21846=AXIS2_PLACEMENT_3D ( 'NONE', #2255, #14266, #16220 ) ;
#21847=ORIENTED_EDGE ( 'NONE', *, *, #9711, .T. ) ;
#21851=CARTESIAN_POINT ( 'NONE',  ( -0.4054897353551412120, 39.99903132614927159, 49.04700738630989321 ) ) ;
#21852=AXIS2_PLACEMENT_3D ( 'NONE', #4818, #13384, #16848 ) ;
#21853=EDGE_CURVE ( 'NONE', #19371, #19744, #10520, .T. ) ;
#21854=CARTESIAN_POINT ( 'NONE',  ( -0.7832310603219697631, 40.00000000000097344, 49.34583618815681660 ) ) ;
#21856=EDGE_LOOP ( 'NONE', ( #2625, #13054, #20325, #8787 ) ) ;
#21857=CONICAL_SURFACE ( 'NONE', #16311, 2.524999999999999467, 0.7853981633974482790 ) ;
#21858=VERTEX_POINT ( 'NONE', #21631 ) ;
#21859=ORIENTED_EDGE ( 'NONE', *, *, #357, .F. ) ;
#21860=CARTESIAN_POINT ( 'NONE',  ( -17.96553007763869658, 11.19640018278690263, 57.57421575614280584 ) ) ;
#21861=CARTESIAN_POINT ( 'NONE',  ( -1.039655021832667670, -3.147609295952975561, -46.52691668518789214 ) ) ;
#21863=CARTESIAN_POINT ( 'NONE',  ( 0.6844983420876992186, -1.267142481712868474, -48.72692999688269566 ) ) ;
#21867=CARTESIAN_POINT ( 'NONE',  ( -5.833333333333339255, 40.00000000000000000, -40.61164310337066041 ) ) ;
#21869=CARTESIAN_POINT ( 'NONE',  ( -6.433485051969688229, 38.94088993357593154, -55.16018527339667088 ) ) ;
#21871=ADVANCED_FACE ( 'NONE', ( #18299, #5818 ), #7995, .F. ) ;
#21874=DIRECTION ( 'NONE',  ( -0.000000000000000000, -1.000000000000000000, -0.000000000000000000 ) ) ;
#21875=CARTESIAN_POINT ( 'NONE',  ( 15.49999999999993960, 42.51666049839543149, 105.0000000000000142 ) ) ;
#21876=CARTESIAN_POINT ( 'NONE',  ( 16.23901130406737181, 8.288052467682684110, 57.02826995000636146 ) ) ;
#21877=DIRECTION ( 'NONE',  ( -0.000000000000000000, 1.000000000000000000, -0.000000000000000000 ) ) ;
#21879=CARTESIAN_POINT ( 'NONE',  ( -1.387778780781445676E-14, 40.00000000000000000, -48.73397172404481381 ) ) ;
#21886=CARTESIAN_POINT ( 'NONE',  ( -13.00000000000011546, 42.51666049839536043, 100.0000000000000000 ) ) ;
#21887=AXIS2_PLACEMENT_3D ( 'NONE', #18544, #15078, #2967 ) ;
#21890=ORIENTED_EDGE ( 'NONE', *, *, #21082, .T. ) ;
#21892=AXIS2_PLACEMENT_3D ( 'NONE', #13256, #13377, #6192 ) ;
#21893=CARTESIAN_POINT ( 'NONE',  ( 10.43027093729392618, 39.22757009021464114, 54.80615623442351847 ) ) ;
#21894=AXIS2_PLACEMENT_3D ( 'NONE', #16100, #10708, #10487 ) ;
#21896=B_SPLINE_CURVE_WITH_KNOTS ( 'NONE', 3,
 ( #1992, #3617, #17803, #3384, #13782, #6937, #10461, #7144, #12086, #22523, #12189, #20798 ),
 .UNSPECIFIED., .F., .F.,
 ( 4, 2, 2, 2, 2, 4 ),
 ( 0.006347202264228477345, 0.007930096811551049646, 0.008721544085212338399, 0.009512991358873625417, 0.01109588590619620292, 0.01267878045351878216 ),
 .UNSPECIFIED. ) ;
#21897=CARTESIAN_POINT ( 'NONE',  ( -2.734690830816374874, 39.99999999999998579, 50.39884290491228569 ) ) ;
#21898=DIRECTION ( 'NONE',  ( -0.000000000000000000, -1.000000000000000000, -0.000000000000000000 ) ) ;
#21899=CARTESIAN_POINT ( 'NONE',  ( -9.454382208758131512, 39.37264146017265176, 54.46710161869616940 ) ) ;
#21905=CARTESIAN_POINT ( 'NONE',  ( -0.03494506074407652957, 39.99999280907451293, -48.76115732596038299 ) ) ;
#21908=CARTESIAN_POINT ( 'NONE',  ( -14.94062893683336668, 21.54390686295445079, 45.79998742252197275 ) ) ;
#21909=DIRECTION ( 'NONE',  ( -0.000000000000000000, -1.000000000000000000, -0.000000000000000000 ) ) ;
#21913=VECTOR ( 'NONE', #7561, 1000.000000000000114 ) ;
#21915=ORIENTED_EDGE ( 'NONE', *, *, #22285, .F. ) ;
#21918=ADVANCED_FACE ( 'NONE', ( #16350 ), #7652, .T. ) ;
#21919=ORIENTED_EDGE ( 'NONE', *, *, #22501, .F. ) ;
#21920=CARTESIAN_POINT ( 'NONE',  ( 17.70396115872092935, 29.35428329955200866, 60.02641142872583657 ) ) ;
#21923=CYLINDRICAL_SURFACE ( 'NONE', #9441, 2.499999999999998668 ) ;
#21925=ORIENTED_EDGE ( 'NONE', *, *, #4723, .F. ) ;
#21926=DIRECTION ( 'NONE',  ( -0.000000000000000000, 1.000000000000000000, -0.000000000000000000 ) ) ;
#21928=CIRCLE ( 'NONE', #13117, 18.00000000000000000 ) ;
#21930=DIRECTION ( 'NONE',  ( -0.000000000000000000, 1.000000000000000000, -0.000000000000000000 ) ) ;
#21931=CARTESIAN_POINT ( 'NONE',  ( -19.47136665037378833, 8.793048248091416497, -57.95785196855348431 ) ) ;
#21932=FACE_OUTER_BOUND ( 'NONE', #1403, .T. ) ;
#21933=ORIENTED_EDGE ( 'NONE', *, *, #16695, .F. ) ;
#21935=CARTESIAN_POINT ( 'NONE',  ( 6.401811138932578693, 38.95166772950821610, -55.13648753466789287 ) ) ;
#21937=CARTESIAN_POINT ( 'NONE',  ( 7.555723902516218615, 38.52224445567402711, 55.93227658743226272 ) ) ;
#21940=CARTESIAN_POINT ( 'NONE',  ( -0.3713120412951391169, -0.009378283650370923194, -50.78681545405707709 ) ) ;
#21943=CARTESIAN_POINT ( 'NONE',  ( 9.165377225651162973, 37.79989650906291132, 54.16098472236621575 ) ) ;
#21946=CARTESIAN_POINT ( 'NONE',  ( 18.09042992579335163, 28.57522027848957080, -57.61279183054943331 ) ) ;
#21958=CARTESIAN_POINT ( 'NONE',  ( 10.99584631063691909, 3.272668205460111945, 57.61971594758629323 ) ) ;
#21965=CARTESIAN_POINT ( 'NONE',  ( 15.50000000000024336, -2.516660498395250745, 100.0000000000000000 ) ) ;
#21968=CARTESIAN_POINT ( 'NONE',  ( 35.00000000000058265, 28.00000000000000000, -55.00000000000076028 ) ) ;
#21969=CARTESIAN_POINT ( 'NONE',  ( -0.1964574450121475135, 39.99977788120574473, 48.88630899457443491 ) ) ;
#21971=AXIS2_PLACEMENT_3D ( 'NONE', #6659, #3459, #20636 ) ;
#21972=CARTESIAN_POINT ( 'NONE',  ( -11.13407802442741534, 9.941921282207673016, 43.93745127716451293 ) ) ;
#21975=ORIENTED_EDGE ( 'NONE', *, *, #12527, .F. ) ;
#21977=ORIENTED_EDGE ( 'NONE', *, *, #12978, .T. ) ;
#21978=CARTESIAN_POINT ( 'NONE',  ( -17.11943327291902150, 30.37830191768460963, 59.85657255524080966 ) ) ;
#21980=CARTESIAN_POINT ( 'NONE',  ( 37.10000000000058407, 28.00000000000000000, -55.00000000000076028 ) ) ;
#21981=EDGE_CURVE ( 'NONE', #3437, #19781, #9817, .T. ) ;
#21983=CARTESIAN_POINT ( 'NONE',  ( 35.00000000000000000, 0.000000000000000000, -9.000000000000000000 ) ) ;
#21984=CARTESIAN_POINT ( 'NONE',  ( 0.6237373291636730821, 39.99088417130652573, 49.47180386667442775 ) ) ;
#21986=CARTESIAN_POINT ( 'NONE',  ( -6.297060429293823702, 38.99690089842329854, -53.73986014815309886 ) ) ;
#21990=CARTESIAN_POINT ( 'NONE',  ( -10.64189282879911147, 39.19489805854265541, 54.88474174651651794 ) ) ;
#21991=CYLINDRICAL_SURFACE ( 'NONE', #15897, 60.00000000000000000 ) ;
#21993=ORIENTED_EDGE ( 'NONE', *, *, #11404, .F. ) ;
#21994=ORIENTED_EDGE ( 'NONE', *, *, #13506, .T. ) ;
#21995=CARTESIAN_POINT ( 'NONE',  ( -35.00000000000000000, 25.00000000000000000, 9.000000000000015987 ) ) ;
#21997=AXIS2_PLACEMENT_3D ( 'NONE', #5907, #16443, #753 ) ;
#22000=CARTESIAN_POINT ( 'NONE',  ( 8.640968485947571054, 40.00000000000000000, -53.20846482585461246 ) ) ;
#22001=ORIENTED_EDGE ( 'NONE', *, *, #21981, .F. ) ;
#22006=CARTESIAN_POINT ( 'NONE',  ( -9.579024991656989840, 31.54842267267897427, -43.05667825653219438 ) ) ;
#22011=CARTESIAN_POINT ( 'NONE',  ( 8.349099696861287612, 1.803277857259548034, -53.93591755799870668 ) ) ;
#22016=EDGE_CURVE ( 'NONE', #2374, #11218, #13088, .T. ) ;
#22017=AXIS2_PLACEMENT_3D ( 'NONE', #5604, #5499, #14417 ) ;
#22020=ORIENTED_EDGE ( 'NONE', *, *, #3031, .T. ) ;
#22024=CARTESIAN_POINT ( 'NONE',  ( 13.63965147459808946, 34.63504322468456564, -58.68815147418791867 ) ) ;
#22027=CARTESIAN_POINT ( 'NONE',  ( 15.34286839272954950, 7.164559734098753019, 59.29291272740924512 ) ) ;
#22028=CARTESIAN_POINT ( 'NONE',  ( 5.422195817667230244, 6.007182364969045452, -40.31637036980818323 ) ) ;
#22033=CARTESIAN_POINT ( 'NONE',  ( -14.52224280010138102, 16.16745304956414842, -45.61498238574513664 ) ) ;
#22036=CARTESIAN_POINT ( 'NONE',  ( 18.48876241336177983, 12.20729522219678920, -60.24712676880312046 ) ) ;
#22037=ORIENTED_EDGE ( 'NONE', *, *, #1802, .F. ) ;
#22038=CARTESIAN_POINT ( 'NONE',  ( -7.552830808693327569, 40.00000000000000000, -52.78252196372452687 ) ) ;
#22039=EDGE_CURVE ( 'NONE', #20199, #6208, #636, .T. ) ;
#22040=( BOUNDED_SURFACE ( )  B_SPLINE_SURFACE ( 3, 2, ( 
 ( #9, #1731, #15695 ),
 ( #7001, #13956, #7874 ),
 ( #4103, #3998, #11073 ),
 ( #16468, #774, #19802 ),
 ( #19907, #14728, #18063 ),
 ( #20027, #4334, #16693 ),
 ( #882, #18405, #21863 ),
 ( #11314, #18300, #7653 ) ),
 .UNSPECIFIED., .F., .F., .F. ) 
 B_SPLINE_SURFACE_WITH_KNOTS ( ( 4, 2, 2, 4 ),
 ( 3, 3 ),
 ( -2.168404344971008868E-18, 0.005619572794283482498, 0.008429359191425223746, 0.01123914558856696673 ),
 ( 0.000000000000000000, 1.000000000000000000 ),
 .UNSPECIFIED. ) 
 GEOMETRIC_REPRESENTATION_ITEM ( )  RATIONAL_B_SPLINE_SURFACE ( (
 ( 1.000000000000000000, 0.7200096751079135826, 1.000000000000000000),
 ( 1.000000000000000000, 0.7496815117904079839, 1.000000000000000000),
 ( 1.000000000000000000, 0.7737746244339125390, 1.000000000000000000),
 ( 1.000000000000000000, 0.8024243379864889336, 1.000000000000000000),
 ( 1.000000000000000000, 0.8107154503870998008, 1.000000000000000000),
 ( 1.000000000000000000, 0.8248921579234514967, 1.000000000000000000),
 ( 1.000000000000000000, 0.8307774003434091892, 1.000000000000000000),
 ( 1.000000000000000000, 0.8354972176269009898, 1.000000000000000000) ) ) 
 REPRESENTATION_ITEM ( '' )  SURFACE ( )  );
#22041=CARTESIAN_POINT ( 'NONE',  ( 4.589505318347391949, 39.46976832855466455, -53.62193830992116261 ) ) ;
#22043=CARTESIAN_POINT ( 'NONE',  ( 42.50000000000000711, -12.00000000000012434, -50.02500000000011227 ) ) ;
#22044=CARTESIAN_POINT ( 'NONE',  ( -2.995584608082017652, -1.237002266245721405, 50.27666343020542428 ) ) ;
#22047=CARTESIAN_POINT ( 'NONE',  ( 8.331955809010597847, 38.18181818181818699, 56.36098470834072316 ) ) ;
#22049=EDGE_CURVE ( 'NONE', #19899, #14723, #17121, .T. ) ;
#22050=CARTESIAN_POINT ( 'NONE',  ( 19.96824854984769004, 18.58379861519964393, -58.13906733436663643 ) ) ;
#22054=ORIENTED_EDGE ( 'NONE', *, *, #20243, .T. ) ;
#22057=CARTESIAN_POINT ( 'NONE',  ( 10.80340688045851216, 39.17018323811936398, 54.94414022070431258 ) ) ;
#22059=ORIENTED_EDGE ( 'NONE', *, *, #16328, .F. ) ;
#22061=CARTESIAN_POINT ( 'NONE',  ( -34.99999999999980815, 26.00000000000000355, 54.99999999999922551 ) ) ;
#22062=EDGE_LOOP ( 'NONE', ( #13271, #19510 ) ) ;
#22069=B_SPLINE_CURVE_WITH_KNOTS ( 'NONE', 3,
 ( #9552, #11719, #21820, #6118, #13081, #1290, #2917, #11497, #20100, #8284 ),
 .UNSPECIFIED., .F., .F.,
 ( 4, 2, 2, 2, 4 ),
 ( -8.975271422312889897E-06, 0.0006698366896151128867, 0.001348648650652538826, 0.002027460611689964332, 0.002706272572727390271 ),
 .UNSPECIFIED. ) ;
#22074=EDGE_CURVE ( 'NONE', #15024, #8759, #14017, .T. ) ;
#22075=AXIS2_PLACEMENT_3D ( 'NONE', #7275, #390, #7386 ) ;
#22079=EDGE_CURVE ( 'NONE', #17839, #790, #6840, .T. ) ;
#22081=CARTESIAN_POINT ( 'NONE',  ( -19.27753112432710481, 25.39788459339701987, 57.95296232962699179 ) ) ;
#22082=FACE_OUTER_BOUND ( 'NONE', #10891, .T. ) ;
#22086=CARTESIAN_POINT ( 'NONE',  ( 42.50000000000000711, -9.600000000000001421, -47.50000000000000000 ) ) ;
#22090=ORIENTED_EDGE ( 'NONE', *, *, #12206, .T. ) ;
#22092=CARTESIAN_POINT ( 'NONE',  ( -4.997499695308150081E-15, -0.2027466127521987682, 49.39731220485085572 ) ) ;
#22094=CARTESIAN_POINT ( 'NONE',  ( -8.331955809010668901, 38.18181818181816567, -56.36098470834073737 ) ) ;
#22095=FACE_OUTER_BOUND ( 'NONE', #7048, .T. ) ;
#22096=VERTEX_POINT ( 'NONE', #5879 ) ;
#22100=B_SPLINE_CURVE_WITH_KNOTS ( 'NONE', 3,
 ( #8340, #10044, #11769, #6737, #13242, #16712, #2742, #8454, #2857, #15314 ),
 .UNSPECIFIED., .F., .F.,
 ( 4, 2, 2, 2, 4 ),
 ( 0.000000000000000000, 0.002975785561748156127, 0.005951571123496312253, 0.008927356685244467946, 0.01190314224699262451 ),
 .UNSPECIFIED. ) ;
#22102=DIRECTION ( 'NONE',  ( 0.000000000000000000, 0.000000000000000000, 1.000000000000000000 ) ) ;
#22105=AXIS2_PLACEMENT_3D ( 'NONE', #3775, #10981, #19814 ) ;
#22108=EDGE_LOOP ( 'NONE', ( #12941, #6431 ) ) ;
#22109=EDGE_CURVE ( 'NONE', #4439, #15664, #14253, .T. ) ;
#22111=CARTESIAN_POINT ( 'NONE',  ( -42.50000000000000711, -12.00000000000012434, 44.97499999999989484 ) ) ;
#22117=CARTESIAN_POINT ( 'NONE',  ( -9.689843208404459673, 39.33333333333334991, -54.54983754392748807 ) ) ;
#22127=AXIS2_PLACEMENT_3D ( 'NONE', #16978, #11492, #20436 ) ;
#22128=CARTESIAN_POINT ( 'NONE',  ( -28.50000000000001421, 19.99999999999982947, -105.0000000000000142 ) ) ;
#22129=CARTESIAN_POINT ( 'NONE',  ( -10.50000000000012079, 42.51666049839536043, -105.0000000000000142 ) ) ;
#22130=CIRCLE ( 'NONE', #15150, 2.500000000000002220 ) ;
#22137=CARTESIAN_POINT ( 'NONE',  ( 9.940687323067940895, 37.37897894777886876, 57.14641600008368982 ) ) ;
#22140=CYLINDRICAL_SURFACE ( 'NONE', #6504, 2.499999999999995115 ) ;
#22143=ORIENTED_EDGE ( 'NONE', *, *, #17587, .F. ) ;
#22153=DIRECTION ( 'NONE',  ( -0.000000000000000000, 1.000000000000000000, -0.000000000000000000 ) ) ;
#22155=CARTESIAN_POINT ( 'NONE',  ( 7.505578006075174891, 1.461761173328240071, -55.63523492904086254 ) ) ;
#22156=VERTEX_POINT ( 'NONE', #3520 ) ;
#22158=EDGE_CURVE ( 'NONE', #3688, #5859, #21580, .T. ) ;
#22162=VECTOR ( 'NONE', #16499, 1000.000000000000000 ) ;
#22163=CARTESIAN_POINT ( 'NONE',  ( 19.23518390577179105, 25.54875756131788123, -60.43569366689261813 ) ) ;
#22170=( BOUNDED_SURFACE ( )  B_SPLINE_SURFACE ( 3, 2, ( 
 ( #13063, #16964, #3003 ),
 ( #8265, #11247, #18245 ),
 ( #2556, #11362, #9535 ),
 ( #821, #7811, #14786 ),
 ( #21803, #19039, #8718 ),
 ( #19148, #18921, #10197 ),
 ( #6658, #19265, #1389 ),
 ( #3568, #8825, #15796 ),
 ( #17190, #15351, #3346 ),
 ( #1502, #5285, #22599 ) ),
 .UNSPECIFIED., .F., .F., .F. ) 
 B_SPLINE_SURFACE_WITH_KNOTS ( ( 4, 2, 2, 2, 4 ),
 ( 3, 3 ),
 ( 0.02809317535148810746, 0.03071213539477267440, 0.03333109543805724134, 0.03595005548134180828, 0.03856901552462637522 ),
 ( 0.2389732943673020804, 1.000000000000000000 ),
 .UNSPECIFIED. ) 
 GEOMETRIC_REPRESENTATION_ITEM ( )  RATIONAL_B_SPLINE_SURFACE ( (
 ( 0.9723126933862670240, 0.9420702913958711733, 1.000000000000000000),
 ( 0.9749922925144016705, 0.9476767737754799859, 1.000000000000000000),
 ( 0.9774153414777251303, 0.9527464803503058466, 1.000000000000000000),
 ( 0.9815341666525440045, 0.9613642323583782012, 1.000000000000000000),
 ( 0.9832251939808056562, 0.9649023417792208512, 1.000000000000000000),
 ( 0.9856873122312799218, 0.9700537923984060562, 1.000000000000000000),
 ( 0.9864553338148209782, 0.9716607116685581635, 1.000000000000000000),
 ( 0.9870557760262803626, 0.9729170072999364649, 1.000000000000000000),
 ( 0.9868934176577699446, 0.9725773074833932164, 1.000000000000000000),
 ( 0.9863383242652692395, 0.9714158944602974133, 1.000000000000000000) ) ) 
 REPRESENTATION_ITEM ( '' )  SURFACE ( )  );
#22176=EDGE_CURVE ( 'NONE', #2120, #20382, #5457, .T. ) ;
#22178=AXIS2_PLACEMENT_3D ( 'NONE', #14022, #1806, #15760 ) ;
#22182=DIRECTION ( 'NONE',  ( 0.000000000000000000, 0.000000000000000000, 1.000000000000000000 ) ) ;
#22184=FACE_OUTER_BOUND ( 'NONE', #21356, .T. ) ;
#22186=CARTESIAN_POINT ( 'NONE',  ( -0.2661007013785012809, 39.99958209025860612, 48.93999295480112721 ) ) ;
#22188=CARTESIAN_POINT ( 'NONE',  ( -15.00000000000001421, 20.00000000000000355, 45.82575694955841072 ) ) ;
#22189=AXIS2_PLACEMENT_3D ( 'NONE', #21401, #319, #2037 ) ;
#22190=AXIS2_PLACEMENT_3D ( 'NONE', #19219, #15864, #9438 ) ;
#22193=CIRCLE ( 'NONE', #592, 2.499999999999995115 ) ;
#22194=VERTEX_POINT ( 'NONE', #10482 ) ;
#22197=CARTESIAN_POINT ( 'NONE',  ( -17.57556337525805290, 10.44046169743836217, 57.45538260706025824 ) ) ;
#22198=CIRCLE ( 'NONE', #18888, 6.499999999999999112 ) ;
#22200=CARTESIAN_POINT ( 'NONE',  ( -19.80807096600700845, 16.80592363802972145, -60.57763526510198915 ) ) ;
#22201=CARTESIAN_POINT ( 'NONE',  ( 7.031141211283101100, 39.67715641065061760, 53.36152252427557130 ) ) ;
#22202=EDGE_CURVE ( 'NONE', #10068, #18961, #8883, .T. ) ;
#22205=ORIENTED_EDGE ( 'NONE', *, *, #5943, .F. ) ;
#22207=CARTESIAN_POINT ( 'NONE',  ( -35.00000000000000000, 0.000000000000000000, 1.387778780781445676E-14 ) ) ;
#22212=CARTESIAN_POINT ( 'NONE',  ( -11.86180952234344588, 38.99999999999292299, 55.35904751185378103 ) ) ;
#22213=CARTESIAN_POINT ( 'NONE',  ( 14.70622169671638169, 6.333487747693914649, 56.50111465620437912 ) ) ;
#22217=DIRECTION ( 'NONE',  ( -0.7752116086454780008, 0.5577761202038526989, -0.2965345874457614439 ) ) ;
#22219=CARTESIAN_POINT ( 'NONE',  ( 6.696867368502865039E-15, 35.00000000000000000, 38.73397172404480671 ) ) ;
#22221=EDGE_LOOP ( 'NONE', ( #5188, #1868, #16992, #9002 ) ) ;
#22224=AXIS2_PLACEMENT_3D ( 'NONE', #11082, #5587, #11199 ) ;
#22226=CARTESIAN_POINT ( 'NONE',  ( -6.674721970908912283, -4.820493483656560052, 49.68071724292274638 ) ) ;
#22227=CARTESIAN_POINT ( 'NONE',  ( -1.387778780781445676E-14, 20.00000000000000000, 102.0000000000000142 ) ) ;
#22232=CARTESIAN_POINT ( 'NONE',  ( -18.64599517736102996, 12.71385791664993370, -57.77541544179386790 ) ) ;
#22234=CARTESIAN_POINT ( 'NONE',  ( -8.553361841769476115, 39.50247004197922251, 54.09836511283659632 ) ) ;
#22236=DIRECTION ( 'NONE',  ( 0.9012767464701764153, 6.280369834735124333E-16, -0.4332438415859287129 ) ) ;
#22238=CARTESIAN_POINT ( 'NONE',  ( 13.59841332577230411, 26.34257281673386686, 45.18857684126744090 ) ) ;
#22241=FACE_OUTER_BOUND ( 'NONE', #16438, .T. ) ;
#22243=AXIS2_PLACEMENT_3D ( 'NONE', #7088, #12028, #13842 ) ;
#22246=CARTESIAN_POINT ( 'NONE',  ( 5.010575289839681368, 5.833430802647523450, 40.02075074423078149 ) ) ;
#22250=CIRCLE ( 'NONE', #5061, 2.099999999999997868 ) ;
#22255=PLANE ( 'NONE',  #14687 ) ;
#22257=CARTESIAN_POINT ( 'NONE',  ( 35.00000000000000000, 25.00000000000000000, 4.258610482196280173E-15 ) ) ;
#22258=DIRECTION ( 'NONE',  ( -0.000000000000000000, 1.000000000000000000, -0.000000000000000000 ) ) ;
#22259=CARTESIAN_POINT ( 'NONE',  ( -12.99999999999980282, -2.516660498395516310, 105.0000000000000142 ) ) ;
#22262=DIRECTION ( 'NONE',  ( 1.000000000000000000, 0.000000000000000000, 0.000000000000000000 ) ) ;
#22263=ORIENTED_EDGE ( 'NONE', *, *, #10026, .T. ) ;
#22264=CARTESIAN_POINT ( 'NONE',  ( -7.017626609043932540, 6.725442770851636887, -41.44244536674932533 ) ) ;
#22265=EDGE_CURVE ( 'NONE', #15997, #17185, #7937, .T. ) ;
#22268=CARTESIAN_POINT ( 'NONE',  ( -1.387778780781494900E-14, 40.00000000000002132, 48.73397172404481381 ) ) ;
#22269=EDGE_LOOP ( 'NONE', ( #13309, #3369, #18178 ) ) ;
#22273=DIRECTION ( 'NONE',  ( 0.000000000000000000, 0.000000000000000000, -1.000000000000000000 ) ) ;
#22274=CARTESIAN_POINT ( 'NONE',  ( -19.73349596156088381, 30.70641346160536855, 58.02568834892373673 ) ) ;
#22276=ORIENTED_EDGE ( 'NONE', *, *, #2366, .T. ) ;
#22277=DIRECTION ( 'NONE',  ( 0.000000000000000000, 0.000000000000000000, 1.000000000000000000 ) ) ;
#22279=EDGE_CURVE ( 'NONE', #14544, #19784, #6158, .T. ) ;
#22280=VECTOR ( 'NONE', #7060, 1000.000000000000000 ) ;
#22283=VECTOR ( 'NONE', #17597, 1000.000000000000000 ) ;
#22284=CARTESIAN_POINT ( 'NONE',  ( 19.98434069128079216, 21.18673122687495436, -60.61816909401677123 ) ) ;
#22285=EDGE_CURVE ( 'NONE', #8864, #19508, #15909, .T. ) ;
#22286=ORIENTED_EDGE ( 'NONE', *, *, #13080, .T. ) ;
#22288=ORIENTED_EDGE ( 'NONE', *, *, #4464, .F. ) ;
#22290=ORIENTED_EDGE ( 'NONE', *, *, #3104, .T. ) ;
#22291=AXIS2_PLACEMENT_3D ( 'NONE', #19043, #13862, #18927 ) ;
#22292=( NAMED_UNIT ( * ) SI_UNIT ( $, .STERADIAN. ) SOLID_ANGLE_UNIT ( ) );
#22294=DIRECTION ( 'NONE',  ( 0.000000000000000000, -1.000000000000000000, 0.000000000000000000 ) ) ;
#22297=ADVANCED_FACE ( 'NONE', ( #12959 ), #2516, .F. ) ;
#22298=CARTESIAN_POINT ( 'NONE',  ( -34.99999999999999289, 40.00000000000000000, 50.00000000000000000 ) ) ;
#22299=ORIENTED_EDGE ( 'NONE', *, *, #3851, .T. ) ;
#22303=AXIS2_PLACEMENT_3D ( 'NONE', #1392, #22602, #10307 ) ;
#22305=ORIENTED_EDGE ( 'NONE', *, *, #20625, .F. ) ;
#22306=FACE_BOUND ( 'NONE', #5757, .T. ) ;
#22307=DIRECTION ( 'NONE',  ( -0.000000000000000000, -0.000000000000000000, -1.000000000000000000 ) ) ;
#22308=CARTESIAN_POINT ( 'NONE',  ( -2.836563456948004695E-15, -1.236374842841498678, -48.24164917503444627 ) ) ;
#22309=CARTESIAN_POINT ( 'NONE',  ( -0.2763205028094647964, 39.99954928602512894, 48.94785969531869085 ) ) ;
#22311=AXIS2_PLACEMENT_3D ( 'NONE', #3008, #13283, #20197 ) ;
#22312=CARTESIAN_POINT ( 'NONE',  ( -5.833333333333327708, 6.180730040185831164, 40.61164310337068173 ) ) ;
#22315=ORIENTED_EDGE ( 'NONE', *, *, #17587, .T. ) ;
#22317=( BOUNDED_SURFACE ( )  B_SPLINE_SURFACE ( 3, 2, ( 
 ( #2862, #12015, #17047 ),
 ( #13249, #15203, #9846 ),
 ( #13587, #16834, #22449 ),
 ( #6742, #13708, #20724 ),
 ( #4913, #15087, #1135 ),
 ( #10165, #20498, #11889 ),
 ( #4804, #8348, #22226 ),
 ( #8127, #15321, #18776 ),
 ( #1474, #5033, #20391 ),
 ( #22342, #11773, #6405 ) ),
 .UNSPECIFIED., .F., .F., .F. ) 
 B_SPLINE_SURFACE_WITH_KNOTS ( ( 4, 2, 2, 2, 4 ),
 ( 3, 3 ),
 ( 0.02858426235558113315, 0.03123866089385130690, 0.03389305943212148065, 0.03654745797039165439, 0.03920185650866182814 ),
 ( 0.2389733096698791748, 1.000000000000000000 ),
 .UNSPECIFIED. ) 
 GEOMETRIC_REPRESENTATION_ITEM ( )  RATIONAL_B_SPLINE_SURFACE ( (
 ( 0.9863379792457529494, 0.9714151744119040588, 1.000000000000000000),
 ( 0.9868982363996166018, 0.9725873914152123323, 1.000000000000000000),
 ( 0.9870568516195763475, 0.9729192594806854721, 1.000000000000000000),
 ( 0.9864435726088423007, 0.9716361057017525171, 1.000000000000000000),
 ( 0.9856669209476500715, 0.9700111299622751204, 1.000000000000000000),
 ( 0.9831963891542060408, 0.9648420761527581879, 1.000000000000000000),
 ( 0.9815057839369669690, 0.9613048501345585750, 1.000000000000000000),
 ( 0.9773970105179623502, 0.9527081298048269975, 1.000000000000000000),
 ( 0.9749831541131945833, 0.9476576569965825536, 1.000000000000000000),
 ( 0.9723126921700375735, 0.9420702925606835310, 1.000000000000000000) ) ) 
 REPRESENTATION_ITEM ( '' )  SURFACE ( )  );
#22318=ORIENTED_EDGE ( 'NONE', *, *, #13136, .T. ) ;
#22320=CARTESIAN_POINT ( 'NONE',  ( -21.32594275109384085, 27.02633437841200603, 58.42208514511725781 ) ) ;
#22324=DIRECTION ( 'NONE',  ( -0.000000000000000000, -0.000000000000000000, 1.000000000000000000 ) ) ;
#22326=VERTEX_POINT ( 'NONE', #4616 ) ;
#22328=CARTESIAN_POINT ( 'NONE',  ( -7.313763316233817591, 40.00000000000000000, -52.68151668814096666 ) ) ;
#22329=DIRECTION ( 'NONE',  ( -0.000000000000000000, -0.000000000000000000, -1.000000000000000000 ) ) ;
#22331=EDGE_CURVE ( 'NONE', #16050, #19216, #13178, .T. ) ;
#22333=CARTESIAN_POINT ( 'NONE',  ( 42.50000000000000711, -5.000000000000000000, -41.00000000000000000 ) ) ;
#22334=VERTEX_POINT ( 'NONE', #724 ) ;
#22335=DIRECTION ( 'NONE',  ( -0.000000000000000000, -1.000000000000000000, -0.000000000000000000 ) ) ;
#22337=DIRECTION ( 'NONE',  ( 0.000000000000000000, -1.000000000000000000, 0.000000000000000000 ) ) ;
#22338=CARTESIAN_POINT ( 'NONE',  ( -5.833333333333328596, 33.81926995981417861, 40.61164310337068173 ) ) ;
#22339=EDGE_CURVE ( 'NONE', #18643, #20516, #7706, .T. ) ;
#22342=CARTESIAN_POINT ( 'NONE',  ( -9.079900094432140634, 0.2952490899071177899, 53.92155887445841955 ) ) ;
#22348=CARTESIAN_POINT ( 'NONE',  ( -19.39432138270236550, 15.03492235294285884, -60.47577240662248954 ) ) ;
#22350=CARTESIAN_POINT ( 'NONE',  ( -13.71171267331838273, 34.59605702017515938, 56.12298047978917026 ) ) ;
#22351=ADVANCED_FACE ( 'NONE', ( #20195 ), #3621, .F. ) ;
#22354=DIRECTION ( 'NONE',  ( 0.000000000000000000, 0.000000000000000000, 1.000000000000000000 ) ) ;
#22356=DIRECTION ( 'NONE',  ( -0.4166911066143264564, 0.000000000000000000, -0.9090481404571091328 ) ) ;
#22358=AXIS2_PLACEMENT_3D ( 'NONE', #9909, #16793, #1197 ) ;
#22361=CARTESIAN_POINT ( 'NONE',  ( 1.072795092646390724, 5.000000000000002665, 38.73397172404480671 ) ) ;
#22362=EDGE_CURVE ( 'NONE', #17743, #18756, #15638, .T. ) ;
#22363=EDGE_CURVE ( 'NONE', #8737, #8568, #7991, .T. ) ;
#22368=ORIENTED_EDGE ( 'NONE', *, *, #14617, .T. ) ;
#22369=CARTESIAN_POINT ( 'NONE',  ( 34.99999999999980815, 40.00000000000000711, 54.99999999999922551 ) ) ;
#22372=FACE_OUTER_BOUND ( 'NONE', #264, .T. ) ;
#22373=CARTESIAN_POINT ( 'NONE',  ( 18.11182660255252230, 11.48022137427003564, 60.14030069439205306 ) ) ;
#22374=DIRECTION ( 'NONE',  ( -0.000000000000000000, -1.000000000000000000, -0.000000000000000000 ) ) ;
#22377=DIRECTION ( 'NONE',  ( -0.000000000000000000, -0.000000000000000000, -1.000000000000000000 ) ) ;
#22378=ORIENTED_EDGE ( 'NONE', *, *, #3068, .T. ) ;
#22379=CARTESIAN_POINT ( 'NONE',  ( -11.86180952234344588, 38.99999999999292299, 55.35904751185378103 ) ) ;
#22380=CARTESIAN_POINT ( 'NONE',  ( -35.00000000000000000, 38.99999999999999289, -59.99999999999998579 ) ) ;
#22381=LINE ( 'NONE', #6670, #2379 ) ;
#22384=CARTESIAN_POINT ( 'NONE',  ( -8.118562887736894496, 39.55762400984859539, -53.90122742181765858 ) ) ;
#22387=CARTESIAN_POINT ( 'NONE',  ( -13.56354382738803466, 2.142135623730931471, 56.03997097393687454 ) ) ;
#22388=ORIENTED_EDGE ( 'NONE', *, *, #22363, .F. ) ;
#22390=CARTESIAN_POINT ( 'NONE',  ( 35.00000000000000711, 40.00000000000000000, 60.00000000000000711 ) ) ;
#22392=CARTESIAN_POINT ( 'NONE',  ( 19.88294660283887794, 17.66261523022804880, -60.59423886784173163 ) ) ;
#22393=ORIENTED_EDGE ( 'NONE', *, *, #7647, .T. ) ;
#22394=EDGE_CURVE ( 'NONE', #14544, #3949, #18924, .T. ) ;
#22395=EDGE_CURVE ( 'NONE', #15748, #22593, #1049, .T. ) ;
#22396=ORIENTED_EDGE ( 'NONE', *, *, #4435, .F. ) ;
#22397=VERTEX_POINT ( 'NONE', #19153 ) ;
#22399=CARTESIAN_POINT ( 'NONE',  ( 6.696867368503558448E-15, 39.00000000000000711, 48.73397172404481381 ) ) ;
#22401=AXIS2_PLACEMENT_3D ( 'NONE', #22369, #10079, #17074 ) ;
#22403=EDGE_CURVE ( 'NONE', #14085, #6835, #1416, .T. ) ;
#22404=EDGE_LOOP ( 'NONE', ( #313, #10077, #19999, #15503 ) ) ;
#22406=LINE ( 'NONE', #16667, #770 ) ;
#22412=CARTESIAN_POINT ( 'NONE',  ( -1.952222864267822100, 39.97720380408218688, 50.19196443857154577 ) ) ;
#22415=CIRCLE ( 'NONE', #11422, 2.499999999999995115 ) ;
#22416=CARTESIAN_POINT ( 'NONE',  ( -14.69988787053504709, 16.91499873015103006, 45.69379240540681053 ) ) ;
#22423=FACE_OUTER_BOUND ( 'NONE', #1840, .T. ) ;
#22425=CARTESIAN_POINT ( 'NONE',  ( -12.24744603030441148, 40.00000000000000000, 54.43639671998950291 ) ) ;
#22429=DIRECTION ( 'NONE',  ( 0.000000000000000000, -1.000000000000000000, 0.000000000000000000 ) ) ;
#22430=CARTESIAN_POINT ( 'NONE',  ( -7.248955618538786894, 40.00000000000000711, -52.65401628672144341 ) ) ;
#22431=CARTESIAN_POINT ( 'NONE',  ( 35.00000000000000711, 38.99999999999999289, 60.00000000000000711 ) ) ;
#22432=DIRECTION ( 'NONE',  ( 0.000000000000000000, 0.000000000000000000, -1.000000000000000000 ) ) ;
#22436=CARTESIAN_POINT ( 'NONE',  ( -10.77132920892044154, 39.17511451495860797, 54.93228420925925093 ) ) ;
#22442=DIRECTION ( 'NONE',  ( -0.000000000000000000, 1.000000000000000000, -0.000000000000000000 ) ) ;
#22449=CARTESIAN_POINT ( 'NONE',  ( -1.533556059876706179, -4.618461881322652118, 46.62226723458652344 ) ) ;
#22450=EDGE_CURVE ( 'NONE', #454, #4439, #21172, .T. ) ;
#22457=ADVANCED_FACE ( 'NONE', ( #12046 ), #11808, .F. ) ;
#22458=CARTESIAN_POINT ( 'NONE',  ( -18.96886095803721517, 26.35434275172291407, -60.36758075326453366 ) ) ;
#22459=CARTESIAN_POINT ( 'NONE',  ( -42.50000000000000711, -5.000000000000000000, -47.50000000000000000 ) ) ;
#22460=CARTESIAN_POINT ( 'NONE',  ( -15.90155957501130146, 35.87083899979363366, 56.88316157031724174 ) ) ;
#22462=CARTESIAN_POINT ( 'NONE',  ( 5.833333333333338366, 33.81926995981415729, 40.61164310337067462 ) ) ;
#22464=AXIS2_PLACEMENT_3D ( 'NONE', #13723, #15338, #1257 ) ;
#22472=CARTESIAN_POINT ( 'NONE',  ( -34.99999999999999289, 39.00000000000000711, -49.99999999999997158 ) ) ;
#22473=CONICAL_SURFACE ( 'NONE', #10728, 17.00000000000001421, 0.7853981633974603804 ) ;
#22474=EDGE_LOOP ( 'NONE', ( #17453, #16074, #4666, #16110 ) ) ;
#22475=AXIS2_PLACEMENT_3D ( 'NONE', #21515, #16348, #658 ) ;
#22478=AXIS2_PLACEMENT_3D ( 'NONE', #5512, #14664, #7234 ) ;
#22484=DIRECTION ( 'NONE',  ( -1.000000000000000000, 0.000000000000000000, 0.000000000000000000 ) ) ;
#22485=ORIENTED_EDGE ( 'NONE', *, *, #3026, .T. ) ;
#22492=CARTESIAN_POINT ( 'NONE',  ( 8.555717054908910768, 39.50215801961479656, 54.09939909776313272 ) ) ;
#22493=ORIENTED_EDGE ( 'NONE', *, *, #2125, .T. ) ;
#22494=CARTESIAN_POINT ( 'NONE',  ( -5.400043222043034774, 39.81718168819095638, -52.45350590964093840 ) ) ;
#22497=CARTESIAN_POINT ( 'NONE',  ( -22.34927643452058632, 22.00360349561975326, 58.65118246389018708 ) ) ;
#22501=EDGE_CURVE ( 'NONE', #22194, #13976, #16967, .T. ) ;
#22502=DIRECTION ( 'NONE',  ( -0.000000000000000000, -1.000000000000000000, -0.000000000000000000 ) ) ;
#22504=CARTESIAN_POINT ( 'NONE',  ( 11.68090480754628402, 3.765577839755378076, -57.90797000640140624 ) ) ;
#22506=VERTEX_POINT ( 'NONE', #15799 ) ;
#22507=EDGE_LOOP ( 'NONE', ( #16199, #2997, #7187, #18582 ) ) ;
#22508=EDGE_CURVE ( 'NONE', #19216, #19994, #4350, .T. ) ;
#22509=CONICAL_SURFACE ( 'NONE', #16272, 8.999999999999973355, 0.7853981633974657095 ) ;
#22510=VERTEX_POINT ( 'NONE', #3572 ) ;
#22511=FACE_OUTER_BOUND ( 'NONE', #6120, .T. ) ;
#22515=CARTESIAN_POINT ( 'NONE',  ( 11.86180952233169705, 39.00000000000000000, 55.35904751184887118 ) ) ;
#22516=CARTESIAN_POINT ( 'NONE',  ( 6.488138469136647934, 39.99999999999999289, -52.32258420267954335 ) ) ;
#22517=EDGE_LOOP ( 'NONE', ( #5608, #5203, #12496, #3655 ) ) ;
#22519=LINE ( 'NONE', #5107, #19313 ) ;
#22520=ORIENTED_EDGE ( 'NONE', *, *, #4252, .F. ) ;
#22521=CARTESIAN_POINT ( 'NONE',  ( -5.510194049583325260, 0.6966826613253894740, 52.42111735158517405 ) ) ;
#22522=EDGE_CURVE ( 'NONE', #14603, #5777, #14302, .T. ) ;
#22523=CARTESIAN_POINT ( 'NONE',  ( 4.986731981817641213, 34.15484146257775677, 40.05110651909060238 ) ) ;
#22524=ORIENTED_EDGE ( 'NONE', *, *, #6949, .F. ) ;
#22525=CARTESIAN_POINT ( 'NONE',  ( 7.938322399564428089, 38.36220367130324860, -56.16250688144687331 ) ) ;
#22527=AXIS2_PLACEMENT_3D ( 'NONE', #4685, #18540, #6283 ) ;
#22538=ORIENTED_EDGE ( 'NONE', *, *, #6446, .T. ) ;
#22544=DIRECTION ( 'NONE',  ( 1.049727191138617217E-16, 0.5150380749100562650, -0.8571673007021111124 ) ) ;
#22546=CARTESIAN_POINT ( 'NONE',  ( 4.589694779437865968, 39.86882943453918671, 51.95767925715862390 ) ) ;
#22547=VECTOR ( 'NONE', #13812, 1000.000000000000000 ) ;
#22548=EDGE_LOOP ( 'NONE', ( #11221, #11095 ) ) ;
#22550=DIRECTION ( 'NONE',  ( -1.000000000000000000, 0.000000000000000000, 0.000000000000000000 ) ) ;
#22552=CARTESIAN_POINT ( 'NONE',  ( 9.952189117650780403, 40.00000000000000000, -53.64426396172070355 ) ) ;
#22557=CARTESIAN_POINT ( 'NONE',  ( -17.90966157241563650, 28.91510314404815318, 60.08313820791177307 ) ) ;
#22559=CONICAL_SURFACE ( 'NONE', #12281, 2.099999999999990763, 1.029744258676652091 ) ;
#22563=ADVANCED_FACE ( 'NONE', ( #9056 ), #9838, .F. ) ;
#22569=ORIENTED_EDGE ( 'NONE', *, *, #2211, .F. ) ;
#22570=CARTESIAN_POINT ( 'NONE',  ( 4.026578693505867612, -4.679980696183926980, -48.24134193084080380 ) ) ;
#22573=AXIS2_PLACEMENT_3D ( 'NONE', #22207, #19101, #15412 ) ;
#22574=AXIS2_PLACEMENT_3D ( 'NONE', #8837, #13870, #10431 ) ;
#22575=ORIENTED_EDGE ( 'NONE', *, *, #15313, .T. ) ;
#22578=DIRECTION ( 'NONE',  ( 0.000000000000000000, 0.000000000000000000, 1.000000000000000000 ) ) ;
#22580=CARTESIAN_POINT ( 'NONE',  ( -19.23106185100149901, 25.51013774189691929, -60.43438466297349976 ) ) ;
#22581=DIRECTION ( 'NONE',  ( 0.000000000000000000, -0.5150380749100547106, -0.8571673007021120005 ) ) ;
#22583=VERTEX_POINT ( 'NONE', #12584 ) ;
#22584=DIRECTION ( 'NONE',  ( 0.000000000000000000, 1.000000000000000000, 0.000000000000000000 ) ) ;
#22585=DIRECTION ( 'NONE',  ( -1.000000000000000000, 0.000000000000000000, 0.000000000000000000 ) ) ;
#22586=CARTESIAN_POINT ( 'NONE',  ( -34.99999999999980815, 26.00000000000000355, 54.99999999999922551 ) ) ;
#22587=FACE_OUTER_BOUND ( 'NONE', #9934, .T. ) ;
#22593=VERTEX_POINT ( 'NONE', #19383 ) ;
#22599=CARTESIAN_POINT ( 'NONE',  ( -0.05567163768954545844, -4.650449146058876160, 45.38800358221619291 ) ) ;
#22602=DIRECTION ( 'NONE',  ( -0.000000000000000000, -0.000000000000000000, 1.000000000000000000 ) ) ;
#22609=AXIS2_PLACEMENT_3D ( 'NONE', #12904, #16584, #19810 ) ;
#22610=DIRECTION ( 'NONE',  ( 0.000000000000000000, 1.000000000000000000, 0.000000000000000000 ) ) ;
#22611=CARTESIAN_POINT ( 'NONE',  ( 6.696867368503558448E-15, 40.00000000000000000, 38.73397172404480671 ) ) ;
#22612=CARTESIAN_POINT ( 'NONE',  ( 7.902600813477331343, 39.58333018208552545, 53.79900148939188398 ) ) ;
#22613=CARTESIAN_POINT ( 'NONE',  ( 14.99999999999998934, 20.38555233723673155, -45.82575694955836809 ) ) ;
#22616=CARTESIAN_POINT ( 'NONE',  ( -22.27968669415840708, 17.44229586407519506, 58.63614535158255592 ) ) ;
#22619=EDGE_CURVE ( 'NONE', #21644, #3949, #10922, .T. ) ;
#22620=CIRCLE ( 'NONE', #6151, 2.524999999999999467 ) ;
#22621=CIRCLE ( 'NONE', #16372, 57.07106781186551103 ) ;
#22622=DIRECTION ( 'NONE',  ( -1.000000000000000000, 0.000000000000000000, 0.000000000000000000 ) ) ;
#22625=CARTESIAN_POINT ( 'NONE',  ( 42.50000000000000711, -9.600000000000001421, 47.50000000000000711 ) ) ;
#22627=EDGE_CURVE ( 'NONE', #1608, #675, #5848, .T. ) ;
#22632=( NAMED_UNIT ( * ) PLANE_ANGLE_UNIT ( ) SI_UNIT ( $, .RADIAN. ) );
#22636=CYLINDRICAL_SURFACE ( 'NONE', #9173, 2.099999999999997868 ) ;
#22637=CARTESIAN_POINT ( 'NONE',  ( 0.9873823069974712041, 39.99999999999999289, 49.36449633666812531 ) ) ;
#22641=CARTESIAN_POINT ( 'NONE',  ( 35.00000000000058265, 28.00000000000000000, -55.00000000000076028 ) ) ;
#22642=VERTEX_POINT ( 'NONE', #19725 ) ;
#22644=CIRCLE ( 'NONE', #2129, 2.099999999999997868 ) ;
#22645=ORIENTED_EDGE ( 'NONE', *, *, #21648, .T. ) ;
#22647=VERTEX_POINT ( 'NONE', #14539 ) ;
#22648=CARTESIAN_POINT ( 'NONE',  ( 8.234900601806485199, 38.24530923897635404, -54.56726664451450404 ) ) ;
#22649=CIRCLE ( 'NONE', #5414, 2.000000000000000000 ) ;
#22651=CARTESIAN_POINT ( 'NONE',  ( 7.776554266669417956E-15, -4.648749848372173865, -45.43309249825056639 ) ) ;
#22653=CARTESIAN_POINT ( 'NONE',  ( -1.109399418554577021, 39.99267480748693515, 49.57771599688018682 ) ) ;
#22657=DIRECTION ( 'NONE',  ( -0.000000000000000000, -0.000000000000000000, 1.000000000000000000 ) ) ;
#22658=EDGE_CURVE ( 'NONE', #15733, #14756, #18261, .T. ) ;
#22659=EDGE_CURVE ( 'NONE', #22194, #11090, #19721, .T. ) ;
#22662=ORIENTED_EDGE ( 'NONE', *, *, #20660, .F. ) ;
#22663=EDGE_LOOP ( 'NONE', ( #12949, #1585 ) ) ;
#22667=CYLINDRICAL_SURFACE ( 'NONE', #4104, 9.000000000000003553 ) ;
#22669=ADVANCED_FACE ( 'NONE', ( #13979, #22511 ), #1301, .T. ) ;
#22671=CARTESIAN_POINT ( 'NONE',  ( 0.1621097943337942160, 39.99984846037706632, 48.85976281227350881 ) ) ;
#22675=DIRECTION ( 'NONE',  ( 1.000000000000000000, 0.000000000000000000, 0.000000000000000000 ) ) ;
#22677=CARTESIAN_POINT ( 'NONE',  ( -1.387778780781445518E-14, 20.00000000000000355, -102.0000000000000142 ) ) ;
#22689=ORIENTED_EDGE ( 'NONE', *, *, #10441, .T. ) ;
#22692=CARTESIAN_POINT ( 'NONE',  ( 12.24744603030438839, 40.00000000000000000, -54.43639671998947449 ) ) ;
#22693=ORIENTED_EDGE ( 'NONE', *, *, #10811, .T. ) ;
#22721=COLOUR_RGB('Sky Blue',0.24,0.69,0.87);
#22722=FILL_AREA_STYLE_COLOUR('',#22721);
#22723=FILL_AREA_STYLE('',(#22722));
#22724=SURFACE_STYLE_FILL_AREA(#22723);
#22725=SURFACE_SIDE_STYLE('',(#22724));
#22726=SURFACE_STYLE_USAGE(.BOTH.,#22725);
#22727=PRESENTATION_STYLE_ASSIGNMENT((#22726));
ENDSEC;
END-ISO-10303-21;
